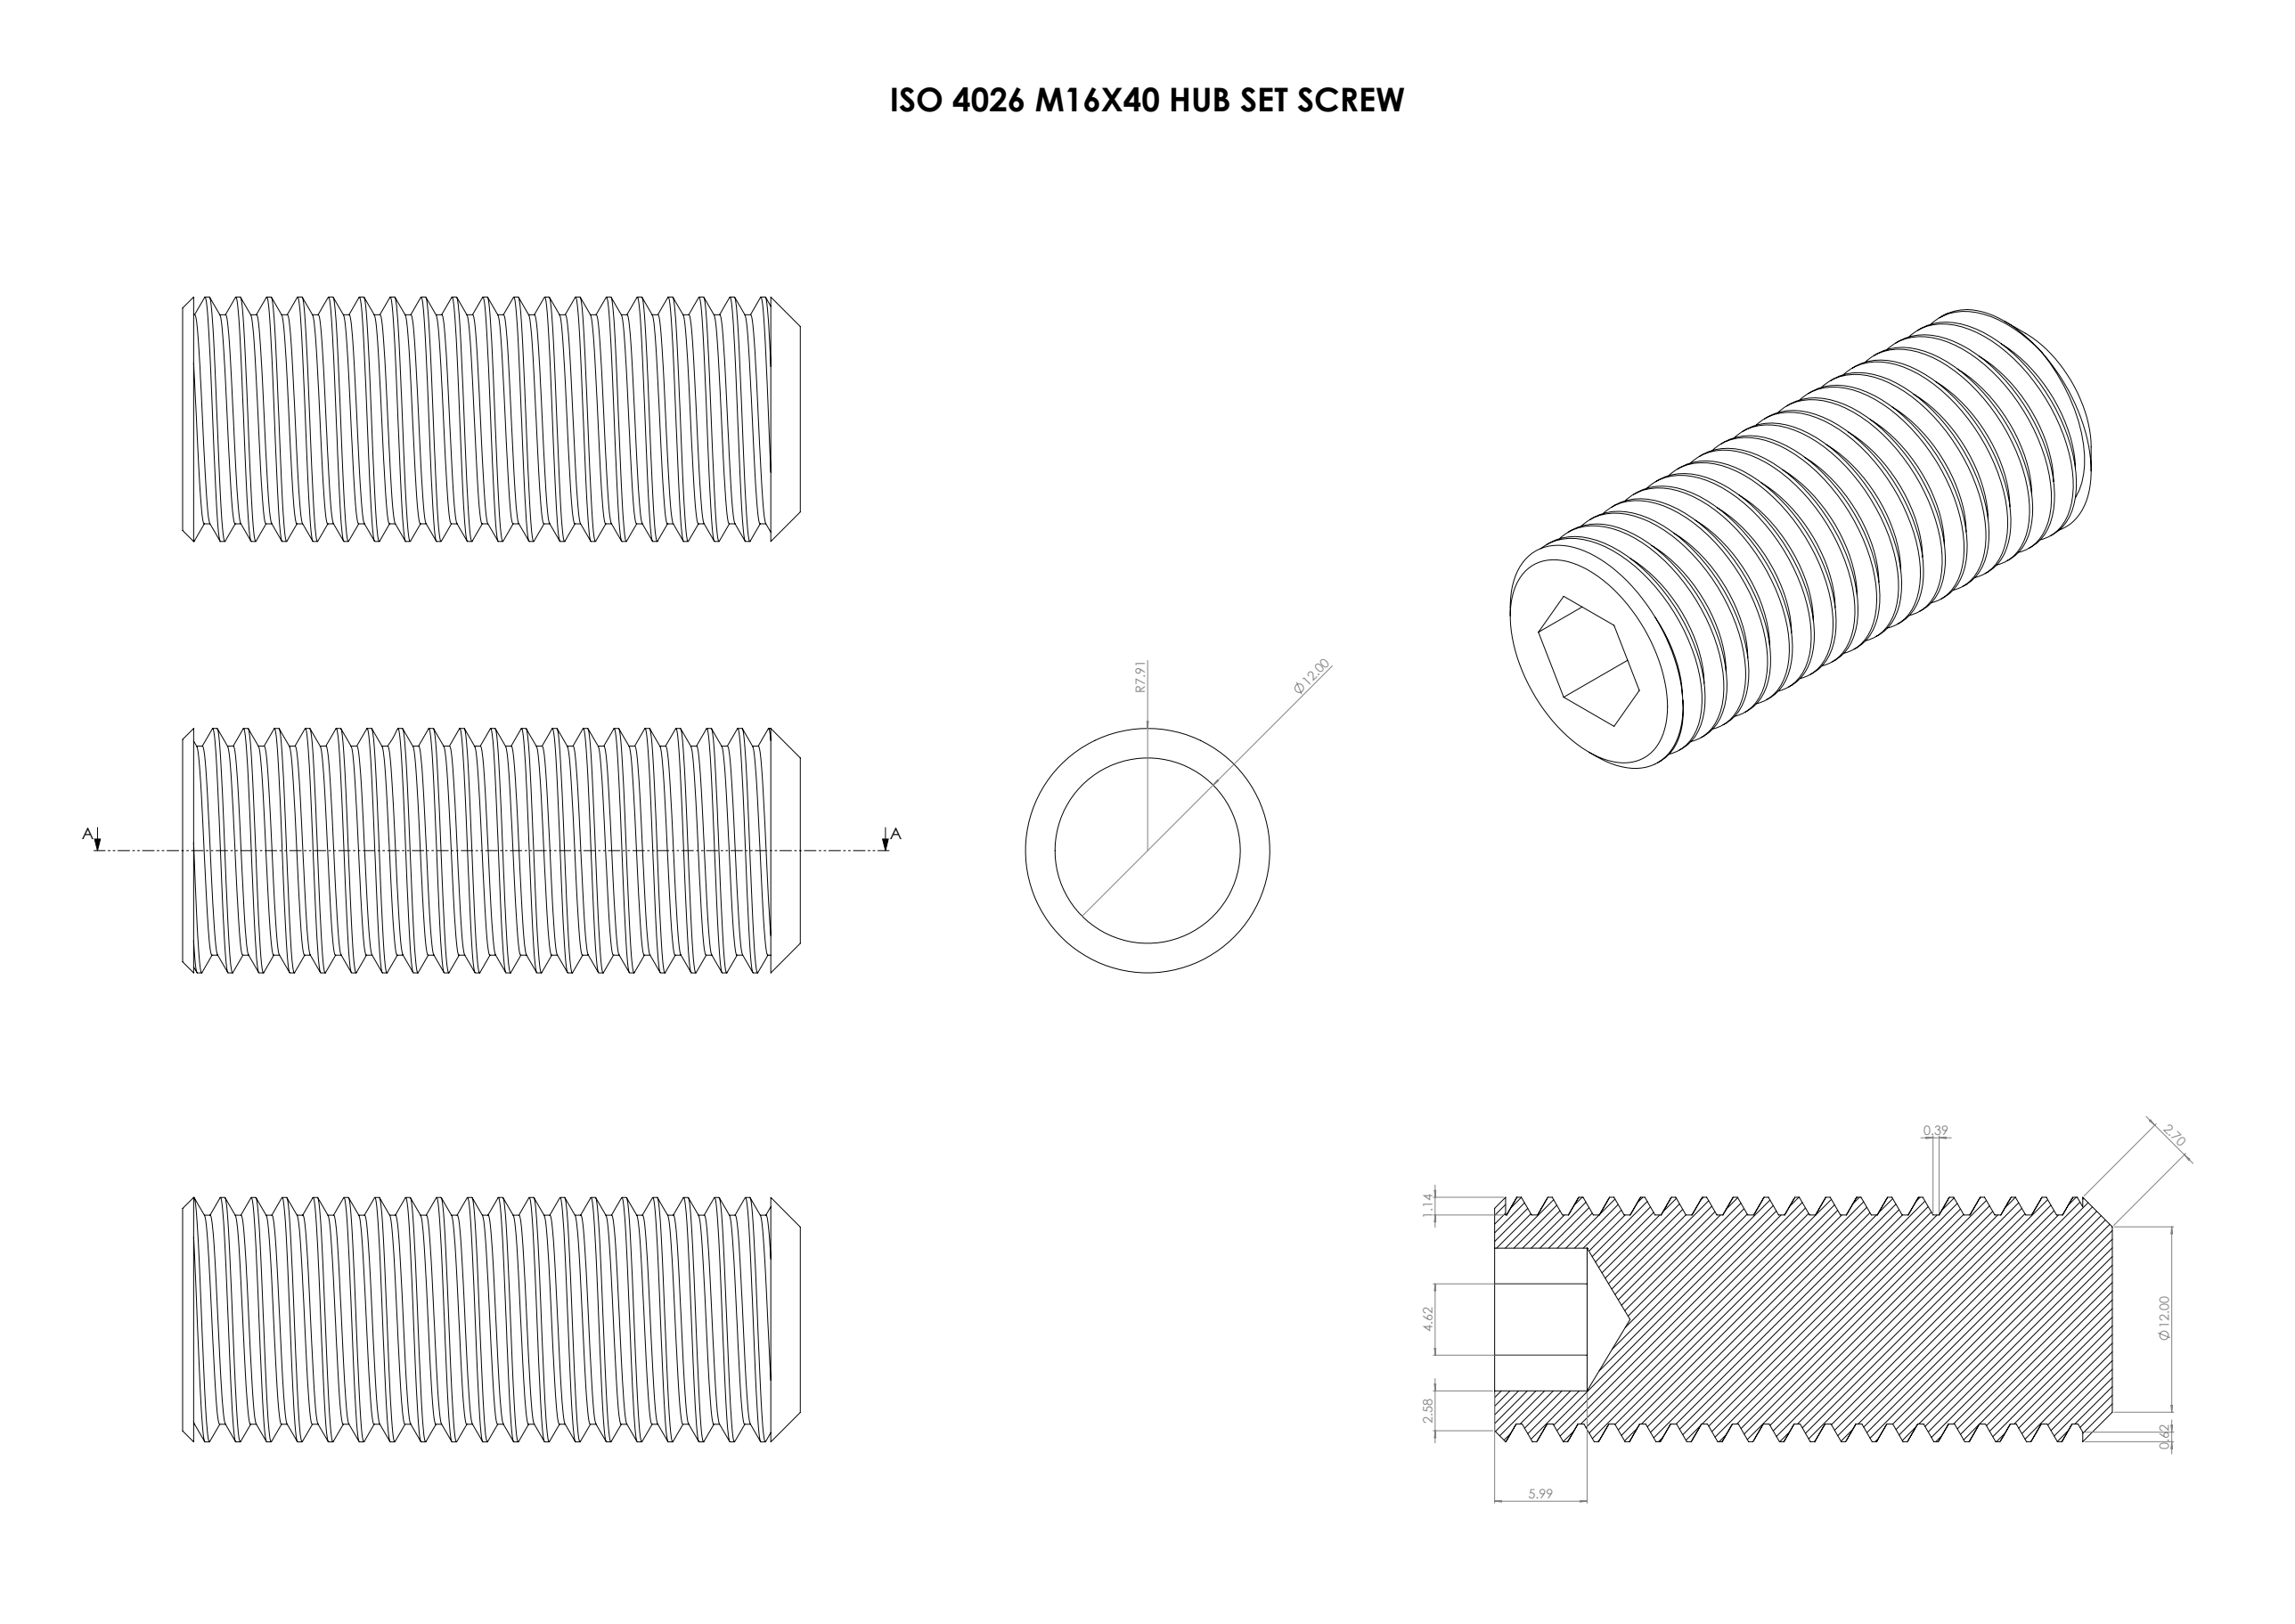
ISO-10303-21;
HEADER;
/* Generated by software containing ST-Developer
 * from STEP Tools, Inc. (www.steptools.com) 
 */

FILE_DESCRIPTION(
/* description */ (''),
/* implementation_level */ '2;1');

FILE_NAME(
/* name */ '14_ISO_4026_M16x40_Hub_Set_Screw.step',
/* time_stamp */ '2026-10-19T23:58:09-07:00',
/* author */ (''),
/* organization */ (''),
/* preprocessor_version */ 'ST-DEVELOPER v20.2',
/* originating_system */ 'Autodesk Translation Framework v15.15.0.0',
/* authorisation */ '');

FILE_SCHEMA (('AP203_CONFIGURATION_CONTROLLED_3D_DESIGN_OF_MECHANICAL_PARTS_AND_ASSEMBLIES_MIM_LF { 1 0 10303 203 3 1 4 }',
'AUTOMOTIVE_DESIGN { 1 0 10303 214 3 1 1 }','INTEGRATED_CNC_SCHEMA','MODEL_BASED_INTEGRATED_MANUFACTURING_SCHEMA',
'PROCESS_PLANNING_SCHEMA','AP242_MANAGED_MODEL_BASED_3D_ENGINEERING_MIM_LF { 1 0 10303 442 3 1 4 }'));
ENDSEC;

DATA;
#10=MECHANICAL_DESIGN_GEOMETRIC_PRESENTATION_REPRESENTATION('',(#416),#70757);
#241=(
BOUNDED_CURVE()
B_SPLINE_CURVE(2,(#59352,#59353,#59354),.UNSPECIFIED.,.F.,.F.)
B_SPLINE_CURVE_WITH_KNOTS((3,3),(0.,0.00348603246849772),.UNSPECIFIED.)
CURVE()
GEOMETRIC_REPRESENTATION_ITEM()
RATIONAL_B_SPLINE_CURVE((1.,1.00000655818292,1.))
REPRESENTATION_ITEM('')
);
#242=(
BOUNDED_CURVE()
B_SPLINE_CURVE(2,(#59356,#59357,#59358),.UNSPECIFIED.,.F.,.F.)
B_SPLINE_CURVE_WITH_KNOTS((3,3),(0.,0.0034860324684977),.UNSPECIFIED.)
CURVE()
GEOMETRIC_REPRESENTATION_ITEM()
RATIONAL_B_SPLINE_CURVE((1.,1.00000655824651,1.))
REPRESENTATION_ITEM('')
);
#243=(
BOUNDED_CURVE()
B_SPLINE_CURVE(2,(#59361,#59362,#59363),.UNSPECIFIED.,.F.,.F.)
B_SPLINE_CURVE_WITH_KNOTS((3,3),(0.,0.00348603246849777),.UNSPECIFIED.)
CURVE()
GEOMETRIC_REPRESENTATION_ITEM()
RATIONAL_B_SPLINE_CURVE((1.,1.00000655828125,1.))
REPRESENTATION_ITEM('')
);
#244=(
BOUNDED_CURVE()
B_SPLINE_CURVE(2,(#59365,#59366,#59367),.UNSPECIFIED.,.F.,.F.)
B_SPLINE_CURVE_WITH_KNOTS((3,3),(0.,0.00348603246849785),.UNSPECIFIED.)
CURVE()
GEOMETRIC_REPRESENTATION_ITEM()
RATIONAL_B_SPLINE_CURVE((1.,1.00000655858972,1.))
REPRESENTATION_ITEM('')
);
#245=(
BOUNDED_CURVE()
B_SPLINE_CURVE(2,(#59370,#59371,#59372),.UNSPECIFIED.,.F.,.F.)
B_SPLINE_CURVE_WITH_KNOTS((3,3),(0.,0.00348603246849743),.UNSPECIFIED.)
CURVE()
GEOMETRIC_REPRESENTATION_ITEM()
RATIONAL_B_SPLINE_CURVE((1.,1.00000655826316,1.))
REPRESENTATION_ITEM('')
);
#246=(
BOUNDED_CURVE()
B_SPLINE_CURVE(2,(#59374,#59375,#59376),.UNSPECIFIED.,.F.,.F.)
B_SPLINE_CURVE_WITH_KNOTS((3,3),(0.,0.00348603246849747),.UNSPECIFIED.)
CURVE()
GEOMETRIC_REPRESENTATION_ITEM()
RATIONAL_B_SPLINE_CURVE((1.,1.00000655837246,1.))
REPRESENTATION_ITEM('')
);
#247=(
BOUNDED_CURVE()
B_SPLINE_CURVE(2,(#59379,#59380,#59381),.UNSPECIFIED.,.F.,.F.)
B_SPLINE_CURVE_WITH_KNOTS((3,3),(0.,0.00348603246849727),.UNSPECIFIED.)
CURVE()
GEOMETRIC_REPRESENTATION_ITEM()
RATIONAL_B_SPLINE_CURVE((1.,1.00000655774933,1.))
REPRESENTATION_ITEM('')
);
#248=(
BOUNDED_CURVE()
B_SPLINE_CURVE(2,(#59383,#59384,#59385),.UNSPECIFIED.,.F.,.F.)
B_SPLINE_CURVE_WITH_KNOTS((3,3),(0.,0.00348603246849747),.UNSPECIFIED.)
CURVE()
GEOMETRIC_REPRESENTATION_ITEM()
RATIONAL_B_SPLINE_CURVE((1.,1.00000655778188,1.))
REPRESENTATION_ITEM('')
);
#249=(
BOUNDED_CURVE()
B_SPLINE_CURVE(2,(#59388,#59389,#59390),.UNSPECIFIED.,.F.,.F.)
B_SPLINE_CURVE_WITH_KNOTS((3,3),(0.,0.00348603246849769),.UNSPECIFIED.)
CURVE()
GEOMETRIC_REPRESENTATION_ITEM()
RATIONAL_B_SPLINE_CURVE((1.,1.00000655825998,1.))
REPRESENTATION_ITEM('')
);
#250=(
BOUNDED_CURVE()
B_SPLINE_CURVE(2,(#59392,#59393,#59394),.UNSPECIFIED.,.F.,.F.)
B_SPLINE_CURVE_WITH_KNOTS((3,3),(0.,0.00348603246849761),.UNSPECIFIED.)
CURVE()
GEOMETRIC_REPRESENTATION_ITEM()
RATIONAL_B_SPLINE_CURVE((1.,1.00000655838487,1.))
REPRESENTATION_ITEM('')
);
#251=(
BOUNDED_CURVE()
B_SPLINE_CURVE(2,(#59397,#59398,#59399),.UNSPECIFIED.,.F.,.F.)
B_SPLINE_CURVE_WITH_KNOTS((3,3),(0.,0.00348603246849764),.UNSPECIFIED.)
CURVE()
GEOMETRIC_REPRESENTATION_ITEM()
RATIONAL_B_SPLINE_CURVE((1.,1.00000655822052,1.))
REPRESENTATION_ITEM('')
);
#252=(
BOUNDED_CURVE()
B_SPLINE_CURVE(2,(#59401,#59402,#59403),.UNSPECIFIED.,.F.,.F.)
B_SPLINE_CURVE_WITH_KNOTS((3,3),(0.,0.00348603246849749),.UNSPECIFIED.)
CURVE()
GEOMETRIC_REPRESENTATION_ITEM()
RATIONAL_B_SPLINE_CURVE((1.,1.00000655832735,1.))
REPRESENTATION_ITEM('')
);
#278=B_SPLINE_SURFACE_WITH_KNOTS('',3,3,((#57157,#57158,#57159,#57160,#57161,
#57162,#57163,#57164,#57165,#57166,#57167,#57168,#57169,#57170,#57171,#57172,
#57173,#57174,#57175,#57176,#57177,#57178,#57179,#57180,#57181,#57182,#57183,
#57184,#57185,#57186,#57187,#57188,#57189,#57190,#57191,#57192,#57193,#57194,
#57195,#57196,#57197,#57198,#57199,#57200,#57201,#57202,#57203,#57204,#57205,
#57206,#57207,#57208,#57209,#57210,#57211,#57212,#57213,#57214,#57215,#57216,
#57217,#57218,#57219,#57220,#57221,#57222,#57223,#57224,#57225,#57226,#57227,
#57228,#57229,#57230,#57231,#57232,#57233,#57234,#57235,#57236,#57237,#57238,
#57239,#57240,#57241,#57242,#57243,#57244,#57245,#57246,#57247,#57248,#57249,
#57250,#57251,#57252,#57253,#57254,#57255,#57256,#57257,#57258,#57259,#57260,
#57261,#57262,#57263,#57264,#57265,#57266,#57267,#57268,#57269,#57270,#57271,
#57272,#57273,#57274,#57275,#57276,#57277,#57278,#57279,#57280,#57281,#57282,
#57283,#57284,#57285,#57286,#57287,#57288,#57289,#57290,#57291,#57292,#57293,
#57294,#57295,#57296,#57297,#57298,#57299,#57300,#57301,#57302,#57303,#57304,
#57305,#57306,#57307,#57308,#57309,#57310,#57311,#57312,#57313,#57314,#57315,
#57316,#57317,#57318,#57319,#57320,#57321,#57322,#57323,#57324,#57325,#57326,
#57327,#57328,#57329,#57330,#57331,#57332,#57333,#57334,#57335,#57336,#57337,
#57338,#57339,#57340,#57341,#57342,#57343,#57344,#57345,#57346,#57347,#57348,
#57349,#57350,#57351,#57352,#57353,#57354,#57355,#57356,#57357,#57358,#57359,
#57360,#57361,#57362,#57363,#57364,#57365,#57366,#57367,#57368,#57369,#57370,
#57371,#57372,#57373,#57374,#57375,#57376,#57377,#57378,#57379,#57380,#57381,
#57382,#57383,#57384,#57385,#57386,#57387,#57388,#57389,#57390,#57391,#57392,
#57393,#57394,#57395,#57396,#57397,#57398,#57399),(#57400,#57401,#57402,
#57403,#57404,#57405,#57406,#57407,#57408,#57409,#57410,#57411,#57412,#57413,
#57414,#57415,#57416,#57417,#57418,#57419,#57420,#57421,#57422,#57423,#57424,
#57425,#57426,#57427,#57428,#57429,#57430,#57431,#57432,#57433,#57434,#57435,
#57436,#57437,#57438,#57439,#57440,#57441,#57442,#57443,#57444,#57445,#57446,
#57447,#57448,#57449,#57450,#57451,#57452,#57453,#57454,#57455,#57456,#57457,
#57458,#57459,#57460,#57461,#57462,#57463,#57464,#57465,#57466,#57467,#57468,
#57469,#57470,#57471,#57472,#57473,#57474,#57475,#57476,#57477,#57478,#57479,
#57480,#57481,#57482,#57483,#57484,#57485,#57486,#57487,#57488,#57489,#57490,
#57491,#57492,#57493,#57494,#57495,#57496,#57497,#57498,#57499,#57500,#57501,
#57502,#57503,#57504,#57505,#57506,#57507,#57508,#57509,#57510,#57511,#57512,
#57513,#57514,#57515,#57516,#57517,#57518,#57519,#57520,#57521,#57522,#57523,
#57524,#57525,#57526,#57527,#57528,#57529,#57530,#57531,#57532,#57533,#57534,
#57535,#57536,#57537,#57538,#57539,#57540,#57541,#57542,#57543,#57544,#57545,
#57546,#57547,#57548,#57549,#57550,#57551,#57552,#57553,#57554,#57555,#57556,
#57557,#57558,#57559,#57560,#57561,#57562,#57563,#57564,#57565,#57566,#57567,
#57568,#57569,#57570,#57571,#57572,#57573,#57574,#57575,#57576,#57577,#57578,
#57579,#57580,#57581,#57582,#57583,#57584,#57585,#57586,#57587,#57588,#57589,
#57590,#57591,#57592,#57593,#57594,#57595,#57596,#57597,#57598,#57599,#57600,
#57601,#57602,#57603,#57604,#57605,#57606,#57607,#57608,#57609,#57610,#57611,
#57612,#57613,#57614,#57615,#57616,#57617,#57618,#57619,#57620,#57621,#57622,
#57623,#57624,#57625,#57626,#57627,#57628,#57629,#57630,#57631,#57632,#57633,
#57634,#57635,#57636,#57637,#57638,#57639,#57640,#57641,#57642),(#57643,
#57644,#57645,#57646,#57647,#57648,#57649,#57650,#57651,#57652,#57653,#57654,
#57655,#57656,#57657,#57658,#57659,#57660,#57661,#57662,#57663,#57664,#57665,
#57666,#57667,#57668,#57669,#57670,#57671,#57672,#57673,#57674,#57675,#57676,
#57677,#57678,#57679,#57680,#57681,#57682,#57683,#57684,#57685,#57686,#57687,
#57688,#57689,#57690,#57691,#57692,#57693,#57694,#57695,#57696,#57697,#57698,
#57699,#57700,#57701,#57702,#57703,#57704,#57705,#57706,#57707,#57708,#57709,
#57710,#57711,#57712,#57713,#57714,#57715,#57716,#57717,#57718,#57719,#57720,
#57721,#57722,#57723,#57724,#57725,#57726,#57727,#57728,#57729,#57730,#57731,
#57732,#57733,#57734,#57735,#57736,#57737,#57738,#57739,#57740,#57741,#57742,
#57743,#57744,#57745,#57746,#57747,#57748,#57749,#57750,#57751,#57752,#57753,
#57754,#57755,#57756,#57757,#57758,#57759,#57760,#57761,#57762,#57763,#57764,
#57765,#57766,#57767,#57768,#57769,#57770,#57771,#57772,#57773,#57774,#57775,
#57776,#57777,#57778,#57779,#57780,#57781,#57782,#57783,#57784,#57785,#57786,
#57787,#57788,#57789,#57790,#57791,#57792,#57793,#57794,#57795,#57796,#57797,
#57798,#57799,#57800,#57801,#57802,#57803,#57804,#57805,#57806,#57807,#57808,
#57809,#57810,#57811,#57812,#57813,#57814,#57815,#57816,#57817,#57818,#57819,
#57820,#57821,#57822,#57823,#57824,#57825,#57826,#57827,#57828,#57829,#57830,
#57831,#57832,#57833,#57834,#57835,#57836,#57837,#57838,#57839,#57840,#57841,
#57842,#57843,#57844,#57845,#57846,#57847,#57848,#57849,#57850,#57851,#57852,
#57853,#57854,#57855,#57856,#57857,#57858,#57859,#57860,#57861,#57862,#57863,
#57864,#57865,#57866,#57867,#57868,#57869,#57870,#57871,#57872,#57873,#57874,
#57875,#57876,#57877,#57878,#57879,#57880,#57881,#57882,#57883,#57884,#57885),
(#57886,#57887,#57888,#57889,#57890,#57891,#57892,#57893,#57894,#57895,
#57896,#57897,#57898,#57899,#57900,#57901,#57902,#57903,#57904,#57905,#57906,
#57907,#57908,#57909,#57910,#57911,#57912,#57913,#57914,#57915,#57916,#57917,
#57918,#57919,#57920,#57921,#57922,#57923,#57924,#57925,#57926,#57927,#57928,
#57929,#57930,#57931,#57932,#57933,#57934,#57935,#57936,#57937,#57938,#57939,
#57940,#57941,#57942,#57943,#57944,#57945,#57946,#57947,#57948,#57949,#57950,
#57951,#57952,#57953,#57954,#57955,#57956,#57957,#57958,#57959,#57960,#57961,
#57962,#57963,#57964,#57965,#57966,#57967,#57968,#57969,#57970,#57971,#57972,
#57973,#57974,#57975,#57976,#57977,#57978,#57979,#57980,#57981,#57982,#57983,
#57984,#57985,#57986,#57987,#57988,#57989,#57990,#57991,#57992,#57993,#57994,
#57995,#57996,#57997,#57998,#57999,#58000,#58001,#58002,#58003,#58004,#58005,
#58006,#58007,#58008,#58009,#58010,#58011,#58012,#58013,#58014,#58015,#58016,
#58017,#58018,#58019,#58020,#58021,#58022,#58023,#58024,#58025,#58026,#58027,
#58028,#58029,#58030,#58031,#58032,#58033,#58034,#58035,#58036,#58037,#58038,
#58039,#58040,#58041,#58042,#58043,#58044,#58045,#58046,#58047,#58048,#58049,
#58050,#58051,#58052,#58053,#58054,#58055,#58056,#58057,#58058,#58059,#58060,
#58061,#58062,#58063,#58064,#58065,#58066,#58067,#58068,#58069,#58070,#58071,
#58072,#58073,#58074,#58075,#58076,#58077,#58078,#58079,#58080,#58081,#58082,
#58083,#58084,#58085,#58086,#58087,#58088,#58089,#58090,#58091,#58092,#58093,
#58094,#58095,#58096,#58097,#58098,#58099,#58100,#58101,#58102,#58103,#58104,
#58105,#58106,#58107,#58108,#58109,#58110,#58111,#58112,#58113,#58114,#58115,
#58116,#58117,#58118,#58119,#58120,#58121,#58122,#58123,#58124,#58125,#58126,
#58127,#58128)),.UNSPECIFIED.,.F.,.F.,.F.,(4,4),(4,1,1,1,1,1,1,1,1,1,1,
1,1,1,1,1,1,1,1,1,1,1,1,1,1,1,1,1,1,1,1,1,1,1,1,1,1,1,1,1,1,1,1,1,1,1,1,
1,1,1,1,1,1,1,1,1,1,1,1,1,1,1,1,1,1,1,1,1,1,1,1,1,1,1,1,1,1,1,1,1,1,1,1,
1,1,1,1,1,1,1,1,1,1,1,1,1,1,1,1,1,1,1,1,1,1,1,1,1,1,1,1,1,1,1,1,1,1,1,1,
1,1,1,1,1,1,1,1,1,1,1,1,1,1,1,1,1,1,1,1,1,1,1,1,1,1,1,1,1,1,1,1,1,1,1,1,
1,1,1,1,1,1,1,1,1,1,1,1,1,1,1,1,1,1,1,1,1,1,1,1,1,1,1,1,1,1,1,1,1,1,1,1,
1,1,1,1,1,1,1,1,1,1,1,1,1,1,1,1,1,1,1,1,1,1,1,1,1,1,1,1,1,1,1,1,1,1,1,1,
1,1,1,1,1,1,1,1,1,1,1,1,1,4),(0.,0.132097741590586),(8.30112925462614,8.79905190745349,
9.29697456028084,9.79489721310818,10.2928198659355,10.7907425187629,11.2886651715902,
11.7865878244176,12.2845104772449,12.7824331300723,13.2803557828996,13.778278435727,
14.2762010885543,14.7741237413817,15.272046394209,15.7699690470363,16.2678916998637,
16.765814352691,17.2637370055184,17.7616596583457,18.2595823111731,18.7575049640004,
19.2554276168278,19.7533502696551,20.2512729224825,20.7491955753098,21.2471182281372,
21.7450408809645,22.2429635337919,22.7408861866192,23.2388088394466,23.7367314922739,
24.2346541451012,24.7325767979286,25.2304994507559,25.7284221035833,26.2263447564106,
26.724267409238,27.2221900620653,27.7201127148927,28.21803536772,28.7159580205474,
29.2138806733747,29.7118033262021,30.2097259790294,30.7076486318568,31.2055712846841,
31.7034939375114,32.2014165903388,32.6993392431661,33.1972618959935,33.6951845488208,
34.1931072016482,34.6910298544755,35.1889525073029,35.6868751601302,36.1847978129576,
36.6827204657849,37.1806431186123,37.6785657714396,38.176488424267,38.6744110770943,
39.1723337299217,39.670256382749,40.1681790355763,40.6661016884037,41.164024341231,
41.6619469940584,42.1598696468857,42.6577922997131,43.1557149525404,43.6536376053678,
44.1515602581951,44.6494829110225,45.1474055638498,45.6453282166772,46.1432508695045,
46.6411735223319,47.1390961751592,47.6370188279866,48.1349414808139,48.6328641336412,
49.1307867864686,49.6287094392959,50.1266320921233,50.6245547449506,51.122477397778,
51.6204000506053,52.1183227034327,52.61624535626,53.1141680090874,53.6120906619147,
54.1100133147421,54.6079359675694,55.1058586203968,55.6037812732241,56.1017039260515,
56.5996265788788,57.0975492317061,57.5954718845335,58.0933945373608,58.5913171901882,
59.0892398430155,59.5871624958429,60.0850851486702,60.5830078014976,61.0809304543249,
61.5788531071523,62.0767757599796,62.574698412807,63.0726210656343,63.5705437184617,
64.068466371289,64.5663890241163,65.0643116769437,65.562234329771,66.0601569825984,
66.5580796354257,67.0560022882531,67.5539249410804,68.0518475939078,68.5497702467351,
69.0476928995625,69.5456155523898,70.0435382052172,70.5414608580445,71.0393835108719,
71.5373061636992,72.0352288165266,72.5331514693539,73.0310741221813,73.5289967750086,
74.0269194278359,74.5248420806633,75.0227647334906,75.520687386318,76.0186100391453,
76.5165326919727,77.0144553448,77.5123779976274,78.0103006504547,78.5082233032821,
79.0061459561094,79.5040686089368,80.0019912617641,80.4999139145914,80.9978365674188,
81.4957592202462,81.9936818730735,82.4916045259008,82.9895271787282,83.4874498315555,
83.9853724843829,84.4832951372102,84.9812177900376,85.4791404428649,85.9770630956923,
86.4749857485196,86.972908401347,87.4708310541743,87.9687537070017,88.466676359829,
88.9645990126564,89.4625216654837,89.960444318311,90.4583669711384,90.9562896239657,
91.4542122767931,91.9521349296204,92.4500575824478,92.9479802352751,93.4459028881025,
93.9438255409298,94.4417481937572,94.9396708465845,95.4375934994119,95.9355161522392,
96.4334388050665,96.9313614578939,97.4292841107213,97.9272067635486,98.4251294163759,
98.9230520692033,99.4209747220306,99.918897374858,100.416820027685,100.914742680513,
101.41266533334,101.910587986167,102.408510638995,102.906433291822,103.404355944649,
103.902278597477,104.400201250304,104.898123903131,105.396046555959,105.893969208786,
106.391891861613,106.889814514441,107.387737167268,107.885659820096,108.383582472923,
108.88150512575,109.379427778578,109.877350431405,110.375273084232,110.87319573706,
111.371118389887,111.869041042714,112.366963695542,112.864886348369,113.362809001196,
113.860731654024,114.358654306851,114.856576959678,115.354499612506,115.852422265333,
116.35034491816,116.848267570988,117.346190223815,117.844112876642,118.34203552947,
118.839958182297,119.337880835125,119.835803487952,120.333726140779,120.831648793607,
121.329571446434,121.827494099261,122.325416752089,122.823339404916,123.321262057743,
123.819184710571,124.317107363398,124.815030016225,125.312952669053,125.81087532188,
126.308797974707,126.806720627535,127.304643280362,127.802565933189),
 .UNSPECIFIED.);
#279=B_SPLINE_SURFACE_WITH_KNOTS('',3,3,((#58334,#58335,#58336,#58337,#58338,
#58339,#58340,#58341,#58342,#58343,#58344,#58345,#58346,#58347,#58348,#58349,
#58350,#58351,#58352,#58353,#58354,#58355,#58356,#58357,#58358,#58359,#58360,
#58361,#58362,#58363,#58364,#58365,#58366,#58367,#58368,#58369,#58370,#58371,
#58372,#58373,#58374,#58375,#58376,#58377,#58378,#58379,#58380,#58381,#58382,
#58383,#58384,#58385,#58386,#58387,#58388,#58389,#58390,#58391,#58392,#58393,
#58394,#58395,#58396,#58397,#58398,#58399,#58400,#58401,#58402,#58403,#58404,
#58405,#58406,#58407,#58408,#58409,#58410,#58411,#58412,#58413,#58414,#58415,
#58416,#58417,#58418,#58419,#58420,#58421,#58422,#58423,#58424,#58425,#58426,
#58427,#58428,#58429,#58430,#58431,#58432,#58433,#58434,#58435,#58436,#58437,
#58438,#58439,#58440,#58441,#58442,#58443,#58444,#58445,#58446,#58447,#58448,
#58449,#58450,#58451,#58452,#58453,#58454,#58455,#58456,#58457,#58458,#58459,
#58460,#58461,#58462,#58463,#58464,#58465,#58466,#58467,#58468,#58469,#58470,
#58471,#58472,#58473,#58474,#58475,#58476,#58477,#58478,#58479,#58480,#58481,
#58482,#58483,#58484,#58485,#58486,#58487,#58488,#58489,#58490,#58491,#58492,
#58493,#58494,#58495,#58496,#58497,#58498,#58499,#58500,#58501,#58502,#58503,
#58504,#58505,#58506,#58507,#58508,#58509,#58510,#58511,#58512,#58513,#58514,
#58515,#58516,#58517,#58518,#58519,#58520,#58521,#58522,#58523,#58524,#58525,
#58526,#58527,#58528,#58529,#58530,#58531,#58532,#58533,#58534,#58535,#58536,
#58537,#58538,#58539,#58540,#58541,#58542,#58543,#58544,#58545,#58546,#58547,
#58548,#58549,#58550,#58551,#58552,#58553,#58554,#58555,#58556,#58557,#58558,
#58559,#58560,#58561,#58562,#58563,#58564,#58565,#58566,#58567,#58568,#58569,
#58570,#58571,#58572,#58573,#58574,#58575,#58576),(#58577,#58578,#58579,
#58580,#58581,#58582,#58583,#58584,#58585,#58586,#58587,#58588,#58589,#58590,
#58591,#58592,#58593,#58594,#58595,#58596,#58597,#58598,#58599,#58600,#58601,
#58602,#58603,#58604,#58605,#58606,#58607,#58608,#58609,#58610,#58611,#58612,
#58613,#58614,#58615,#58616,#58617,#58618,#58619,#58620,#58621,#58622,#58623,
#58624,#58625,#58626,#58627,#58628,#58629,#58630,#58631,#58632,#58633,#58634,
#58635,#58636,#58637,#58638,#58639,#58640,#58641,#58642,#58643,#58644,#58645,
#58646,#58647,#58648,#58649,#58650,#58651,#58652,#58653,#58654,#58655,#58656,
#58657,#58658,#58659,#58660,#58661,#58662,#58663,#58664,#58665,#58666,#58667,
#58668,#58669,#58670,#58671,#58672,#58673,#58674,#58675,#58676,#58677,#58678,
#58679,#58680,#58681,#58682,#58683,#58684,#58685,#58686,#58687,#58688,#58689,
#58690,#58691,#58692,#58693,#58694,#58695,#58696,#58697,#58698,#58699,#58700,
#58701,#58702,#58703,#58704,#58705,#58706,#58707,#58708,#58709,#58710,#58711,
#58712,#58713,#58714,#58715,#58716,#58717,#58718,#58719,#58720,#58721,#58722,
#58723,#58724,#58725,#58726,#58727,#58728,#58729,#58730,#58731,#58732,#58733,
#58734,#58735,#58736,#58737,#58738,#58739,#58740,#58741,#58742,#58743,#58744,
#58745,#58746,#58747,#58748,#58749,#58750,#58751,#58752,#58753,#58754,#58755,
#58756,#58757,#58758,#58759,#58760,#58761,#58762,#58763,#58764,#58765,#58766,
#58767,#58768,#58769,#58770,#58771,#58772,#58773,#58774,#58775,#58776,#58777,
#58778,#58779,#58780,#58781,#58782,#58783,#58784,#58785,#58786,#58787,#58788,
#58789,#58790,#58791,#58792,#58793,#58794,#58795,#58796,#58797,#58798,#58799,
#58800,#58801,#58802,#58803,#58804,#58805,#58806,#58807,#58808,#58809,#58810,
#58811,#58812,#58813,#58814,#58815,#58816,#58817,#58818,#58819),(#58820,
#58821,#58822,#58823,#58824,#58825,#58826,#58827,#58828,#58829,#58830,#58831,
#58832,#58833,#58834,#58835,#58836,#58837,#58838,#58839,#58840,#58841,#58842,
#58843,#58844,#58845,#58846,#58847,#58848,#58849,#58850,#58851,#58852,#58853,
#58854,#58855,#58856,#58857,#58858,#58859,#58860,#58861,#58862,#58863,#58864,
#58865,#58866,#58867,#58868,#58869,#58870,#58871,#58872,#58873,#58874,#58875,
#58876,#58877,#58878,#58879,#58880,#58881,#58882,#58883,#58884,#58885,#58886,
#58887,#58888,#58889,#58890,#58891,#58892,#58893,#58894,#58895,#58896,#58897,
#58898,#58899,#58900,#58901,#58902,#58903,#58904,#58905,#58906,#58907,#58908,
#58909,#58910,#58911,#58912,#58913,#58914,#58915,#58916,#58917,#58918,#58919,
#58920,#58921,#58922,#58923,#58924,#58925,#58926,#58927,#58928,#58929,#58930,
#58931,#58932,#58933,#58934,#58935,#58936,#58937,#58938,#58939,#58940,#58941,
#58942,#58943,#58944,#58945,#58946,#58947,#58948,#58949,#58950,#58951,#58952,
#58953,#58954,#58955,#58956,#58957,#58958,#58959,#58960,#58961,#58962,#58963,
#58964,#58965,#58966,#58967,#58968,#58969,#58970,#58971,#58972,#58973,#58974,
#58975,#58976,#58977,#58978,#58979,#58980,#58981,#58982,#58983,#58984,#58985,
#58986,#58987,#58988,#58989,#58990,#58991,#58992,#58993,#58994,#58995,#58996,
#58997,#58998,#58999,#59000,#59001,#59002,#59003,#59004,#59005,#59006,#59007,
#59008,#59009,#59010,#59011,#59012,#59013,#59014,#59015,#59016,#59017,#59018,
#59019,#59020,#59021,#59022,#59023,#59024,#59025,#59026,#59027,#59028,#59029,
#59030,#59031,#59032,#59033,#59034,#59035,#59036,#59037,#59038,#59039,#59040,
#59041,#59042,#59043,#59044,#59045,#59046,#59047,#59048,#59049,#59050,#59051,
#59052,#59053,#59054,#59055,#59056,#59057,#59058,#59059,#59060,#59061,#59062),
(#59063,#59064,#59065,#59066,#59067,#59068,#59069,#59070,#59071,#59072,
#59073,#59074,#59075,#59076,#59077,#59078,#59079,#59080,#59081,#59082,#59083,
#59084,#59085,#59086,#59087,#59088,#59089,#59090,#59091,#59092,#59093,#59094,
#59095,#59096,#59097,#59098,#59099,#59100,#59101,#59102,#59103,#59104,#59105,
#59106,#59107,#59108,#59109,#59110,#59111,#59112,#59113,#59114,#59115,#59116,
#59117,#59118,#59119,#59120,#59121,#59122,#59123,#59124,#59125,#59126,#59127,
#59128,#59129,#59130,#59131,#59132,#59133,#59134,#59135,#59136,#59137,#59138,
#59139,#59140,#59141,#59142,#59143,#59144,#59145,#59146,#59147,#59148,#59149,
#59150,#59151,#59152,#59153,#59154,#59155,#59156,#59157,#59158,#59159,#59160,
#59161,#59162,#59163,#59164,#59165,#59166,#59167,#59168,#59169,#59170,#59171,
#59172,#59173,#59174,#59175,#59176,#59177,#59178,#59179,#59180,#59181,#59182,
#59183,#59184,#59185,#59186,#59187,#59188,#59189,#59190,#59191,#59192,#59193,
#59194,#59195,#59196,#59197,#59198,#59199,#59200,#59201,#59202,#59203,#59204,
#59205,#59206,#59207,#59208,#59209,#59210,#59211,#59212,#59213,#59214,#59215,
#59216,#59217,#59218,#59219,#59220,#59221,#59222,#59223,#59224,#59225,#59226,
#59227,#59228,#59229,#59230,#59231,#59232,#59233,#59234,#59235,#59236,#59237,
#59238,#59239,#59240,#59241,#59242,#59243,#59244,#59245,#59246,#59247,#59248,
#59249,#59250,#59251,#59252,#59253,#59254,#59255,#59256,#59257,#59258,#59259,
#59260,#59261,#59262,#59263,#59264,#59265,#59266,#59267,#59268,#59269,#59270,
#59271,#59272,#59273,#59274,#59275,#59276,#59277,#59278,#59279,#59280,#59281,
#59282,#59283,#59284,#59285,#59286,#59287,#59288,#59289,#59290,#59291,#59292,
#59293,#59294,#59295,#59296,#59297,#59298,#59299,#59300,#59301,#59302,#59303,
#59304,#59305)),.UNSPECIFIED.,.F.,.F.,.F.,(4,4),(4,1,1,1,1,1,1,1,1,1,1,
1,1,1,1,1,1,1,1,1,1,1,1,1,1,1,1,1,1,1,1,1,1,1,1,1,1,1,1,1,1,1,1,1,1,1,1,
1,1,1,1,1,1,1,1,1,1,1,1,1,1,1,1,1,1,1,1,1,1,1,1,1,1,1,1,1,1,1,1,1,1,1,1,
1,1,1,1,1,1,1,1,1,1,1,1,1,1,1,1,1,1,1,1,1,1,1,1,1,1,1,1,1,1,1,1,1,1,1,1,
1,1,1,1,1,1,1,1,1,1,1,1,1,1,1,1,1,1,1,1,1,1,1,1,1,1,1,1,1,1,1,1,1,1,1,1,
1,1,1,1,1,1,1,1,1,1,1,1,1,1,1,1,1,1,1,1,1,1,1,1,1,1,1,1,1,1,1,1,1,1,1,1,
1,1,1,1,1,1,1,1,1,1,1,1,1,1,1,1,1,1,1,1,1,1,1,1,1,1,1,1,1,1,1,1,1,1,1,1,
1,1,1,1,1,1,1,1,1,1,1,1,1,4),(0.,0.132097741590586),(11.6150328478182,12.1129555006455,
12.6108781534729,13.1088008063002,13.6067234591276,14.1046461119549,14.6025687647823,
15.1004914176096,15.5984140704369,16.0963367232643,16.5942593760916,17.092182028919,
17.5901046817463,18.0880273345737,18.585949987401,19.0838726402284,19.5817952930557,
20.0797179458831,20.5776405987104,21.0755632515378,21.5734859043651,22.0714085571925,
22.5693312100198,23.0672538628472,23.5651765156745,24.0630991685018,24.5610218213292,
25.0589444741565,25.5568671269839,26.0547897798112,26.5527124326386,27.0506350854659,
27.5485577382933,28.0464803911206,28.544403043948,29.0423256967753,29.5402483496027,
30.03817100243,30.5360936552574,31.0340163080847,31.5319389609121,32.0298616137394,
32.5277842665667,33.0257069193941,33.5236295722214,34.0215522250488,34.5194748778761,
35.0173975307035,35.5153201835308,36.0132428363582,36.5111654891855,37.0090881420129,
37.5070107948402,38.0049334476676,38.5028561004949,39.0007787533223,39.4987014061496,
39.9966240589769,40.4945467118043,40.9924693646316,41.490392017459,41.9883146702863,
42.4862373231137,42.984159975941,43.4820826287684,43.9800052815957,44.4779279344231,
44.9758505872504,45.4737732400778,45.9716958929051,46.4696185457325,46.9675411985598,
47.4654638513871,47.9633865042145,48.4613091570418,48.9592318098692,49.4571544626965,
49.9550771155239,50.4529997683512,50.9509224211786,51.4488450740059,51.9467677268333,
52.4446903796606,52.942613032488,53.4405356853153,53.9384583381427,54.43638099097,
54.9343036437973,55.4322262966247,55.930148949452,56.4280716022794,56.9259942551067,
57.4239169079341,57.9218395607614,58.4197622135888,58.9176848664161,59.4156075192435,
59.9135301720708,60.4114528248982,60.9093754777255,61.4072981305529,61.9052207833802,
62.4031434362076,62.9010660890349,63.3989887418622,63.8969113946896,64.3948340475169,
64.8927567003443,65.3906793531716,65.888602005999,66.3865246588263,66.8844473116537,
67.382369964481,67.8802926173084,68.3782152701357,68.8761379229631,69.3740605757904,
69.8719832286178,70.3699058814451,70.8678285342725,71.3657511870998,71.8636738399271,
72.3615964927545,72.8595191455818,73.3574417984092,73.8553644512365,74.3532871040639,
74.8512097568912,75.3491324097186,75.8470550625459,76.3449777153733,76.8429003682006,
77.340823021028,77.8387456738553,78.3366683266827,78.83459097951,79.3325136323374,
79.8304362851647,80.328358937992,80.8262815908194,81.3242042436467,81.8221268964741,
82.3200495493014,82.8179722021288,83.3158948549561,83.8138175077835,84.3117401606108,
84.8096628134382,85.3075854662655,85.8055081190928,86.3034307719202,86.8013534247476,
87.2992760775749,87.7971987304022,88.2951213832296,88.7930440360569,89.2909666888843,
89.7888893417116,90.286811994539,90.7847346473663,91.2826573001937,91.780579953021,
92.2785026058484,92.7764252586757,93.2743479115031,93.7722705643304,94.2701932171578,
94.7681158699851,95.2660385228125,95.7639611756398,96.2618838284671,96.7598064812945,
97.2577291341218,97.7556517869492,98.2535744397765,98.7514970926039,99.2494197454312,
99.7473423982586,100.245265051086,100.743187703913,101.241110356741,101.739033009568,
102.236955662395,102.734878315223,103.23280096805,103.730723620877,104.228646273705,
104.726568926532,105.224491579359,105.722414232187,106.220336885014,106.718259537841,
107.216182190669,107.714104843496,108.212027496323,108.709950149151,109.207872801978,
109.705795454805,110.203718107633,110.70164076046,111.199563413288,111.697486066115,
112.195408718942,112.69333137177,113.191254024597,113.689176677424,114.187099330252,
114.685021983079,115.182944635906,115.680867288734,116.178789941561,116.676712594388,
117.174635247216,117.672557900043,118.17048055287,118.668403205698,119.166325858525,
119.664248511352,120.16217116418,120.660093817007,121.158016469834,121.655939122662,
122.153861775489,122.651784428317,123.149707081144,123.647629733971,124.145552386799,
124.643475039626,125.141397692453,125.639320345281,126.137242998108,126.635165650935,
127.133088303763,127.63101095659,128.128933609417,128.626856262245,129.124778915072,
129.622701567899,130.120624220727,130.618546873554,131.116469526381),
 .UNSPECIFIED.);
#386=SHAPE_REPRESENTATION_RELATIONSHIP('SRR','None',#70827,#401);
#401=ADVANCED_BREP_SHAPE_REPRESENTATION('',(#476),#70751);
#416=STYLED_ITEM('',(#71054),#476);
#476=MANIFOLD_SOLID_BREP('Set screw',#26881);
#683=CYLINDRICAL_SURFACE('',#27690,0.7911);
#684=CYLINDRICAL_SURFACE('',#27692,0.7911);
#685=CYLINDRICAL_SURFACE('',#27693,0.7911);
#686=CYLINDRICAL_SURFACE('',#27694,0.7911);
#687=CYLINDRICAL_SURFACE('',#27695,0.7911);
#688=CYLINDRICAL_SURFACE('',#27696,0.7911);
#689=CYLINDRICAL_SURFACE('',#27697,0.7911);
#690=CYLINDRICAL_SURFACE('',#27698,0.7911);
#691=CYLINDRICAL_SURFACE('',#27699,0.7911);
#692=CYLINDRICAL_SURFACE('',#27700,0.7911);
#693=CYLINDRICAL_SURFACE('',#27701,0.7911);
#694=CYLINDRICAL_SURFACE('',#27702,0.7911);
#695=CYLINDRICAL_SURFACE('',#27703,0.7911);
#696=CYLINDRICAL_SURFACE('',#27704,0.7911);
#697=CYLINDRICAL_SURFACE('',#27705,0.7911);
#698=CYLINDRICAL_SURFACE('',#27706,0.7911);
#699=CYLINDRICAL_SURFACE('',#27707,0.7911);
#700=CYLINDRICAL_SURFACE('',#27708,0.7911);
#701=CYLINDRICAL_SURFACE('',#27709,0.7911);
#702=CYLINDRICAL_SURFACE('',#27710,0.6767);
#703=CYLINDRICAL_SURFACE('',#27712,0.6767);
#704=CYLINDRICAL_SURFACE('',#27714,0.6767);
#705=CYLINDRICAL_SURFACE('',#27715,0.6767);
#706=CYLINDRICAL_SURFACE('',#27716,0.6767);
#707=CYLINDRICAL_SURFACE('',#27717,0.6767);
#708=CYLINDRICAL_SURFACE('',#27718,0.6767);
#709=CYLINDRICAL_SURFACE('',#27719,0.6767);
#710=CYLINDRICAL_SURFACE('',#27720,0.6767);
#711=CYLINDRICAL_SURFACE('',#27721,0.6767);
#712=CYLINDRICAL_SURFACE('',#27722,0.6767);
#713=CYLINDRICAL_SURFACE('',#27723,0.6767);
#714=CYLINDRICAL_SURFACE('',#27724,0.6767);
#715=CYLINDRICAL_SURFACE('',#27725,0.6767);
#716=CYLINDRICAL_SURFACE('',#27726,0.6767);
#717=CYLINDRICAL_SURFACE('',#27727,0.6767);
#718=CYLINDRICAL_SURFACE('',#27728,0.6767);
#719=CYLINDRICAL_SURFACE('',#27729,0.6767);
#720=CYLINDRICAL_SURFACE('',#27730,0.6767);
#721=CYLINDRICAL_SURFACE('',#27738,0.6767);
#722=CYLINDRICAL_SURFACE('',#27786,0.7911);
#867=FACE_BOUND('',#4614,.T.);
#1293=B_SPLINE_CURVE_WITH_KNOTS('',3,(#54716,#54717,#54718,#54719,#54720,
#54721,#54722,#54723,#54724,#54725,#54726,#54727,#54728,#54729,#54730,#54731),
 .UNSPECIFIED.,.F.,.F.,(4,3,3,3,3,4),(-4.09293042013069,-3.98338122261878,
-3.48545856979143,-2.98753591696408,-2.48961326413674,-2.07498647268396),
 .UNSPECIFIED.);
#1294=B_SPLINE_CURVE_WITH_KNOTS('',3,(#54734,#54735,#54736,#54737,#54738,
#54739,#54740,#54741,#54742,#54743),.UNSPECIFIED.,.F.,.F.,(4,3,3,4),(0.,
0.497922652827334,0.99584530565469,1.12364870614302),.UNSPECIFIED.);
#1295=B_SPLINE_CURVE_WITH_KNOTS('',3,(#54748,#54749,#54750,#54751,#54752,
#54753,#54754,#54755,#54756,#54757,#54758,#54759,#54760,#54761,#54762,#54763,
#54764,#54765,#54766,#54767,#54768,#54769,#54770,#54771,#54772,#54773,#54774,
#54775,#54776,#54777,#54778,#54779,#54780,#54781,#54782,#54783,#54784,#54785,
#54786,#54787),.UNSPECIFIED.,.F.,.F.,(4,3,3,3,3,3,3,3,3,3,3,3,3,4),(-10.3761157273103,
-9.95845305654694,-9.46053040371959,-8.96260775089224,-8.4646850980649,
-7.96676244523755,-7.46883979241021,-6.97091713958286,-6.47299448675551,
-5.97507183392816,-5.47714918110082,-4.97922652827347,-4.48130387544612,
-4.09293042013069),.UNSPECIFIED.);
#1296=B_SPLINE_CURVE_WITH_KNOTS('',3,(#54788,#54789,#54790,#54791,#54792,
#54793,#54794,#54795,#54796,#54797,#54798,#54799,#54800,#54801,#54802,#54803,
#54804,#54805,#54806,#54807,#54808,#54809,#54810,#54811,#54812,#54813,#54814,
#54815,#54816,#54817,#54818,#54819,#54820,#54821,#54822,#54823,#54824,#54825,
#54826,#54827),.UNSPECIFIED.,.F.,.F.,(4,3,3,3,3,3,3,3,3,3,3,3,3,4),(1.12364870614302,
1.49376795848204,1.99169061130939,2.48961326413673,2.98753591696408,3.48545856979143,
3.98338122261877,4.48130387544612,4.97922652827347,5.47714918110082,5.97507183392816,
6.47299448675551,6.97091713958286,7.40683401332261),.UNSPECIFIED.);
#1297=B_SPLINE_CURVE_WITH_KNOTS('',3,(#54832,#54833,#54834,#54835,#54836,
#54837,#54838,#54839,#54840,#54841,#54842,#54843,#54844,#54845,#54846,#54847,
#54848,#54849,#54850,#54851,#54852,#54853,#54854,#54855,#54856,#54857,#54858,
#54859,#54860,#54861,#54862,#54863,#54864,#54865,#54866,#54867,#54868,#54869,
#54870,#54871,#54872,#54873,#54874),.UNSPECIFIED.,.F.,.F.,(4,3,3,3,3,3,
3,3,3,3,3,3,3,3,4),(-16.6593010344899,-16.4314475433024,-15.9335248904751,
-15.4356022376478,-14.9376795848204,-14.4397569319931,-13.9418342791657,
-13.4439116263384,-12.945988973511,-12.4480663206837,-11.9501436678563,
-11.452221015029,-10.9542983622016,-10.4563757093743,-10.3761157273103),
 .UNSPECIFIED.);
#1298=B_SPLINE_CURVE_WITH_KNOTS('',3,(#54875,#54876,#54877,#54878,#54879,
#54880,#54881,#54882,#54883,#54884,#54885,#54886,#54887,#54888,#54889,#54890,
#54891,#54892,#54893,#54894,#54895,#54896,#54897,#54898,#54899,#54900,#54901,
#54902,#54903,#54904,#54905,#54906,#54907,#54908,#54909,#54910,#54911,#54912,
#54913,#54914,#54915,#54916,#54917),.UNSPECIFIED.,.F.,.F.,(4,3,3,3,3,3,
3,3,3,3,3,3,3,3,4),(7.40683401332261,7.4688397924102,7.96676244523755,8.4646850980649,
8.96260775089224,9.46053040371959,9.95845305654694,10.4563757093743,10.9542983622016,
11.452221015029,11.9501436678563,12.4480663206837,12.945988973511,13.4439116263384,
13.6900193205022),.UNSPECIFIED.);
#1299=B_SPLINE_CURVE_WITH_KNOTS('',3,(#54922,#54923,#54924,#54925,#54926,
#54927,#54928,#54929,#54930,#54931,#54932,#54933,#54934,#54935,#54936,#54937,
#54938,#54939,#54940,#54941,#54942,#54943,#54944,#54945,#54946,#54947,#54948,
#54949,#54950,#54951,#54952,#54953,#54954,#54955,#54956,#54957,#54958,#54959,
#54960,#54961,#54962,#54963,#54964),.UNSPECIFIED.,.F.,.F.,(4,3,3,3,3,3,
3,3,3,3,3,3,3,3,4),(-22.9424863416694,-22.904442030058,-22.4065193772306,
-21.9085967244033,-21.4106740715759,-20.9127514187486,-20.4148287659212,
-19.9169061130939,-19.4189834602665,-18.9210608074392,-18.4231381546118,
-17.9252155017845,-17.4272928489571,-16.9293701961298,-16.6593010344899),
 .UNSPECIFIED.);
#1300=B_SPLINE_CURVE_WITH_KNOTS('',3,(#54965,#54966,#54967,#54968,#54969,
#54970,#54971,#54972,#54973,#54974,#54975,#54976,#54977,#54978,#54979,#54980,
#54981,#54982,#54983,#54984,#54985,#54986,#54987,#54988,#54989,#54990,#54991,
#54992,#54993,#54994,#54995,#54996,#54997,#54998,#54999,#55000,#55001,#55002,
#55003,#55004,#55005,#55006,#55007),.UNSPECIFIED.,.F.,.F.,(4,3,3,3,3,3,
3,3,3,3,3,3,3,3,4),(13.6900193205022,13.9418342791657,14.4397569319931,
14.9376795848204,15.4356022376478,15.9335248904751,16.4314475433025,16.9293701961298,
17.4272928489571,17.9252155017845,18.4231381546118,18.9210608074392,19.4189834602665,
19.9169061130939,19.9732046276818),.UNSPECIFIED.);
#1301=B_SPLINE_CURVE_WITH_KNOTS('',3,(#55012,#55013,#55014,#55015,#55016,
#55017,#55018,#55019,#55020,#55021,#55022,#55023,#55024,#55025,#55026,#55027,
#55028,#55029,#55030,#55031,#55032,#55033,#55034,#55035,#55036,#55037,#55038,
#55039,#55040,#55041,#55042,#55043,#55044,#55045,#55046,#55047,#55048,#55049,
#55050,#55051),.UNSPECIFIED.,.F.,.F.,(4,3,3,3,3,3,3,3,3,3,3,3,3,4),(-29.225671648849,
-28.8795138639861,-28.3815912111588,-27.8836685583314,-27.3857459055041,
-26.8878232526767,-26.3899005998494,-25.891977947022,-25.3940552941947,
-24.8961326413673,-24.39820998854,-23.9002873357127,-23.4023646828853,-22.9424863416694),
 .UNSPECIFIED.);
#1302=B_SPLINE_CURVE_WITH_KNOTS('',3,(#55052,#55053,#55054,#55055,#55056,
#55057,#55058,#55059,#55060,#55061,#55062,#55063,#55064,#55065,#55066,#55067,
#55068,#55069,#55070,#55071,#55072,#55073,#55074,#55075,#55076,#55077,#55078,
#55079,#55080,#55081,#55082,#55083,#55084,#55085,#55086,#55087,#55088,#55089,
#55090,#55091),.UNSPECIFIED.,.F.,.F.,(4,3,3,3,3,3,3,3,3,3,3,3,3,4),(19.9732046276818,
20.4148287659212,20.9127514187486,21.4106740715759,21.9085967244033,22.4065193772306,
22.904442030058,23.4023646828853,23.9002873357127,24.39820998854,24.8961326413673,
25.3940552941947,25.891977947022,26.2563899348614),.UNSPECIFIED.);
#1303=B_SPLINE_CURVE_WITH_KNOTS('',3,(#55096,#55097,#55098,#55099,#55100,
#55101,#55102,#55103,#55104,#55105,#55106,#55107,#55108,#55109,#55110,#55111,
#55112,#55113,#55114,#55115,#55116,#55117,#55118,#55119,#55120,#55121,#55122,
#55123,#55124,#55125,#55126,#55127,#55128,#55129,#55130,#55131,#55132,#55133,
#55134,#55135,#55136,#55137,#55138),.UNSPECIFIED.,.F.,.F.,(4,3,3,3,3,3,
3,3,3,3,3,3,3,3,4),(-35.5088569560286,-35.3525083507416,-34.8545856979143,
-34.3566630450869,-33.8587403922596,-33.3608177394322,-32.8628950866049,
-32.3649724337776,-31.8670497809502,-31.3691271281229,-30.8712044752955,
-30.3732818224682,-29.8753591696408,-29.3774365168135,-29.225671648849),
 .UNSPECIFIED.);
#1304=B_SPLINE_CURVE_WITH_KNOTS('',3,(#55139,#55140,#55141,#55142,#55143,
#55144,#55145,#55146,#55147,#55148,#55149,#55150,#55151,#55152,#55153,#55154,
#55155,#55156,#55157,#55158,#55159,#55160,#55161,#55162,#55163,#55164,#55165,
#55166,#55167,#55168,#55169,#55170,#55171,#55172,#55173,#55174,#55175,#55176,
#55177,#55178,#55179,#55180,#55181),.UNSPECIFIED.,.F.,.F.,(4,3,3,3,3,3,
3,3,3,3,3,3,3,3,4),(26.2563899348614,26.3899005998494,26.8878232526767,
27.3857459055041,27.8836685583314,28.3815912111588,28.8795138639861,29.3774365168135,
29.8753591696408,30.3732818224682,30.8712044752955,31.3691271281229,31.8670497809502,
32.3649724337775,32.5395752420409),.UNSPECIFIED.);
#1305=B_SPLINE_CURVE_WITH_KNOTS('',3,(#55186,#55187,#55188,#55189,#55190,
#55191,#55192,#55193,#55194,#55195,#55196,#55197,#55198,#55199,#55200,#55201,
#55202,#55203,#55204,#55205,#55206,#55207,#55208,#55209,#55210,#55211,#55212,
#55213,#55214,#55215,#55216,#55217,#55218,#55219,#55220,#55221,#55222,#55223,
#55224,#55225),.UNSPECIFIED.,.F.,.F.,(4,3,3,3,3,3,3,3,3,3,3,3,3,4),(-41.7920422632082,
-41.3275801846698,-40.8296575318424,-40.3317348790151,-39.8338122261878,
-39.3358895733604,-38.8379669205331,-38.3400442677057,-37.8421216148784,
-37.344198962051,-36.8462763092237,-36.3483536563963,-35.850431003569,-35.5088569560286),
 .UNSPECIFIED.);
#1306=B_SPLINE_CURVE_WITH_KNOTS('',3,(#55226,#55227,#55228,#55229,#55230,
#55231,#55232,#55233,#55234,#55235,#55236,#55237,#55238,#55239,#55240,#55241,
#55242,#55243,#55244,#55245,#55246,#55247,#55248,#55249,#55250,#55251,#55252,
#55253,#55254,#55255,#55256,#55257,#55258,#55259,#55260,#55261,#55262,#55263,
#55264,#55265),.UNSPECIFIED.,.F.,.F.,(4,3,3,3,3,3,3,3,3,3,3,3,3,4),(32.5395752420409,
32.8628950866049,33.3608177394322,33.8587403922596,34.3566630450869,34.8545856979143,
35.3525083507416,35.850431003569,36.3483536563963,36.8462763092237,37.344198962051,
37.8421216148784,38.3400442677057,38.8227605492205),.UNSPECIFIED.);
#1307=B_SPLINE_CURVE_WITH_KNOTS('',3,(#55270,#55271,#55272,#55273,#55274,
#55275,#55276,#55277,#55278,#55279,#55280,#55281,#55282,#55283,#55284,#55285,
#55286,#55287,#55288,#55289,#55290,#55291,#55292,#55293,#55294,#55295,#55296,
#55297,#55298,#55299,#55300,#55301,#55302,#55303,#55304,#55305,#55306,#55307,
#55308,#55309,#55310,#55311,#55312),.UNSPECIFIED.,.F.,.F.,(4,3,3,3,3,3,
3,3,3,3,3,3,3,3,4),(-48.0752275703878,-47.8005746714253,-47.302652018598,
-46.8047293657706,-46.3068067129433,-45.8088840601159,-45.3109614072886,
-44.8130387544612,-44.3151161016339,-43.8171934488065,-43.3192707959792,
-42.8213481431518,-42.3234254903245,-41.8255028374971,-41.7920422632082),
 .UNSPECIFIED.);
#1308=B_SPLINE_CURVE_WITH_KNOTS('',3,(#55313,#55314,#55315,#55316,#55317,
#55318,#55319,#55320,#55321,#55322,#55323,#55324,#55325,#55326,#55327,#55328,
#55329,#55330,#55331,#55332,#55333,#55334,#55335,#55336,#55337,#55338,#55339,
#55340,#55341,#55342,#55343,#55344,#55345,#55346,#55347,#55348,#55349,#55350,
#55351,#55352,#55353,#55354,#55355),.UNSPECIFIED.,.F.,.F.,(4,3,3,3,3,3,
3,3,3,3,3,3,3,3,4),(38.8227605492205,38.8379669205331,39.3358895733604,
39.8338122261878,40.3317348790151,40.8296575318425,41.3275801846698,41.8255028374971,
42.3234254903245,42.8213481431518,43.3192707959792,43.8171934488065,44.3151161016339,
44.8130387544612,45.1059458564001),.UNSPECIFIED.);
#1309=B_SPLINE_CURVE_WITH_KNOTS('',3,(#55360,#55361,#55362,#55363,#55364,
#55365,#55366,#55367,#55368,#55369,#55370,#55371,#55372,#55373,#55374,#55375,
#55376,#55377,#55378,#55379,#55380,#55381,#55382,#55383,#55384,#55385,#55386,
#55387,#55388,#55389,#55390,#55391,#55392,#55393,#55394,#55395,#55396,#55397,
#55398,#55399,#55400,#55401,#55402),.UNSPECIFIED.,.F.,.F.,(4,3,3,3,3,3,
3,3,3,3,3,3,3,3,4),(-54.3584128775674,-54.2735691581808,-53.7756465053535,
-53.2777238525261,-52.7798011996988,-52.2818785468714,-51.7839558940441,
-51.2860332412167,-50.7881105883894,-50.290187935562,-49.7922652827347,
-49.2943426299073,-48.79641997708,-48.2984973242527,-48.0752275703878),
 .UNSPECIFIED.);
#1310=B_SPLINE_CURVE_WITH_KNOTS('',3,(#55403,#55404,#55405,#55406,#55407,
#55408,#55409,#55410,#55411,#55412,#55413,#55414,#55415,#55416,#55417,#55418,
#55419,#55420,#55421,#55422,#55423,#55424,#55425,#55426,#55427,#55428,#55429,
#55430,#55431,#55432,#55433,#55434,#55435,#55436,#55437,#55438,#55439,#55440,
#55441,#55442,#55443,#55444,#55445),.UNSPECIFIED.,.F.,.F.,(4,3,3,3,3,3,
3,3,3,3,3,3,3,3,4),(45.1059458564001,45.3109614072886,45.8088840601159,
46.3068067129433,46.8047293657706,47.302652018598,47.8005746714253,48.2984973242527,
48.79641997708,49.2943426299074,49.7922652827347,50.2901879355621,50.7881105883894,
51.2860332412167,51.3891311635797),.UNSPECIFIED.);
#1311=B_SPLINE_CURVE_WITH_KNOTS('',3,(#55450,#55451,#55452,#55453,#55454,
#55455,#55456,#55457,#55458,#55459,#55460,#55461,#55462,#55463,#55464,#55465,
#55466,#55467,#55468,#55469,#55470,#55471,#55472,#55473,#55474,#55475,#55476,
#55477,#55478,#55479,#55480,#55481,#55482,#55483,#55484,#55485,#55486,#55487,
#55488,#55489),.UNSPECIFIED.,.F.,.F.,(4,3,3,3,3,3,3,3,3,3,3,3,3,4),(-60.641598184747,
-60.248640992109,-59.7507183392816,-59.2527956864543,-58.754873033627,-58.2569503807996,
-57.7590277279723,-57.2611050751449,-56.7631824223175,-56.2652597694902,
-55.7673371166629,-55.2694144638355,-54.7714918110082,-54.3584128775674),
 .UNSPECIFIED.);
#1312=B_SPLINE_CURVE_WITH_KNOTS('',3,(#55490,#55491,#55492,#55493,#55494,
#55495,#55496,#55497,#55498,#55499,#55500,#55501,#55502,#55503,#55504,#55505,
#55506,#55507,#55508,#55509,#55510,#55511,#55512,#55513,#55514,#55515,#55516,
#55517,#55518,#55519,#55520,#55521,#55522,#55523,#55524,#55525,#55526,#55527,
#55528,#55529),.UNSPECIFIED.,.F.,.F.,(4,3,3,3,3,3,3,3,3,3,3,3,3,4),(51.3891311635797,
51.7839558940441,52.2818785468714,52.7798011996988,53.2777238525261,53.7756465053535,
54.2735691581808,54.7714918110082,55.2694144638355,55.7673371166629,56.2652597694902,
56.7631824223176,57.2611050751449,57.6723164707593),.UNSPECIFIED.);
#1313=B_SPLINE_CURVE_WITH_KNOTS('',3,(#55534,#55535,#55536,#55537,#55538,
#55539,#55540,#55541,#55542,#55543,#55544,#55545,#55546,#55547,#55548,#55549,
#55550,#55551,#55552,#55553,#55554,#55555,#55556,#55557,#55558,#55559,#55560,
#55561,#55562,#55563,#55564,#55565,#55566,#55567,#55568,#55569,#55570,#55571,
#55572,#55573,#55574,#55575,#55576),.UNSPECIFIED.,.F.,.F.,(4,3,3,3,3,3,
3,3,3,3,3,3,3,3,4),(-66.9247834919266,-66.7216354788645,-66.2237128260371,
-65.7257901732098,-65.2278675203824,-64.7299448675551,-64.2320222147278,
-63.7340995619004,-63.2361769090731,-62.7382542562457,-62.2403316034184,
-61.742408950591,-61.2444862977637,-60.7465636449363,-60.641598184747),
 .UNSPECIFIED.);
#1314=B_SPLINE_CURVE_WITH_KNOTS('',3,(#55577,#55578,#55579,#55580,#55581,
#55582,#55583,#55584,#55585,#55586,#55587,#55588,#55589,#55590,#55591,#55592,
#55593,#55594,#55595,#55596,#55597,#55598,#55599,#55600,#55601,#55602,#55603,
#55604,#55605,#55606,#55607,#55608,#55609,#55610,#55611,#55612,#55613,#55614,
#55615,#55616,#55617,#55618,#55619),.UNSPECIFIED.,.F.,.F.,(4,3,3,3,3,3,
3,3,3,3,3,3,3,3,4),(57.6723164707593,57.7590277279723,58.2569503807996,
58.754873033627,59.2527956864543,59.7507183392817,60.248640992109,60.7465636449363,
61.2444862977637,61.742408950591,62.2403316034184,62.7382542562457,63.2361769090731,
63.7340995619004,63.9555017779389),.UNSPECIFIED.);
#1315=B_SPLINE_CURVE_WITH_KNOTS('',3,(#55624,#55625,#55626,#55627,#55628,
#55629,#55630,#55631,#55632,#55633,#55634,#55635,#55636,#55637,#55638,#55639,
#55640,#55641,#55642,#55643,#55644,#55645,#55646,#55647,#55648,#55649,#55650,
#55651,#55652,#55653,#55654,#55655,#55656,#55657,#55658,#55659,#55660,#55661,
#55662,#55663,#55664,#55665,#55666),.UNSPECIFIED.,.F.,.F.,(4,3,3,3,3,3,
3,3,3,3,3,3,3,3,4),(-73.2079687991062,-73.19462996562,-72.6967073127926,
-72.1987846599653,-71.700862007138,-71.2029393543106,-70.7050167014833,
-70.2070940486559,-69.7091713958286,-69.2112487430012,-68.7133260901739,
-68.2154034373465,-67.7174807845192,-67.2195581316918,-66.9247834919266),
 .UNSPECIFIED.);
#1316=B_SPLINE_CURVE_WITH_KNOTS('',3,(#55667,#55668,#55669,#55670,#55671,
#55672,#55673,#55674,#55675,#55676,#55677,#55678,#55679,#55680,#55681,#55682,
#55683,#55684,#55685,#55686,#55687,#55688,#55689,#55690,#55691,#55692,#55693,
#55694,#55695,#55696,#55697,#55698,#55699,#55700,#55701,#55702,#55703,#55704,
#55705,#55706,#55707,#55708,#55709),.UNSPECIFIED.,.F.,.F.,(4,3,3,3,3,3,
3,3,3,3,3,3,3,3,4),(63.9555017779389,64.2320222147278,64.7299448675551,
65.2278675203825,65.7257901732098,66.2237128260372,66.7216354788645,67.2195581316918,
67.7174807845192,68.2154034373465,68.7133260901739,69.2112487430012,69.7091713958286,
70.2070940486559,70.2386870851185),.UNSPECIFIED.);
#1317=B_SPLINE_CURVE_WITH_KNOTS('',3,(#55714,#55715,#55716,#55717,#55718,
#55719,#55720,#55721,#55722,#55723,#55724,#55725,#55726,#55727,#55728,#55729,
#55730,#55731,#55732,#55733,#55734,#55735,#55736,#55737,#55738,#55739,#55740,
#55741,#55742,#55743,#55744,#55745,#55746,#55747,#55748,#55749,#55750,#55751,
#55752,#55753),.UNSPECIFIED.,.F.,.F.,(4,3,3,3,3,3,3,3,3,3,3,3,3,4),(-79.4911541062858,
-79.1697017995482,-78.6717791467208,-78.1738564938935,-77.6759338410661,
-77.1780111882388,-76.6800885354114,-76.1821658825841,-75.6842432297567,
-75.1863205769294,-74.688397924102,-74.1904752712747,-73.6925526184473,
-73.2079687991062),.UNSPECIFIED.);
#1318=B_SPLINE_CURVE_WITH_KNOTS('',3,(#55754,#55755,#55756,#55757,#55758,
#55759,#55760,#55761,#55762,#55763,#55764,#55765,#55766,#55767,#55768,#55769,
#55770,#55771,#55772,#55773,#55774,#55775,#55776,#55777,#55778,#55779,#55780,
#55781,#55782,#55783,#55784,#55785,#55786,#55787,#55788,#55789,#55790,#55791,
#55792,#55793),.UNSPECIFIED.,.F.,.F.,(4,3,3,3,3,3,3,3,3,3,3,3,3,4),(70.2386870851185,
70.7050167014833,71.2029393543106,71.700862007138,72.1987846599653,72.6967073127927,
73.19462996562,73.6925526184474,74.1904752712747,74.688397924102,75.1863205769294,
75.6842432297567,76.1821658825841,76.5218723922981),.UNSPECIFIED.);
#1319=B_SPLINE_CURVE_WITH_KNOTS('',3,(#55798,#55799,#55800,#55801,#55802,
#55803,#55804,#55805,#55806,#55807,#55808,#55809,#55810,#55811,#55812,#55813,
#55814,#55815,#55816,#55817,#55818,#55819,#55820,#55821,#55822,#55823,#55824,
#55825,#55826,#55827,#55828,#55829,#55830,#55831,#55832,#55833,#55834,#55835,
#55836,#55837,#55838,#55839,#55840),.UNSPECIFIED.,.F.,.F.,(4,3,3,3,3,3,
3,3,3,3,3,3,3,3,4),(-85.7743394134654,-85.6426962863037,-85.1447736334763,
-84.646850980649,-84.1489283278216,-83.6510056749943,-83.153083022167,-82.6551603693396,
-82.1572377165122,-81.6593150636849,-81.1613924108575,-80.6634697580302,
-80.1655471052028,-79.6676244523755,-79.4911541062858),.UNSPECIFIED.);
#1320=B_SPLINE_CURVE_WITH_KNOTS('',3,(#55841,#55842,#55843,#55844,#55845,
#55846,#55847,#55848,#55849,#55850,#55851,#55852,#55853,#55854,#55855,#55856,
#55857,#55858,#55859,#55860,#55861,#55862,#55863,#55864,#55865,#55866,#55867,
#55868,#55869,#55870,#55871,#55872,#55873,#55874,#55875,#55876,#55877,#55878,
#55879,#55880,#55881,#55882,#55883),.UNSPECIFIED.,.F.,.F.,(4,3,3,3,3,3,
3,3,3,3,3,3,3,3,4),(76.5218723922981,76.6800885354114,77.1780111882388,
77.6759338410661,78.1738564938935,78.6717791467208,79.1697017995482,79.6676244523755,
80.1655471052028,80.6634697580302,81.1613924108576,81.6593150636849,82.1572377165122,
82.6551603693396,82.8050576994777),.UNSPECIFIED.);
#1321=B_SPLINE_CURVE_WITH_KNOTS('',3,(#55888,#55889,#55890,#55891,#55892,
#55893,#55894,#55895,#55896,#55897,#55898,#55899,#55900,#55901,#55902,#55903,
#55904,#55905,#55906,#55907,#55908,#55909,#55910,#55911,#55912,#55913,#55914,
#55915,#55916,#55917,#55918,#55919,#55920,#55921,#55922,#55923,#55924,#55925,
#55926,#55927),.UNSPECIFIED.,.F.,.F.,(4,3,3,3,3,3,3,3,3,3,3,3,3,4),(-92.057524720645,
-91.6177681202318,-91.1198454674045,-90.6219228145771,-90.1240001617498,
-89.6260775089224,-89.1281548560951,-88.6302322032678,-88.1323095504404,
-87.6343868976131,-87.1364642447857,-86.6385415919584,-86.140618939131,
-85.7743394134654),.UNSPECIFIED.);
#1322=B_SPLINE_CURVE_WITH_KNOTS('',3,(#55928,#55929,#55930,#55931,#55932,
#55933,#55934,#55935,#55936,#55937,#55938,#55939,#55940,#55941,#55942,#55943,
#55944,#55945,#55946,#55947,#55948,#55949,#55950,#55951,#55952,#55953,#55954,
#55955,#55956,#55957,#55958,#55959,#55960,#55961,#55962,#55963,#55964,#55965,
#55966,#55967),.UNSPECIFIED.,.F.,.F.,(4,3,3,3,3,3,3,3,3,3,3,3,3,4),(82.8050576994777,
83.1530830221669,83.6510056749943,84.1489283278216,84.646850980649,85.1447736334763,
85.6426962863037,86.140618939131,86.6385415919584,87.1364642447857,87.6343868976131,
88.1323095504404,88.6302322032678,89.0882430066573),.UNSPECIFIED.);
#1323=B_SPLINE_CURVE_WITH_KNOTS('',3,(#55972,#55973,#55974,#55975,#55976,
#55977,#55978,#55979,#55980,#55981,#55982,#55983,#55984,#55985,#55986,#55987,
#55988,#55989,#55990,#55991,#55992,#55993,#55994,#55995,#55996,#55997,#55998,
#55999,#56000,#56001,#56002,#56003,#56004,#56005,#56006,#56007,#56008,#56009,
#56010,#56011,#56012,#56013,#56014),.UNSPECIFIED.,.F.,.F.,(4,3,3,3,3,3,
3,3,3,3,3,3,3,3,4),(-98.3407100278245,-98.0907626069873,-97.59283995416,
-97.0949173013326,-96.5969946485053,-96.099071995678,-95.6011493428506,
-95.1032266900232,-94.6053040371959,-94.1073813843686,-93.6094587315412,
-93.1115360787139,-92.6136134258865,-92.1156907730592,-92.057524720645),
 .UNSPECIFIED.);
#1324=B_SPLINE_CURVE_WITH_KNOTS('',3,(#56015,#56016,#56017,#56018,#56019,
#56020,#56021,#56022,#56023,#56024,#56025,#56026,#56027,#56028,#56029,#56030,
#56031,#56032,#56033,#56034,#56035,#56036,#56037,#56038,#56039,#56040,#56041,
#56042,#56043,#56044,#56045,#56046,#56047,#56048,#56049,#56050,#56051,#56052,
#56053,#56054,#56055,#56056,#56057),.UNSPECIFIED.,.F.,.F.,(4,3,3,3,3,3,
3,3,3,3,3,3,3,3,4),(89.0882430066573,89.1281548560951,89.6260775089225,
90.1240001617498,90.6219228145772,91.1198454674045,91.6177681202318,92.1156907730592,
92.6136134258865,93.1115360787139,93.6094587315412,94.1073813843686,94.6053040371959,
95.1032266900233,95.3714283138369),.UNSPECIFIED.);
#1325=B_SPLINE_CURVE_WITH_KNOTS('',3,(#56062,#56063,#56064,#56065,#56066,
#56067,#56068,#56069,#56070,#56071,#56072,#56073,#56074,#56075,#56076,#56077,
#56078,#56079,#56080,#56081,#56082,#56083,#56084,#56085,#56086,#56087,#56088,
#56089,#56090,#56091,#56092,#56093,#56094,#56095,#56096,#56097,#56098,#56099,
#56100,#56101,#56102,#56103,#56104),.UNSPECIFIED.,.F.,.F.,(4,3,3,3,3,3,
3,3,3,3,3,3,3,3,4),(-104.623895335004,-104.563757093743,-104.065834440916,
-103.567911788088,-103.069989135261,-102.572066482433,-102.074143829606,
-101.576221176779,-101.078298523951,-100.580375871124,-100.082453218297,
-99.5845305654694,-99.086607912642,-98.5886852598147,-98.3407100278245),
 .UNSPECIFIED.);
#1326=B_SPLINE_CURVE_WITH_KNOTS('',3,(#56105,#56106,#56107,#56108,#56109,
#56110,#56111,#56112,#56113,#56114,#56115,#56116,#56117,#56118,#56119,#56120,
#56121,#56122,#56123,#56124,#56125,#56126,#56127,#56128,#56129,#56130,#56131,
#56132,#56133,#56134,#56135,#56136,#56137,#56138,#56139,#56140,#56141,#56142,
#56143,#56144,#56145,#56146,#56147),.UNSPECIFIED.,.F.,.F.,(4,3,3,3,3,3,
3,3,3,3,3,3,3,3,4),(95.3714283138369,95.6011493428506,96.099071995678,96.5969946485053,
97.0949173013327,97.59283995416,98.0907626069874,98.5886852598147,99.0866079126421,
99.5845305654694,100.082453218297,100.580375871124,101.078298523951,101.576221176779,
101.654613621016),.UNSPECIFIED.);
#1327=B_SPLINE_CURVE_WITH_KNOTS('',3,(#56152,#56153,#56154,#56155,#56156,
#56157,#56158,#56159,#56160,#56161,#56162,#56163,#56164,#56165,#56166,#56167,
#56168,#56169,#56170,#56171,#56172,#56173,#56174,#56175,#56176,#56177,#56178,
#56179,#56180,#56181,#56182,#56183,#56184,#56185,#56186,#56187,#56188,#56189,
#56190,#56191),.UNSPECIFIED.,.F.,.F.,(4,3,3,3,3,3,3,3,3,3,3,3,3,4),(-110.907080642184,
-110.538828927671,-110.040906274844,-109.542983622016,-109.045060969189,
-108.547138316362,-108.049215663534,-107.551293010707,-107.05337035788,
-106.555447705052,-106.057525052225,-105.559602399398,-105.06167974657,
-104.623895335004),.UNSPECIFIED.);
#1328=B_SPLINE_CURVE_WITH_KNOTS('',3,(#56192,#56193,#56194,#56195,#56196,
#56197,#56198,#56199,#56200,#56201,#56202,#56203,#56204,#56205,#56206,#56207,
#56208,#56209,#56210,#56211,#56212,#56213,#56214,#56215,#56216,#56217,#56218,
#56219,#56220,#56221,#56222,#56223,#56224,#56225,#56226,#56227,#56228,#56229,
#56230,#56231),.UNSPECIFIED.,.F.,.F.,(4,3,3,3,3,3,3,3,3,3,3,3,3,4),(101.654613621016,
102.074143829606,102.572066482433,103.069989135261,103.567911788088,104.065834440916,
104.563757093743,105.06167974657,105.559602399398,106.057525052225,106.555447705052,
107.05337035788,107.551293010707,107.937798928196),.UNSPECIFIED.);
#1329=B_SPLINE_CURVE_WITH_KNOTS('',3,(#56236,#56237,#56238,#56239,#56240,
#56241,#56242,#56243,#56244,#56245,#56246,#56247,#56248,#56249,#56250,#56251,
#56252,#56253,#56254,#56255,#56256,#56257,#56258,#56259,#56260,#56261,#56262,
#56263,#56264,#56265,#56266,#56267,#56268,#56269,#56270,#56271,#56272,#56273,
#56274,#56275,#56276,#56277,#56278),.UNSPECIFIED.,.F.,.F.,(4,3,3,3,3,3,
3,3,3,3,3,3,3,3,4),(-117.190265949363,-117.011823414427,-116.513900761599,
-116.015978108772,-115.518055455944,-115.020132803117,-114.52221015029,
-114.024287497462,-113.526364844635,-113.028442191808,-112.53051953898,
-112.032596886153,-111.534674233326,-111.036751580498,-110.907080642184),
 .UNSPECIFIED.);
#1330=B_SPLINE_CURVE_WITH_KNOTS('',3,(#56279,#56280,#56281,#56282,#56283,
#56284,#56285,#56286,#56287,#56288,#56289,#56290,#56291,#56292,#56293,#56294,
#56295,#56296,#56297,#56298,#56299,#56300,#56301,#56302,#56303,#56304,#56305,
#56306,#56307,#56308,#56309,#56310,#56311,#56312,#56313,#56314,#56315,#56316,
#56317,#56318,#56319,#56320,#56321),.UNSPECIFIED.,.F.,.F.,(4,3,3,3,3,3,
3,3,3,3,3,3,3,3,4),(107.937798928196,108.049215663534,108.547138316362,
109.045060969189,109.542983622016,110.040906274844,110.538828927671,111.036751580498,
111.534674233326,112.032596886153,112.53051953898,113.028442191808,113.526364844635,
114.024287497462,114.220984235376),.UNSPECIFIED.);
#1331=B_SPLINE_CURVE_WITH_KNOTS('',3,(#56327,#56328,#56329,#56330),
 .UNSPECIFIED.,.F.,.F.,(4,4),(128.805298797182,129.041483053697),
 .UNSPECIFIED.);
#1332=B_SPLINE_CURVE_WITH_KNOTS('',3,(#56336,#56337,#56338,#56339,#56340,
#56341,#56342,#56343,#56344,#56345,#56346,#56347,#56348,#56349,#56350,#56351,
#56352),.UNSPECIFIED.,.F.,.F.,(4,1,1,1,1,1,1,1,1,1,1,1,1,1,4),(122.522113490002,
122.651784428317,123.149707081144,123.647629733971,124.145552386799,124.643475039626,
125.141397692453,125.639320345281,126.137242998108,126.635165650935,127.133088303763,
127.63101095659,128.128933609417,128.626856262245,128.805298797182),
 .UNSPECIFIED.);
#1333=B_SPLINE_CURVE_WITH_KNOTS('',3,(#56355,#56356,#56357,#56358,#56359,
#56360,#56361,#56362,#56363,#56364,#56365,#56366,#56367,#56368),
 .UNSPECIFIED.,.F.,.F.,(4,1,1,1,1,1,1,1,1,1,1,4),(122.522113490002,122.823339404916,
123.321262057743,123.819184710571,124.317107363398,124.815030016225,125.312952669053,
125.81087532188,126.308797974707,126.806720627535,127.304643280362,127.802565933189),
 .UNSPECIFIED.);
#1334=B_SPLINE_CURVE_WITH_KNOTS('',3,(#56373,#56374,#56375,#56376,#56377,
#56378,#56379,#56380,#56381,#56382,#56383,#56384,#56385,#56386,#56387,#56388),
 .UNSPECIFIED.,.F.,.F.,(4,1,1,1,1,1,1,1,1,1,1,1,1,4),(116.238928182822,
116.676712594388,117.174635247216,117.672557900043,118.17048055287,118.668403205698,
119.166325858525,119.664248511352,120.16217116418,120.660093817007,121.158016469834,
121.655939122662,122.153861775489,122.522113490002),.UNSPECIFIED.);
#1335=B_SPLINE_CURVE_WITH_KNOTS('',3,(#56389,#56390,#56391,#56392,#56393,
#56394,#56395,#56396,#56397,#56398,#56399,#56400,#56401,#56402,#56403,#56404,
#56405),.UNSPECIFIED.,.F.,.F.,(4,1,1,1,1,1,1,1,1,1,1,1,1,1,4),(116.238928182822,
116.35034491816,116.848267570988,117.346190223815,117.844112876642,118.34203552947,
118.839958182297,119.337880835125,119.835803487952,120.333726140779,120.831648793607,
121.329571446434,121.827494099261,122.325416752089,122.522113490002),
 .UNSPECIFIED.);
#1336=B_SPLINE_CURVE_WITH_KNOTS('',3,(#56410,#56411,#56412,#56413,#56414,
#56415,#56416,#56417,#56418,#56419,#56420,#56421,#56422,#56423,#56424,#56425,
#56426),.UNSPECIFIED.,.F.,.F.,(4,1,1,1,1,1,1,1,1,1,1,1,1,1,4),(109.955742875643,
110.203718107633,110.70164076046,111.199563413288,111.697486066115,112.195408718942,
112.69333137177,113.191254024597,113.689176677424,114.187099330252,114.685021983079,
115.182944635906,115.680867288734,116.178789941561,116.238928182822),
 .UNSPECIFIED.);
#1337=B_SPLINE_CURVE_WITH_KNOTS('',3,(#56427,#56428,#56429,#56430,#56431,
#56432,#56433,#56434,#56435,#56436,#56437,#56438,#56439,#56440,#56441,#56442),
 .UNSPECIFIED.,.F.,.F.,(4,1,1,1,1,1,1,1,1,1,1,1,1,4),(109.955742875643,
110.375273084232,110.87319573706,111.371118389887,111.869041042714,112.366963695542,
112.864886348369,113.362809001196,113.860731654024,114.358654306851,114.856576959678,
115.354499612506,115.852422265333,116.238928182822),.UNSPECIFIED.);
#1338=B_SPLINE_CURVE_WITH_KNOTS('',3,(#56447,#56448,#56449,#56450,#56451,
#56452,#56453,#56454,#56455,#56456,#56457,#56458,#56459,#56460,#56461,#56462,
#56463),.UNSPECIFIED.,.F.,.F.,(4,1,1,1,1,1,1,1,1,1,1,1,1,1,4),(103.672557568463,
103.730723620877,104.228646273705,104.726568926532,105.224491579359,105.722414232187,
106.220336885014,106.718259537841,107.216182190669,107.714104843496,108.212027496323,
108.709950149151,109.207872801978,109.705795454805,109.955742875643),
 .UNSPECIFIED.);
#1339=B_SPLINE_CURVE_WITH_KNOTS('',3,(#56464,#56465,#56466,#56467,#56468,
#56469,#56470,#56471,#56472,#56473,#56474,#56475,#56476,#56477,#56478,#56479,
#56480),.UNSPECIFIED.,.F.,.F.,(4,1,1,1,1,1,1,1,1,1,1,1,1,1,4),(103.672557568463,
103.902278597477,104.400201250304,104.898123903131,105.396046555959,105.893969208786,
106.391891861613,106.889814514441,107.387737167268,107.885659820096,108.383582472923,
108.88150512575,109.379427778578,109.877350431405,109.955742875643),
 .UNSPECIFIED.);
#1340=B_SPLINE_CURVE_WITH_KNOTS('',3,(#56485,#56486,#56487,#56488,#56489,
#56490,#56491,#56492,#56493,#56494,#56495,#56496,#56497,#56498,#56499,#56500),
 .UNSPECIFIED.,.F.,.F.,(4,1,1,1,1,1,1,1,1,1,1,1,1,4),(97.3893722612835,
97.7556517869492,98.2535744397765,98.7514970926039,99.2494197454312,99.7473423982586,
100.245265051086,100.743187703913,101.241110356741,101.739033009568,102.236955662395,
102.734878315223,103.23280096805,103.672557568463),.UNSPECIFIED.);
#1341=B_SPLINE_CURVE_WITH_KNOTS('',3,(#56501,#56502,#56503,#56504,#56505,
#56506,#56507,#56508,#56509,#56510,#56511,#56512,#56513,#56514,#56515,#56516,
#56517),.UNSPECIFIED.,.F.,.F.,(4,1,1,1,1,1,1,1,1,1,1,1,1,1,4),(97.3893722612835,
97.4292841107213,97.9272067635486,98.4251294163759,98.9230520692033,99.4209747220306,
99.918897374858,100.416820027685,100.914742680513,101.41266533334,101.910587986167,
102.408510638995,102.906433291822,103.404355944649,103.672557568463),
 .UNSPECIFIED.);
#1342=B_SPLINE_CURVE_WITH_KNOTS('',3,(#56522,#56523,#56524,#56525,#56526,
#56527,#56528,#56529,#56530,#56531,#56532,#56533,#56534,#56535,#56536,#56537,
#56538),.UNSPECIFIED.,.F.,.F.,(4,1,1,1,1,1,1,1,1,1,1,1,1,1,4),(91.106186954104,
91.2826573001937,91.780579953021,92.2785026058484,92.7764252586757,93.2743479115031,
93.7722705643304,94.2701932171578,94.7681158699851,95.2660385228125,95.7639611756398,
96.2618838284671,96.7598064812945,97.2577291341218,97.3893722612835),
 .UNSPECIFIED.);
#1343=B_SPLINE_CURVE_WITH_KNOTS('',3,(#56539,#56540,#56541,#56542,#56543,
#56544,#56545,#56546,#56547,#56548,#56549,#56550,#56551,#56552,#56553,#56554),
 .UNSPECIFIED.,.F.,.F.,(4,1,1,1,1,1,1,1,1,1,1,1,1,4),(91.106186954104,91.4542122767931,
91.9521349296204,92.4500575824478,92.9479802352751,93.4459028881025,93.9438255409298,
94.4417481937572,94.9396708465845,95.4375934994119,95.9355161522392,96.4334388050665,
96.9313614578939,97.3893722612835),.UNSPECIFIED.);
#1344=B_SPLINE_CURVE_WITH_KNOTS('',3,(#56559,#56560,#56561,#56562,#56563,
#56564,#56565,#56566,#56567,#56568,#56569,#56570,#56571,#56572,#56573,#56574),
 .UNSPECIFIED.,.F.,.F.,(4,1,1,1,1,1,1,1,1,1,1,1,1,4),(84.8230016469244,
85.3075854662655,85.8055081190928,86.3034307719202,86.8013534247476,87.2992760775749,
87.7971987304022,88.2951213832296,88.7930440360569,89.2909666888843,89.7888893417116,
90.286811994539,90.7847346473663,91.106186954104),.UNSPECIFIED.);
#1345=B_SPLINE_CURVE_WITH_KNOTS('',3,(#56575,#56576,#56577,#56578,#56579,
#56580,#56581,#56582,#56583,#56584,#56585,#56586,#56587,#56588,#56589,#56590,
#56591),.UNSPECIFIED.,.F.,.F.,(4,1,1,1,1,1,1,1,1,1,1,1,1,1,4),(84.8230016469244,
84.9812177900376,85.4791404428649,85.9770630956923,86.4749857485196,86.972908401347,
87.4708310541743,87.9687537070017,88.466676359829,88.9645990126564,89.4625216654837,
89.960444318311,90.4583669711384,90.9562896239657,91.106186954104),
 .UNSPECIFIED.);
#1346=B_SPLINE_CURVE_WITH_KNOTS('',3,(#56596,#56597,#56598,#56599,#56600,
#56601,#56602,#56603,#56604,#56605,#56606,#56607,#56608,#56609,#56610,#56611,
#56612),.UNSPECIFIED.,.F.,.F.,(4,1,1,1,1,1,1,1,1,1,1,1,1,1,4),(78.5398163397448,
78.83459097951,79.3325136323374,79.8304362851647,80.328358937992,80.8262815908194,
81.3242042436467,81.8221268964741,82.3200495493014,82.8179722021288,83.3158948549561,
83.8138175077835,84.3117401606108,84.8096628134382,84.8230016469244),
 .UNSPECIFIED.);
#1347=B_SPLINE_CURVE_WITH_KNOTS('',3,(#56613,#56614,#56615,#56616,#56617,
#56618,#56619,#56620,#56621,#56622,#56623,#56624,#56625,#56626,#56627,#56628),
 .UNSPECIFIED.,.F.,.F.,(4,1,1,1,1,1,1,1,1,1,1,1,1,4),(78.5398163397448,
79.0061459561094,79.5040686089368,80.0019912617641,80.4999139145914,80.9978365674188,
81.4957592202462,81.9936818730735,82.4916045259008,82.9895271787282,83.4874498315555,
83.9853724843829,84.4832951372102,84.8230016469244),.UNSPECIFIED.);
#1348=B_SPLINE_CURVE_WITH_KNOTS('',3,(#56633,#56634,#56635,#56636,#56637,
#56638,#56639,#56640,#56641,#56642,#56643,#56644,#56645,#56646,#56647,#56648,
#56649),.UNSPECIFIED.,.F.,.F.,(4,1,1,1,1,1,1,1,1,1,1,1,1,1,4),(72.2566310325652,
72.3615964927545,72.8595191455818,73.3574417984092,73.8553644512365,74.3532871040639,
74.8512097568912,75.3491324097186,75.8470550625459,76.3449777153733,76.8429003682006,
77.340823021028,77.8387456738553,78.3366683266827,78.5398163397448),
 .UNSPECIFIED.);
#1349=B_SPLINE_CURVE_WITH_KNOTS('',3,(#56650,#56651,#56652,#56653,#56654,
#56655,#56656,#56657,#56658,#56659,#56660,#56661,#56662,#56663,#56664,#56665,
#56666),.UNSPECIFIED.,.F.,.F.,(4,1,1,1,1,1,1,1,1,1,1,1,1,1,4),(72.2566310325652,
72.5331514693539,73.0310741221813,73.5289967750086,74.0269194278359,74.5248420806633,
75.0227647334906,75.520687386318,76.0186100391453,76.5165326919727,77.0144553448,
77.5123779976274,78.0103006504547,78.5082233032821,78.5398163397448),
 .UNSPECIFIED.);
#1350=B_SPLINE_CURVE_WITH_KNOTS('',3,(#56671,#56672,#56673,#56674,#56675,
#56676,#56677,#56678,#56679,#56680,#56681,#56682,#56683,#56684,#56685,#56686),
 .UNSPECIFIED.,.F.,.F.,(4,1,1,1,1,1,1,1,1,1,1,1,1,4),(65.9734457253856,
66.3865246588263,66.8844473116537,67.382369964481,67.8802926173084,68.3782152701357,
68.8761379229631,69.3740605757904,69.8719832286178,70.3699058814451,70.8678285342725,
71.3657511870998,71.8636738399271,72.2566310325652),.UNSPECIFIED.);
#1351=B_SPLINE_CURVE_WITH_KNOTS('',3,(#56687,#56688,#56689,#56690,#56691,
#56692,#56693,#56694,#56695,#56696,#56697,#56698,#56699,#56700,#56701,#56702,
#56703),.UNSPECIFIED.,.F.,.F.,(4,1,1,1,1,1,1,1,1,1,1,1,1,1,4),(65.9734457253856,
66.0601569825984,66.5580796354257,67.0560022882531,67.5539249410804,68.0518475939078,
68.5497702467351,69.0476928995625,69.5456155523898,70.0435382052172,70.5414608580445,
71.0393835108719,71.5373061636992,72.0352288165266,72.2566310325652),
 .UNSPECIFIED.);
#1352=B_SPLINE_CURVE_WITH_KNOTS('',3,(#56708,#56709,#56710,#56711,#56712,
#56713,#56714,#56715,#56716,#56717,#56718,#56719,#56720,#56721,#56722,#56723,
#56724),.UNSPECIFIED.,.F.,.F.,(4,1,1,1,1,1,1,1,1,1,1,1,1,1,4),(59.690260418206,
59.9135301720708,60.4114528248982,60.9093754777255,61.4072981305529,61.9052207833802,
62.4031434362076,62.9010660890349,63.3989887418622,63.8969113946896,64.3948340475169,
64.8927567003443,65.3906793531716,65.888602005999,65.9734457253856),
 .UNSPECIFIED.);
#1353=B_SPLINE_CURVE_WITH_KNOTS('',3,(#56725,#56726,#56727,#56728,#56729,
#56730,#56731,#56732,#56733,#56734,#56735,#56736,#56737,#56738,#56739,#56740),
 .UNSPECIFIED.,.F.,.F.,(4,1,1,1,1,1,1,1,1,1,1,1,1,4),(59.690260418206,60.0850851486702,
60.5830078014976,61.0809304543249,61.5788531071523,62.0767757599796,62.574698412807,
63.0726210656343,63.5705437184617,64.068466371289,64.5663890241163,65.0643116769437,
65.562234329771,65.9734457253856),.UNSPECIFIED.);
#1354=B_SPLINE_CURVE_WITH_KNOTS('',3,(#56745,#56746,#56747,#56748,#56749,
#56750,#56751,#56752,#56753,#56754,#56755,#56756,#56757,#56758,#56759,#56760,
#56761),.UNSPECIFIED.,.F.,.F.,(4,1,1,1,1,1,1,1,1,1,1,1,1,1,4),(53.4070751110264,
53.4405356853153,53.9384583381427,54.43638099097,54.9343036437973,55.4322262966247,
55.930148949452,56.4280716022794,56.9259942551067,57.4239169079341,57.9218395607614,
58.4197622135888,58.9176848664161,59.4156075192435,59.690260418206),
 .UNSPECIFIED.);
#1355=B_SPLINE_CURVE_WITH_KNOTS('',3,(#56762,#56763,#56764,#56765,#56766,
#56767,#56768,#56769,#56770,#56771,#56772,#56773,#56774,#56775,#56776,#56777,
#56778),.UNSPECIFIED.,.F.,.F.,(4,1,1,1,1,1,1,1,1,1,1,1,1,1,4),(53.4070751110264,
53.6120906619147,54.1100133147421,54.6079359675694,55.1058586203968,55.6037812732241,
56.1017039260515,56.5996265788788,57.0975492317061,57.5954718845335,58.0933945373608,
58.5913171901882,59.0892398430155,59.5871624958429,59.690260418206),
 .UNSPECIFIED.);
#1356=B_SPLINE_CURVE_WITH_KNOTS('',3,(#56783,#56784,#56785,#56786,#56787,
#56788,#56789,#56790,#56791,#56792,#56793,#56794,#56795,#56796,#56797,#56798),
 .UNSPECIFIED.,.F.,.F.,(4,1,1,1,1,1,1,1,1,1,1,1,1,4),(47.1238898038468,
47.4654638513871,47.9633865042145,48.4613091570418,48.9592318098692,49.4571544626965,
49.9550771155239,50.4529997683512,50.9509224211786,51.4488450740059,51.9467677268333,
52.4446903796606,52.942613032488,53.4070751110264),.UNSPECIFIED.);
#1357=B_SPLINE_CURVE_WITH_KNOTS('',3,(#56799,#56800,#56801,#56802,#56803,
#56804,#56805,#56806,#56807,#56808,#56809,#56810,#56811,#56812,#56813,#56814,
#56815),.UNSPECIFIED.,.F.,.F.,(4,1,1,1,1,1,1,1,1,1,1,1,1,1,4),(47.1238898038468,
47.1390961751592,47.6370188279866,48.1349414808139,48.6328641336412,49.1307867864686,
49.6287094392959,50.1266320921233,50.6245547449506,51.122477397778,51.6204000506053,
52.1183227034327,52.61624535626,53.1141680090874,53.4070751110264),
 .UNSPECIFIED.);
#1358=B_SPLINE_CURVE_WITH_KNOTS('',3,(#56820,#56821,#56822,#56823,#56824,
#56825,#56826,#56827,#56828,#56829,#56830,#56831,#56832,#56833,#56834,#56835,
#56836),.UNSPECIFIED.,.F.,.F.,(4,1,1,1,1,1,1,1,1,1,1,1,1,1,4),(40.8407044966672,
40.9924693646316,41.490392017459,41.9883146702863,42.4862373231137,42.984159975941,
43.4820826287684,43.9800052815957,44.4779279344231,44.9758505872504,45.4737732400778,
45.9716958929051,46.4696185457325,46.9675411985598,47.1238898038468),
 .UNSPECIFIED.);
#1359=B_SPLINE_CURVE_WITH_KNOTS('',3,(#56837,#56838,#56839,#56840,#56841,
#56842,#56843,#56844,#56845,#56846,#56847,#56848,#56849,#56850,#56851,#56852),
 .UNSPECIFIED.,.F.,.F.,(4,1,1,1,1,1,1,1,1,1,1,1,1,4),(40.8407044966672,
41.164024341231,41.6619469940584,42.1598696468857,42.6577922997131,43.1557149525404,
43.6536376053678,44.1515602581951,44.6494829110225,45.1474055638498,45.6453282166772,
46.1432508695045,46.6411735223319,47.1238898038468),.UNSPECIFIED.);
#1360=B_SPLINE_CURVE_WITH_KNOTS('',3,(#56857,#56858,#56859,#56860,#56861,
#56862,#56863,#56864,#56865,#56866,#56867,#56868,#56869,#56870,#56871,#56872),
 .UNSPECIFIED.,.F.,.F.,(4,1,1,1,1,1,1,1,1,1,1,1,1,4),(34.5575191894876,
35.0173975307035,35.5153201835308,36.0132428363582,36.5111654891855,37.0090881420129,
37.5070107948402,38.0049334476676,38.5028561004949,39.0007787533223,39.4987014061496,
39.9966240589769,40.4945467118043,40.8407044966672),.UNSPECIFIED.);
#1361=B_SPLINE_CURVE_WITH_KNOTS('',3,(#56873,#56874,#56875,#56876,#56877,
#56878,#56879,#56880,#56881,#56882,#56883,#56884,#56885,#56886,#56887,#56888,
#56889),.UNSPECIFIED.,.F.,.F.,(4,1,1,1,1,1,1,1,1,1,1,1,1,1,4),(34.5575191894876,
34.6910298544755,35.1889525073029,35.6868751601302,36.1847978129576,36.6827204657849,
37.1806431186123,37.6785657714396,38.176488424267,38.6744110770943,39.1723337299217,
39.670256382749,40.1681790355763,40.6661016884037,40.8407044966672),
 .UNSPECIFIED.);
#1362=B_SPLINE_CURVE_WITH_KNOTS('',3,(#56894,#56895,#56896,#56897,#56898,
#56899,#56900,#56901,#56902,#56903,#56904,#56905,#56906,#56907,#56908,#56909,
#56910),.UNSPECIFIED.,.F.,.F.,(4,1,1,1,1,1,1,1,1,1,1,1,1,1,4),(28.274333882308,
28.544403043948,29.0423256967753,29.5402483496027,30.03817100243,30.5360936552574,
31.0340163080847,31.5319389609121,32.0298616137394,32.5277842665667,33.0257069193941,
33.5236295722214,34.0215522250488,34.5194748778761,34.5575191894876),
 .UNSPECIFIED.);
#1363=B_SPLINE_CURVE_WITH_KNOTS('',3,(#56911,#56912,#56913,#56914,#56915,
#56916,#56917,#56918,#56919,#56920,#56921,#56922,#56923,#56924,#56925,#56926),
 .UNSPECIFIED.,.F.,.F.,(4,1,1,1,1,1,1,1,1,1,1,1,1,4),(28.274333882308,28.7159580205474,
29.2138806733747,29.7118033262021,30.2097259790294,30.7076486318568,31.2055712846841,
31.7034939375114,32.2014165903388,32.6993392431661,33.1972618959935,33.6951845488208,
34.1931072016482,34.5575191894876),.UNSPECIFIED.);
#1364=B_SPLINE_CURVE_WITH_KNOTS('',3,(#56931,#56932,#56933,#56934,#56935,
#56936,#56937,#56938,#56939,#56940,#56941,#56942,#56943,#56944,#56945,#56946,
#56947),.UNSPECIFIED.,.F.,.F.,(4,1,1,1,1,1,1,1,1,1,1,1,1,1,4),(21.9911485751285,
22.0714085571925,22.5693312100198,23.0672538628472,23.5651765156745,24.0630991685018,
24.5610218213292,25.0589444741565,25.5568671269839,26.0547897798112,26.5527124326386,
27.0506350854659,27.5485577382933,28.0464803911206,28.274333882308),
 .UNSPECIFIED.);
#1365=B_SPLINE_CURVE_WITH_KNOTS('',3,(#56948,#56949,#56950,#56951,#56952,
#56953,#56954,#56955,#56956,#56957,#56958,#56959,#56960,#56961,#56962,#56963,
#56964),.UNSPECIFIED.,.F.,.F.,(4,1,1,1,1,1,1,1,1,1,1,1,1,1,4),(21.9911485751284,
22.2429635337919,22.7408861866192,23.2388088394466,23.7367314922739,24.2346541451012,
24.7325767979286,25.2304994507559,25.7284221035833,26.2263447564106,26.724267409238,
27.2221900620653,27.7201127148927,28.21803536772,28.274333882308),
 .UNSPECIFIED.);
#1366=B_SPLINE_CURVE_WITH_KNOTS('',3,(#56969,#56970,#56971,#56972,#56973,
#56974,#56975,#56976,#56977,#56978,#56979,#56980,#56981,#56982,#56983,#56984),
 .UNSPECIFIED.,.F.,.F.,(4,1,1,1,1,1,1,1,1,1,1,1,1,4),(15.7079632679489,
16.0963367232643,16.5942593760916,17.092182028919,17.5901046817463,18.0880273345737,
18.585949987401,19.0838726402284,19.5817952930557,20.0797179458831,20.5776405987104,
21.0755632515378,21.5734859043651,21.9911485751285),.UNSPECIFIED.);
#1367=B_SPLINE_CURVE_WITH_KNOTS('',3,(#56985,#56986,#56987,#56988,#56989,
#56990,#56991,#56992,#56993,#56994,#56995,#56996,#56997,#56998,#56999,#57000,
#57001),.UNSPECIFIED.,.F.,.F.,(4,1,1,1,1,1,1,1,1,1,1,1,1,1,4),(15.7079632679489,
15.7699690470363,16.2678916998637,16.765814352691,17.2637370055184,17.7616596583457,
18.2595823111731,18.7575049640004,19.2554276168278,19.7533502696551,20.2512729224825,
20.7491955753098,21.2471182281372,21.7450408809645,21.9911485751284),
 .UNSPECIFIED.);
#1368=B_SPLINE_CURVE_WITH_KNOTS('',3,(#57004,#57005,#57006,#57007,#57008,
#57009,#57010,#57011,#57012,#57013,#57014,#57015,#57016,#57017,#57018,#57019,
#57020,#57021,#57022,#57023,#57024,#57025,#57026,#57027,#57028,#57029,#57030,
#57031,#57032,#57033,#57034,#57035,#57036,#57037,#57038,#57039,#57040,#57041,
#57042,#57043,#57044,#57045,#57046,#57047,#57048,#57049,#57050,#57051,#57052,
#57053,#57054,#57055,#57056,#57057,#57058,#57059,#57060,#57061,#57062,#57063,
#57064,#57065,#57066,#57067,#57068,#57069,#57070,#57071,#57072,#57073,#57074,
#57075,#57076),.UNSPECIFIED.,.F.,.F.,(4,3,3,3,3,3,3,3,3,3,3,3,3,3,3,3,3,
3,3,3,3,3,3,3,4),(-1.5337369924875,-1.47677061263148,-1.38962639938855,
-1.35507536526616,-1.32724414064724,-1.22771895015351,-1.18711717053979,
-1.15068880045998,-1.12819375965977,-1.025630033795,-0.956371897287304,
-0.903212019653327,-0.873016070576496,-0.765510661060737,-0.671471231953964,
-0.617073852749348,-0.584769201911625,-0.476808850183147,-0.389352944633647,
-0.338455007564916,-0.310839780970012,-0.288641127038734,-0.179465062927756,
-0.0693975027893272,0.),.UNSPECIFIED.);
#1369=B_SPLINE_CURVE_WITH_KNOTS('',3,(#57081,#57082,#57083,#57084,#57085,
#57086,#57087,#57088,#57089,#57090,#57091,#57092,#57093,#57094,#57095,#57096,
#57097,#57098,#57099,#57100,#57101,#57102,#57103,#57104,#57105,#57106,#57107,
#57108,#57109,#57110,#57111,#57112,#57113,#57114,#57115,#57116,#57117,#57118,
#57119,#57120,#57121,#57122,#57123,#57124,#57125,#57126,#57127,#57128,#57129,
#57130,#57131,#57132,#57133,#57134,#57135,#57136,#57137,#57138,#57139,#57140,
#57141,#57142,#57143,#57144,#57145,#57146,#57147,#57148,#57149,#57150,#57151,
#57152,#57153,#57154,#57155,#57156),.UNSPECIFIED.,.F.,.F.,(4,3,3,3,3,3,
3,3,3,3,3,3,3,3,3,3,3,3,3,3,3,3,3,3,3,4),(-1.52870610664523,-1.46295898258929,
-1.36663193757431,-1.32703526012654,-1.2997044260243,-1.18867761427683,
-1.11943990274735,-1.09574005239823,-1.07765080252936,-0.970731016244023,
-0.864758172879583,-0.827864567613179,-0.806080610019377,-0.705048430139015,
-0.615223349572955,-0.566959037307119,-0.545377495328381,-0.521920092205195,
-0.420087461813239,-0.345748107874776,-0.297592979860876,-0.272101849578479,
-0.253166135873108,-0.153094666311387,-0.0548803280409424,0.),
 .UNSPECIFIED.);
#1370=B_SPLINE_CURVE_WITH_KNOTS('',3,(#58129,#58130,#58131,#58132,#58133,
#58134,#58135,#58136,#58137,#58138,#58139,#58140,#58141,#58142,#58143,#58144,
#58145,#58146,#58147,#58148,#58149,#58150),.UNSPECIFIED.,.F.,.F.,(4,3,3,
3,3,3,3,4),(114.220984235376,114.52221015029,115.020132803117,115.518055455945,
116.015978108772,116.513900761599,117.011823414427,117.426450205879),
 .UNSPECIFIED.);
#1371=B_SPLINE_CURVE_WITH_KNOTS('',3,(#58152,#58153,#58154,#58155,#58156,
#58157,#58158,#58159,#58160,#58161,#58162,#58163,#58164,#58165,#58166,#58167,
#58168,#58169,#58170,#58171,#58172,#58173,#58174,#58175,#58176,#58177,#58178,
#58179,#58180,#58181,#58182,#58183,#58184,#58185,#58186,#58187,#58188,#58189,
#58190,#58191,#58192,#58193,#58194,#58195,#58196,#58197,#58198,#58199,#58200,
#58201,#58202,#58203,#58204,#58205,#58206,#58207,#58208,#58209,#58210,#58211,
#58212,#58213,#58214,#58215,#58216,#58217,#58218,#58219,#58220,#58221,#58222,
#58223,#58224),.UNSPECIFIED.,.F.,.F.,(4,3,3,3,3,3,3,3,3,3,3,3,3,3,3,3,3,
3,3,3,3,3,3,3,4),(-1.53373699248749,-1.47677061263144,-1.38962639938852,
-1.35507537101752,-1.32724414240614,-1.22771895103294,-1.18711716909541,
-1.15068880119813,-1.12819375965975,-1.02563002916522,-0.95637190842141,
-0.903212033779905,-0.873016068995821,-0.765510661060749,-0.671471231953977,
-0.617073858764053,-0.584769201584582,-0.476808845396831,-0.389352944633662,
-0.338455004320312,-0.310839774199194,-0.288641121416588,-0.179465094293374,
-0.0693975125282933,0.),.UNSPECIFIED.);
#1372=B_SPLINE_CURVE_WITH_KNOTS('',3,(#58225,#58226,#58227,#58228,#58229,
#58230,#58231,#58232,#58233,#58234,#58235,#58236,#58237,#58238),
 .UNSPECIFIED.,.F.,.F.,(4,1,1,1,1,1,1,1,1,1,1,4),(10.3761157273101,10.7907425187629,
11.2886651715902,11.7865878244176,12.2845104772449,12.7824331300723,13.2803557828996,
13.778278435727,14.2762010885543,14.7741237413817,15.272046394209,15.7079632679489),
 .UNSPECIFIED.);
#1373=B_SPLINE_CURVE_WITH_KNOTS('',3,(#58244,#58245,#58246,#58247,#58248,
#58249,#58250,#58251,#58252,#58253,#58254,#58255,#58256,#58257,#58258,#58259,
#58260,#58261,#58262,#58263,#58264,#58265,#58266,#58267,#58268,#58269,#58270,
#58271,#58272,#58273,#58274,#58275,#58276,#58277,#58278,#58279,#58280,#58281,
#58282,#58283,#58284,#58285,#58286,#58287,#58288,#58289,#58290,#58291,#58292,
#58293,#58294,#58295,#58296,#58297,#58298,#58299,#58300,#58301,#58302,#58303,
#58304,#58305,#58306,#58307,#58308,#58309,#58310,#58311,#58312,#58313,#58314,
#58315,#58316,#58317,#58318,#58319),.UNSPECIFIED.,.F.,.F.,(4,3,3,3,3,3,
3,3,3,3,3,3,3,3,3,3,3,3,3,3,3,3,3,3,3,4),(-1.52870610664511,-1.46295898258918,
-1.36663193757421,-1.32703525676065,-1.29970441890487,-1.18867761071707,
-1.11943990050039,-1.09574005213221,-1.07765080252928,-0.970731019336594,
-0.864758197089689,-0.827864489400151,-0.806080595680503,-0.705048430138953,
-0.615223349572903,-0.566959036424461,-0.545377489997276,-0.521920089539238,
-0.420087427185088,-0.345748107874755,-0.297592967728844,-0.272101809436843,
-0.253166083083881,-0.153094612893034,-0.0548803342925537,0.),
 .UNSPECIFIED.);
#1374=B_SPLINE_CURVE_WITH_KNOTS('',3,(#58322,#58323,#58324,#58325,#58326,
#58327,#58328,#58329,#58330,#58331,#58332,#58333),.UNSPECIFIED.,.F.,.F.,
(4,1,1,1,1,1,1,1,1,4),(11.6150328478182,12.1129555006455,12.6108781534729,
13.1088008063002,13.6067234591276,14.1046461119549,14.6025687647823,15.1004914176096,
15.5984140704369,15.7079632679489),.UNSPECIFIED.);
#1375=B_SPLINE_CURVE_WITH_KNOTS('',3,(#59306,#59307,#59308,#59309,#59310,
#59311,#59312,#59313,#59314,#59315,#59316,#59317,#59318,#59319,#59320,#59321),
 .UNSPECIFIED.,.F.,.F.,(4,3,3,3,3,4),(-119.501436678563,-119.003514025736,
-118.505591372909,-118.007668720081,-117.509746067254,-117.190265949363),
 .UNSPECIFIED.);
#1877=PLANE('',#27731);
#1878=PLANE('',#27734);
#1879=PLANE('',#27739);
#1880=PLANE('',#27741);
#1881=PLANE('',#27743);
#1882=PLANE('',#27745);
#1883=PLANE('',#27747);
#1884=PLANE('',#27749);
#1885=PLANE('',#27759);
#1886=PLANE('',#27760);
#1887=PLANE('',#27761);
#1888=PLANE('',#27762);
#1889=PLANE('',#27763);
#1890=PLANE('',#27764);
#1891=PLANE('',#27765);
#1892=PLANE('',#27766);
#1893=PLANE('',#27767);
#1894=PLANE('',#27768);
#1895=PLANE('',#27769);
#1896=PLANE('',#27770);
#1897=PLANE('',#27771);
#1898=PLANE('',#27772);
#1899=PLANE('',#27773);
#1900=PLANE('',#27774);
#1901=PLANE('',#27775);
#1902=PLANE('',#27776);
#1903=PLANE('',#27777);
#1904=PLANE('',#27778);
#1905=PLANE('',#27779);
#1906=PLANE('',#27780);
#1907=PLANE('',#27781);
#1908=PLANE('',#27782);
#1909=PLANE('',#27783);
#1910=PLANE('',#27790);
#3024=FACE_OUTER_BOUND('',#4535,.T.);
#3025=FACE_OUTER_BOUND('',#4536,.T.);
#3026=FACE_OUTER_BOUND('',#4537,.T.);
#3027=FACE_OUTER_BOUND('',#4538,.T.);
#3028=FACE_OUTER_BOUND('',#4539,.T.);
#3029=FACE_OUTER_BOUND('',#4540,.T.);
#3030=FACE_OUTER_BOUND('',#4541,.T.);
#3031=FACE_OUTER_BOUND('',#4542,.T.);
#3032=FACE_OUTER_BOUND('',#4543,.T.);
#3033=FACE_OUTER_BOUND('',#4544,.T.);
#3034=FACE_OUTER_BOUND('',#4545,.T.);
#3035=FACE_OUTER_BOUND('',#4546,.T.);
#3036=FACE_OUTER_BOUND('',#4547,.T.);
#3037=FACE_OUTER_BOUND('',#4548,.T.);
#3038=FACE_OUTER_BOUND('',#4549,.T.);
#3039=FACE_OUTER_BOUND('',#4550,.T.);
#3040=FACE_OUTER_BOUND('',#4551,.T.);
#3041=FACE_OUTER_BOUND('',#4552,.T.);
#3042=FACE_OUTER_BOUND('',#4553,.T.);
#3043=FACE_OUTER_BOUND('',#4554,.T.);
#3044=FACE_OUTER_BOUND('',#4555,.T.);
#3045=FACE_OUTER_BOUND('',#4556,.T.);
#3046=FACE_OUTER_BOUND('',#4557,.T.);
#3047=FACE_OUTER_BOUND('',#4558,.T.);
#3048=FACE_OUTER_BOUND('',#4559,.T.);
#3049=FACE_OUTER_BOUND('',#4560,.T.);
#3050=FACE_OUTER_BOUND('',#4561,.T.);
#3051=FACE_OUTER_BOUND('',#4562,.T.);
#3052=FACE_OUTER_BOUND('',#4563,.T.);
#3053=FACE_OUTER_BOUND('',#4564,.T.);
#3054=FACE_OUTER_BOUND('',#4565,.T.);
#3055=FACE_OUTER_BOUND('',#4566,.T.);
#3056=FACE_OUTER_BOUND('',#4567,.T.);
#3057=FACE_OUTER_BOUND('',#4568,.T.);
#3058=FACE_OUTER_BOUND('',#4569,.T.);
#3059=FACE_OUTER_BOUND('',#4570,.T.);
#3060=FACE_OUTER_BOUND('',#4571,.T.);
#3061=FACE_OUTER_BOUND('',#4572,.T.);
#3062=FACE_OUTER_BOUND('',#4573,.T.);
#3063=FACE_OUTER_BOUND('',#4574,.T.);
#3064=FACE_OUTER_BOUND('',#4575,.T.);
#3065=FACE_OUTER_BOUND('',#4576,.T.);
#3066=FACE_OUTER_BOUND('',#4577,.T.);
#3067=FACE_OUTER_BOUND('',#4578,.T.);
#3068=FACE_OUTER_BOUND('',#4579,.T.);
#3069=FACE_OUTER_BOUND('',#4580,.T.);
#3070=FACE_OUTER_BOUND('',#4581,.T.);
#3071=FACE_OUTER_BOUND('',#4582,.T.);
#3072=FACE_OUTER_BOUND('',#4583,.T.);
#3073=FACE_OUTER_BOUND('',#4584,.T.);
#3074=FACE_OUTER_BOUND('',#4585,.T.);
#3075=FACE_OUTER_BOUND('',#4586,.T.);
#3076=FACE_OUTER_BOUND('',#4587,.T.);
#3077=FACE_OUTER_BOUND('',#4588,.T.);
#3078=FACE_OUTER_BOUND('',#4589,.T.);
#3079=FACE_OUTER_BOUND('',#4590,.T.);
#3080=FACE_OUTER_BOUND('',#4591,.T.);
#3081=FACE_OUTER_BOUND('',#4592,.T.);
#3082=FACE_OUTER_BOUND('',#4593,.T.);
#3083=FACE_OUTER_BOUND('',#4594,.T.);
#3084=FACE_OUTER_BOUND('',#4595,.T.);
#3085=FACE_OUTER_BOUND('',#4596,.T.);
#3086=FACE_OUTER_BOUND('',#4597,.T.);
#3087=FACE_OUTER_BOUND('',#4598,.T.);
#3088=FACE_OUTER_BOUND('',#4599,.T.);
#3089=FACE_OUTER_BOUND('',#4600,.T.);
#3090=FACE_OUTER_BOUND('',#4601,.T.);
#3091=FACE_OUTER_BOUND('',#4602,.T.);
#3092=FACE_OUTER_BOUND('',#4603,.T.);
#3093=FACE_OUTER_BOUND('',#4604,.T.);
#3094=FACE_OUTER_BOUND('',#4605,.T.);
#3095=FACE_OUTER_BOUND('',#4606,.T.);
#3096=FACE_OUTER_BOUND('',#4607,.T.);
#3097=FACE_OUTER_BOUND('',#4608,.T.);
#3098=FACE_OUTER_BOUND('',#4609,.T.);
#3099=FACE_OUTER_BOUND('',#4610,.T.);
#3100=FACE_OUTER_BOUND('',#4611,.T.);
#3101=FACE_OUTER_BOUND('',#4612,.T.);
#3102=FACE_OUTER_BOUND('',#4613,.T.);
#4535=EDGE_LOOP('',(#19856,#19857,#19858,#19859));
#4536=EDGE_LOOP('',(#19860,#19861,#19862,#19863));
#4537=EDGE_LOOP('',(#19864,#19865,#19866,#19867));
#4538=EDGE_LOOP('',(#19868,#19869,#19870,#19871));
#4539=EDGE_LOOP('',(#19872,#19873,#19874,#19875));
#4540=EDGE_LOOP('',(#19876,#19877,#19878,#19879));
#4541=EDGE_LOOP('',(#19880,#19881,#19882,#19883));
#4542=EDGE_LOOP('',(#19884,#19885,#19886,#19887));
#4543=EDGE_LOOP('',(#19888,#19889,#19890,#19891));
#4544=EDGE_LOOP('',(#19892,#19893,#19894,#19895));
#4545=EDGE_LOOP('',(#19896,#19897,#19898,#19899));
#4546=EDGE_LOOP('',(#19900,#19901,#19902,#19903));
#4547=EDGE_LOOP('',(#19904,#19905,#19906,#19907));
#4548=EDGE_LOOP('',(#19908,#19909,#19910,#19911));
#4549=EDGE_LOOP('',(#19912,#19913,#19914,#19915));
#4550=EDGE_LOOP('',(#19916,#19917,#19918,#19919));
#4551=EDGE_LOOP('',(#19920,#19921,#19922,#19923));
#4552=EDGE_LOOP('',(#19924,#19925,#19926,#19927));
#4553=EDGE_LOOP('',(#19928,#19929,#19930,#19931));
#4554=EDGE_LOOP('',(#19932,#19933,#19934));
#4555=EDGE_LOOP('',(#19935,#19936,#19937,#19938,#19939));
#4556=EDGE_LOOP('',(#19940,#19941,#19942,#19943));
#4557=EDGE_LOOP('',(#19944,#19945,#19946,#19947));
#4558=EDGE_LOOP('',(#19948,#19949,#19950,#19951));
#4559=EDGE_LOOP('',(#19952,#19953,#19954,#19955));
#4560=EDGE_LOOP('',(#19956,#19957,#19958,#19959));
#4561=EDGE_LOOP('',(#19960,#19961,#19962,#19963));
#4562=EDGE_LOOP('',(#19964,#19965,#19966,#19967));
#4563=EDGE_LOOP('',(#19968,#19969,#19970,#19971));
#4564=EDGE_LOOP('',(#19972,#19973,#19974,#19975));
#4565=EDGE_LOOP('',(#19976,#19977,#19978,#19979));
#4566=EDGE_LOOP('',(#19980,#19981,#19982,#19983));
#4567=EDGE_LOOP('',(#19984,#19985,#19986,#19987));
#4568=EDGE_LOOP('',(#19988,#19989,#19990,#19991));
#4569=EDGE_LOOP('',(#19992,#19993,#19994,#19995));
#4570=EDGE_LOOP('',(#19996,#19997,#19998,#19999));
#4571=EDGE_LOOP('',(#20000,#20001,#20002,#20003));
#4572=EDGE_LOOP('',(#20004,#20005,#20006,#20007));
#4573=EDGE_LOOP('',(#20008,#20009,#20010,#20011,#20012,#20013));
#4574=EDGE_LOOP('',(#20014,#20015,#20016,#20017,#20018,#20019,#20020,#20021,
#20022,#20023,#20024,#20025,#20026,#20027,#20028,#20029,#20030,#20031,#20032,
#20033,#20034,#20035,#20036,#20037,#20038,#20039,#20040,#20041,#20042,#20043,
#20044,#20045,#20046,#20047,#20048,#20049,#20050,#20051,#20052,#20053,#20054));
#4575=EDGE_LOOP('',(#20055,#20056,#20057,#20058,#20059));
#4576=EDGE_LOOP('',(#20060,#20061,#20062,#20063));
#4577=EDGE_LOOP('',(#20064,#20065,#20066,#20067,#20068,#20069,#20070,#20071,
#20072,#20073,#20074,#20075,#20076,#20077,#20078,#20079,#20080,#20081,#20082,
#20083,#20084,#20085,#20086,#20087,#20088,#20089,#20090,#20091,#20092,#20093,
#20094,#20095,#20096,#20097,#20098,#20099,#20100,#20101,#20102,#20103,#20104,
#20105));
#4578=EDGE_LOOP('',(#20106,#20107));
#4579=EDGE_LOOP('',(#20108,#20109));
#4580=EDGE_LOOP('',(#20110,#20111));
#4581=EDGE_LOOP('',(#20112,#20113));
#4582=EDGE_LOOP('',(#20114,#20115));
#4583=EDGE_LOOP('',(#20116,#20117));
#4584=EDGE_LOOP('',(#20118,#20119,#20120,#20121,#20122,#20123,#20124,#20125,
#20126,#20127,#20128,#20129,#20130,#20131,#20132,#20133,#20134,#20135,#20136,
#20137,#20138,#20139,#20140,#20141,#20142,#20143,#20144));
#4585=EDGE_LOOP('',(#20145,#20146,#20147,#20148));
#4586=EDGE_LOOP('',(#20149,#20150,#20151));
#4587=EDGE_LOOP('',(#20152,#20153,#20154,#20155));
#4588=EDGE_LOOP('',(#20156,#20157,#20158));
#4589=EDGE_LOOP('',(#20159,#20160,#20161));
#4590=EDGE_LOOP('',(#20162,#20163,#20164,#20165));
#4591=EDGE_LOOP('',(#20166,#20167,#20168));
#4592=EDGE_LOOP('',(#20169,#20170,#20171,#20172));
#4593=EDGE_LOOP('',(#20173,#20174,#20175));
#4594=EDGE_LOOP('',(#20176,#20177,#20178));
#4595=EDGE_LOOP('',(#20179,#20180,#20181));
#4596=EDGE_LOOP('',(#20182,#20183,#20184));
#4597=EDGE_LOOP('',(#20185,#20186,#20187));
#4598=EDGE_LOOP('',(#20188,#20189,#20190));
#4599=EDGE_LOOP('',(#20191,#20192,#20193));
#4600=EDGE_LOOP('',(#20194,#20195,#20196,#20197));
#4601=EDGE_LOOP('',(#20198,#20199,#20200,#20201));
#4602=EDGE_LOOP('',(#20202,#20203,#20204));
#4603=EDGE_LOOP('',(#20205,#20206,#20207));
#4604=EDGE_LOOP('',(#20208,#20209,#20210));
#4605=EDGE_LOOP('',(#20211,#20212,#20213,#20214));
#4606=EDGE_LOOP('',(#20215,#20216,#20217));
#4607=EDGE_LOOP('',(#20218,#20219,#20220));
#4608=EDGE_LOOP('',(#20221,#20222,#20223));
#4609=EDGE_LOOP('',(#20224));
#4610=EDGE_LOOP('',(#20225,#20226,#20227,#20228,#20229,#20230));
#4611=EDGE_LOOP('',(#20231,#20232,#20233,#20234));
#4612=EDGE_LOOP('',(#20235,#20236,#20237,#20238,#20239,#20240));
#4613=EDGE_LOOP('',(#20241));
#4614=EDGE_LOOP('',(#20242,#20243,#20244,#20245,#20246,#20247));
#6157=LINE('',#54714,#8654);
#6158=LINE('',#54747,#8655);
#6159=LINE('',#54831,#8656);
#6160=LINE('',#54921,#8657);
#6161=LINE('',#55011,#8658);
#6162=LINE('',#55095,#8659);
#6163=LINE('',#55185,#8660);
#6164=LINE('',#55269,#8661);
#6165=LINE('',#55359,#8662);
#6166=LINE('',#55449,#8663);
#6167=LINE('',#55533,#8664);
#6168=LINE('',#55623,#8665);
#6169=LINE('',#55713,#8666);
#6170=LINE('',#55797,#8667);
#6171=LINE('',#55887,#8668);
#6172=LINE('',#55971,#8669);
#6173=LINE('',#56061,#8670);
#6174=LINE('',#56151,#8671);
#6175=LINE('',#56235,#8672);
#6176=LINE('',#56325,#8673);
#6177=LINE('',#56335,#8674);
#6178=LINE('',#56372,#8675);
#6179=LINE('',#56409,#8676);
#6180=LINE('',#56446,#8677);
#6181=LINE('',#56484,#8678);
#6182=LINE('',#56521,#8679);
#6183=LINE('',#56558,#8680);
#6184=LINE('',#56595,#8681);
#6185=LINE('',#56632,#8682);
#6186=LINE('',#56670,#8683);
#6187=LINE('',#56707,#8684);
#6188=LINE('',#56744,#8685);
#6189=LINE('',#56782,#8686);
#6190=LINE('',#56819,#8687);
#6191=LINE('',#56856,#8688);
#6192=LINE('',#56893,#8689);
#6193=LINE('',#56930,#8690);
#6194=LINE('',#56968,#8691);
#6195=LINE('',#59325,#8692);
#6196=LINE('',#59329,#8693);
#6197=LINE('',#59333,#8694);
#6198=LINE('',#59337,#8695);
#6199=LINE('',#59341,#8696);
#6200=LINE('',#59344,#8697);
#6201=LINE('',#59349,#8698);
#6202=LINE('',#59407,#8699);
#6203=LINE('',#59409,#8700);
#6204=LINE('',#59410,#8701);
#6205=LINE('',#59413,#8702);
#6206=LINE('',#59414,#8703);
#6207=LINE('',#59417,#8704);
#6208=LINE('',#59418,#8705);
#6209=LINE('',#59421,#8706);
#6210=LINE('',#59422,#8707);
#6211=LINE('',#59425,#8708);
#6212=LINE('',#59426,#8709);
#6213=LINE('',#59429,#8710);
#6214=LINE('',#59430,#8711);
#6215=LINE('',#59433,#8712);
#6216=LINE('',#59434,#8713);
#6217=LINE('',#59437,#8714);
#6218=LINE('',#59438,#8715);
#6219=LINE('',#59441,#8716);
#6220=LINE('',#59442,#8717);
#6221=LINE('',#59444,#8718);
#6222=LINE('',#59446,#8719);
#6223=LINE('',#59449,#8720);
#6224=LINE('',#59452,#8721);
#6225=LINE('',#59453,#8722);
#6226=LINE('',#59455,#8723);
#6227=LINE('',#59457,#8724);
#6228=LINE('',#59460,#8725);
#6229=LINE('',#59461,#8726);
#6230=LINE('',#59463,#8727);
#6231=LINE('',#59467,#8728);
#6232=LINE('',#59475,#8729);
#6233=LINE('',#59481,#8730);
#8654=VECTOR('',#30788,0.8);
#8655=VECTOR('',#30793,0.8);
#8656=VECTOR('',#30796,0.8);
#8657=VECTOR('',#30799,0.8);
#8658=VECTOR('',#30802,0.8);
#8659=VECTOR('',#30805,0.8);
#8660=VECTOR('',#30808,0.8);
#8661=VECTOR('',#30811,0.8);
#8662=VECTOR('',#30814,0.8);
#8663=VECTOR('',#30817,0.8);
#8664=VECTOR('',#30820,0.8);
#8665=VECTOR('',#30823,0.8);
#8666=VECTOR('',#30826,0.8);
#8667=VECTOR('',#30829,0.8);
#8668=VECTOR('',#30832,0.8);
#8669=VECTOR('',#30835,0.8);
#8670=VECTOR('',#30838,0.8);
#8671=VECTOR('',#30841,0.8);
#8672=VECTOR('',#30844,0.8);
#8673=VECTOR('',#30847,0.6767);
#8674=VECTOR('',#30852,0.6767);
#8675=VECTOR('',#30857,0.6767);
#8676=VECTOR('',#30860,0.6767);
#8677=VECTOR('',#30863,0.6767);
#8678=VECTOR('',#30866,0.6767);
#8679=VECTOR('',#30869,0.6767);
#8680=VECTOR('',#30872,0.6767);
#8681=VECTOR('',#30875,0.6767);
#8682=VECTOR('',#30878,0.6767);
#8683=VECTOR('',#30881,0.6767);
#8684=VECTOR('',#30884,0.6767);
#8685=VECTOR('',#30887,0.6767);
#8686=VECTOR('',#30890,0.6767);
#8687=VECTOR('',#30893,0.6767);
#8688=VECTOR('',#30896,0.6767);
#8689=VECTOR('',#30899,0.6767);
#8690=VECTOR('',#30902,0.6767);
#8691=VECTOR('',#30905,0.6767);
#8692=VECTOR('',#30924,1.);
#8693=VECTOR('',#30929,1.);
#8694=VECTOR('',#30934,1.);
#8695=VECTOR('',#30939,1.);
#8696=VECTOR('',#30944,1.);
#8697=VECTOR('',#30949,1.);
#8698=VECTOR('',#30954,0.23094010767585);
#8699=VECTOR('',#30971,1.);
#8700=VECTOR('',#30972,1.);
#8701=VECTOR('',#30973,1.);
#8702=VECTOR('',#30976,1.);
#8703=VECTOR('',#30977,1.);
#8704=VECTOR('',#30980,1.);
#8705=VECTOR('',#30981,1.);
#8706=VECTOR('',#30984,1.);
#8707=VECTOR('',#30985,1.);
#8708=VECTOR('',#30988,1.);
#8709=VECTOR('',#30989,1.);
#8710=VECTOR('',#30992,1.);
#8711=VECTOR('',#30993,1.);
#8712=VECTOR('',#30996,1.);
#8713=VECTOR('',#30997,1.);
#8714=VECTOR('',#31000,1.);
#8715=VECTOR('',#31001,1.);
#8716=VECTOR('',#31004,1.);
#8717=VECTOR('',#31005,1.);
#8718=VECTOR('',#31008,1.);
#8719=VECTOR('',#31011,1.);
#8720=VECTOR('',#31016,1.);
#8721=VECTOR('',#31019,1.);
#8722=VECTOR('',#31020,1.);
#8723=VECTOR('',#31023,1.);
#8724=VECTOR('',#31026,1.);
#8725=VECTOR('',#31029,1.);
#8726=VECTOR('',#31030,1.);
#8727=VECTOR('',#31033,1.);
#8728=VECTOR('',#31040,1.);
#8729=VECTOR('',#31053,0.7);
#8730=VECTOR('',#31062,0.76);
#10840=CIRCLE('',#27691,0.7911);
#10841=CIRCLE('',#27711,0.6767);
#10842=CIRCLE('',#27713,0.6767);
#10843=CIRCLE('',#27732,0.7911);
#10844=CIRCLE('',#27733,0.7911);
#10845=CIRCLE('',#27735,0.7911);
#10846=CIRCLE('',#27736,0.7911);
#10847=CIRCLE('',#27737,0.6767);
#10848=CIRCLE('',#27740,0.461880215351701);
#10849=CIRCLE('',#27742,0.461880215351701);
#10850=CIRCLE('',#27744,0.461880215351701);
#10851=CIRCLE('',#27746,0.461880215351701);
#10852=CIRCLE('',#27748,0.461880215351701);
#10853=CIRCLE('',#27750,0.461880215351701);
#10854=CIRCLE('',#27752,0.460219541126976);
#10855=CIRCLE('',#27753,0.460219541126976);
#10856=CIRCLE('',#27754,0.460219541126976);
#10857=CIRCLE('',#27755,0.460219541126976);
#10858=CIRCLE('',#27756,0.460219541126976);
#10859=CIRCLE('',#27757,0.460219541126976);
#10860=CIRCLE('',#27758,0.460219541126976);
#10861=CIRCLE('',#27784,0.6);
#10862=CIRCLE('',#27787,0.7911);
#10863=CIRCLE('',#27789,0.72);
#11884=VERTEX_POINT('',#54712);
#11885=VERTEX_POINT('',#54713);
#11886=VERTEX_POINT('',#54715);
#11887=VERTEX_POINT('',#54732);
#11888=VERTEX_POINT('',#54745);
#11889=VERTEX_POINT('',#54746);
#11890=VERTEX_POINT('',#54829);
#11891=VERTEX_POINT('',#54830);
#11892=VERTEX_POINT('',#54919);
#11893=VERTEX_POINT('',#54920);
#11894=VERTEX_POINT('',#55009);
#11895=VERTEX_POINT('',#55010);
#11896=VERTEX_POINT('',#55093);
#11897=VERTEX_POINT('',#55094);
#11898=VERTEX_POINT('',#55183);
#11899=VERTEX_POINT('',#55184);
#11900=VERTEX_POINT('',#55267);
#11901=VERTEX_POINT('',#55268);
#11902=VERTEX_POINT('',#55357);
#11903=VERTEX_POINT('',#55358);
#11904=VERTEX_POINT('',#55447);
#11905=VERTEX_POINT('',#55448);
#11906=VERTEX_POINT('',#55531);
#11907=VERTEX_POINT('',#55532);
#11908=VERTEX_POINT('',#55621);
#11909=VERTEX_POINT('',#55622);
#11910=VERTEX_POINT('',#55711);
#11911=VERTEX_POINT('',#55712);
#11912=VERTEX_POINT('',#55795);
#11913=VERTEX_POINT('',#55796);
#11914=VERTEX_POINT('',#55885);
#11915=VERTEX_POINT('',#55886);
#11916=VERTEX_POINT('',#55969);
#11917=VERTEX_POINT('',#55970);
#11918=VERTEX_POINT('',#56059);
#11919=VERTEX_POINT('',#56060);
#11920=VERTEX_POINT('',#56149);
#11921=VERTEX_POINT('',#56150);
#11922=VERTEX_POINT('',#56233);
#11923=VERTEX_POINT('',#56234);
#11924=VERTEX_POINT('',#56323);
#11925=VERTEX_POINT('',#56324);
#11926=VERTEX_POINT('',#56326);
#11927=VERTEX_POINT('',#56333);
#11928=VERTEX_POINT('',#56334);
#11929=VERTEX_POINT('',#56353);
#11930=VERTEX_POINT('',#56370);
#11931=VERTEX_POINT('',#56371);
#11932=VERTEX_POINT('',#56407);
#11933=VERTEX_POINT('',#56408);
#11934=VERTEX_POINT('',#56444);
#11935=VERTEX_POINT('',#56445);
#11936=VERTEX_POINT('',#56482);
#11937=VERTEX_POINT('',#56483);
#11938=VERTEX_POINT('',#56519);
#11939=VERTEX_POINT('',#56520);
#11940=VERTEX_POINT('',#56556);
#11941=VERTEX_POINT('',#56557);
#11942=VERTEX_POINT('',#56593);
#11943=VERTEX_POINT('',#56594);
#11944=VERTEX_POINT('',#56630);
#11945=VERTEX_POINT('',#56631);
#11946=VERTEX_POINT('',#56668);
#11947=VERTEX_POINT('',#56669);
#11948=VERTEX_POINT('',#56705);
#11949=VERTEX_POINT('',#56706);
#11950=VERTEX_POINT('',#56742);
#11951=VERTEX_POINT('',#56743);
#11952=VERTEX_POINT('',#56780);
#11953=VERTEX_POINT('',#56781);
#11954=VERTEX_POINT('',#56817);
#11955=VERTEX_POINT('',#56818);
#11956=VERTEX_POINT('',#56854);
#11957=VERTEX_POINT('',#56855);
#11958=VERTEX_POINT('',#56891);
#11959=VERTEX_POINT('',#56892);
#11960=VERTEX_POINT('',#56928);
#11961=VERTEX_POINT('',#56929);
#11962=VERTEX_POINT('',#56966);
#11963=VERTEX_POINT('',#56967);
#11964=VERTEX_POINT('',#57003);
#11965=VERTEX_POINT('',#57077);
#11966=VERTEX_POINT('',#57079);
#11967=VERTEX_POINT('',#58151);
#11968=VERTEX_POINT('',#58240);
#11969=VERTEX_POINT('',#58243);
#11970=VERTEX_POINT('',#59323);
#11971=VERTEX_POINT('',#59324);
#11972=VERTEX_POINT('',#59328);
#11973=VERTEX_POINT('',#59332);
#11974=VERTEX_POINT('',#59336);
#11975=VERTEX_POINT('',#59340);
#11976=VERTEX_POINT('',#59347);
#11977=VERTEX_POINT('',#59348);
#11978=VERTEX_POINT('',#59350);
#11979=VERTEX_POINT('',#59355);
#11980=VERTEX_POINT('',#59359);
#11981=VERTEX_POINT('',#59364);
#11982=VERTEX_POINT('',#59368);
#11983=VERTEX_POINT('',#59373);
#11984=VERTEX_POINT('',#59377);
#11985=VERTEX_POINT('',#59382);
#11986=VERTEX_POINT('',#59386);
#11987=VERTEX_POINT('',#59391);
#11988=VERTEX_POINT('',#59395);
#11989=VERTEX_POINT('',#59400);
#11990=VERTEX_POINT('',#59406);
#11991=VERTEX_POINT('',#59408);
#11992=VERTEX_POINT('',#59412);
#11993=VERTEX_POINT('',#59416);
#11994=VERTEX_POINT('',#59420);
#11995=VERTEX_POINT('',#59424);
#11996=VERTEX_POINT('',#59428);
#11997=VERTEX_POINT('',#59432);
#11998=VERTEX_POINT('',#59436);
#11999=VERTEX_POINT('',#59440);
#12000=VERTEX_POINT('',#59451);
#12001=VERTEX_POINT('',#59459);
#12002=VERTEX_POINT('',#59472);
#12003=VERTEX_POINT('',#59479);
#14781=EDGE_CURVE('',#11884,#11885,#6157,.T.);
#14782=EDGE_CURVE('',#11884,#11886,#1293,.T.);
#14783=EDGE_CURVE('',#11886,#11887,#10840,.T.);
#14784=EDGE_CURVE('',#11887,#11885,#1294,.T.);
#14785=EDGE_CURVE('',#11888,#11889,#6158,.T.);
#14786=EDGE_CURVE('',#11888,#11884,#1295,.T.);
#14787=EDGE_CURVE('',#11885,#11889,#1296,.T.);
#14788=EDGE_CURVE('',#11890,#11891,#6159,.T.);
#14789=EDGE_CURVE('',#11890,#11888,#1297,.T.);
#14790=EDGE_CURVE('',#11889,#11891,#1298,.T.);
#14791=EDGE_CURVE('',#11892,#11893,#6160,.T.);
#14792=EDGE_CURVE('',#11892,#11890,#1299,.T.);
#14793=EDGE_CURVE('',#11891,#11893,#1300,.T.);
#14794=EDGE_CURVE('',#11894,#11895,#6161,.T.);
#14795=EDGE_CURVE('',#11894,#11892,#1301,.T.);
#14796=EDGE_CURVE('',#11893,#11895,#1302,.T.);
#14797=EDGE_CURVE('',#11896,#11897,#6162,.T.);
#14798=EDGE_CURVE('',#11896,#11894,#1303,.T.);
#14799=EDGE_CURVE('',#11895,#11897,#1304,.T.);
#14800=EDGE_CURVE('',#11898,#11899,#6163,.T.);
#14801=EDGE_CURVE('',#11898,#11896,#1305,.T.);
#14802=EDGE_CURVE('',#11897,#11899,#1306,.T.);
#14803=EDGE_CURVE('',#11900,#11901,#6164,.T.);
#14804=EDGE_CURVE('',#11900,#11898,#1307,.T.);
#14805=EDGE_CURVE('',#11899,#11901,#1308,.T.);
#14806=EDGE_CURVE('',#11902,#11903,#6165,.T.);
#14807=EDGE_CURVE('',#11902,#11900,#1309,.T.);
#14808=EDGE_CURVE('',#11901,#11903,#1310,.T.);
#14809=EDGE_CURVE('',#11904,#11905,#6166,.T.);
#14810=EDGE_CURVE('',#11904,#11902,#1311,.T.);
#14811=EDGE_CURVE('',#11903,#11905,#1312,.T.);
#14812=EDGE_CURVE('',#11906,#11907,#6167,.T.);
#14813=EDGE_CURVE('',#11906,#11904,#1313,.T.);
#14814=EDGE_CURVE('',#11905,#11907,#1314,.T.);
#14815=EDGE_CURVE('',#11908,#11909,#6168,.T.);
#14816=EDGE_CURVE('',#11908,#11906,#1315,.T.);
#14817=EDGE_CURVE('',#11907,#11909,#1316,.T.);
#14818=EDGE_CURVE('',#11910,#11911,#6169,.T.);
#14819=EDGE_CURVE('',#11910,#11908,#1317,.T.);
#14820=EDGE_CURVE('',#11909,#11911,#1318,.T.);
#14821=EDGE_CURVE('',#11912,#11913,#6170,.T.);
#14822=EDGE_CURVE('',#11912,#11910,#1319,.T.);
#14823=EDGE_CURVE('',#11911,#11913,#1320,.T.);
#14824=EDGE_CURVE('',#11914,#11915,#6171,.T.);
#14825=EDGE_CURVE('',#11914,#11912,#1321,.T.);
#14826=EDGE_CURVE('',#11913,#11915,#1322,.T.);
#14827=EDGE_CURVE('',#11916,#11917,#6172,.T.);
#14828=EDGE_CURVE('',#11916,#11914,#1323,.T.);
#14829=EDGE_CURVE('',#11915,#11917,#1324,.T.);
#14830=EDGE_CURVE('',#11918,#11919,#6173,.T.);
#14831=EDGE_CURVE('',#11918,#11916,#1325,.T.);
#14832=EDGE_CURVE('',#11917,#11919,#1326,.T.);
#14833=EDGE_CURVE('',#11920,#11921,#6174,.T.);
#14834=EDGE_CURVE('',#11920,#11918,#1327,.T.);
#14835=EDGE_CURVE('',#11919,#11921,#1328,.T.);
#14836=EDGE_CURVE('',#11922,#11923,#6175,.T.);
#14837=EDGE_CURVE('',#11922,#11920,#1329,.T.);
#14838=EDGE_CURVE('',#11921,#11923,#1330,.T.);
#14839=EDGE_CURVE('',#11924,#11925,#6176,.T.);
#14840=EDGE_CURVE('',#11924,#11926,#1331,.T.);
#14841=EDGE_CURVE('',#11925,#11926,#10841,.T.);
#14842=EDGE_CURVE('',#11927,#11928,#6177,.T.);
#14843=EDGE_CURVE('',#11927,#11924,#1332,.T.);
#14844=EDGE_CURVE('',#11929,#11925,#10842,.T.);
#14845=EDGE_CURVE('',#11928,#11929,#1333,.T.);
#14846=EDGE_CURVE('',#11930,#11931,#6178,.T.);
#14847=EDGE_CURVE('',#11930,#11927,#1334,.T.);
#14848=EDGE_CURVE('',#11931,#11928,#1335,.T.);
#14849=EDGE_CURVE('',#11932,#11933,#6179,.T.);
#14850=EDGE_CURVE('',#11932,#11930,#1336,.T.);
#14851=EDGE_CURVE('',#11933,#11931,#1337,.T.);
#14852=EDGE_CURVE('',#11934,#11935,#6180,.T.);
#14853=EDGE_CURVE('',#11934,#11932,#1338,.T.);
#14854=EDGE_CURVE('',#11935,#11933,#1339,.T.);
#14855=EDGE_CURVE('',#11936,#11937,#6181,.T.);
#14856=EDGE_CURVE('',#11936,#11934,#1340,.T.);
#14857=EDGE_CURVE('',#11937,#11935,#1341,.T.);
#14858=EDGE_CURVE('',#11938,#11939,#6182,.T.);
#14859=EDGE_CURVE('',#11938,#11936,#1342,.T.);
#14860=EDGE_CURVE('',#11939,#11937,#1343,.T.);
#14861=EDGE_CURVE('',#11940,#11941,#6183,.T.);
#14862=EDGE_CURVE('',#11940,#11938,#1344,.T.);
#14863=EDGE_CURVE('',#11941,#11939,#1345,.T.);
#14864=EDGE_CURVE('',#11942,#11943,#6184,.T.);
#14865=EDGE_CURVE('',#11942,#11940,#1346,.T.);
#14866=EDGE_CURVE('',#11943,#11941,#1347,.T.);
#14867=EDGE_CURVE('',#11944,#11945,#6185,.T.);
#14868=EDGE_CURVE('',#11944,#11942,#1348,.T.);
#14869=EDGE_CURVE('',#11945,#11943,#1349,.T.);
#14870=EDGE_CURVE('',#11946,#11947,#6186,.T.);
#14871=EDGE_CURVE('',#11946,#11944,#1350,.T.);
#14872=EDGE_CURVE('',#11947,#11945,#1351,.T.);
#14873=EDGE_CURVE('',#11948,#11949,#6187,.T.);
#14874=EDGE_CURVE('',#11948,#11946,#1352,.T.);
#14875=EDGE_CURVE('',#11949,#11947,#1353,.T.);
#14876=EDGE_CURVE('',#11950,#11951,#6188,.T.);
#14877=EDGE_CURVE('',#11950,#11948,#1354,.T.);
#14878=EDGE_CURVE('',#11951,#11949,#1355,.T.);
#14879=EDGE_CURVE('',#11952,#11953,#6189,.T.);
#14880=EDGE_CURVE('',#11952,#11950,#1356,.T.);
#14881=EDGE_CURVE('',#11953,#11951,#1357,.T.);
#14882=EDGE_CURVE('',#11954,#11955,#6190,.T.);
#14883=EDGE_CURVE('',#11954,#11952,#1358,.T.);
#14884=EDGE_CURVE('',#11955,#11953,#1359,.T.);
#14885=EDGE_CURVE('',#11956,#11957,#6191,.T.);
#14886=EDGE_CURVE('',#11956,#11954,#1360,.T.);
#14887=EDGE_CURVE('',#11957,#11955,#1361,.T.);
#14888=EDGE_CURVE('',#11958,#11959,#6192,.T.);
#14889=EDGE_CURVE('',#11958,#11956,#1362,.T.);
#14890=EDGE_CURVE('',#11959,#11957,#1363,.T.);
#14891=EDGE_CURVE('',#11960,#11961,#6193,.T.);
#14892=EDGE_CURVE('',#11960,#11958,#1364,.T.);
#14893=EDGE_CURVE('',#11961,#11959,#1365,.T.);
#14894=EDGE_CURVE('',#11962,#11963,#6194,.T.);
#14895=EDGE_CURVE('',#11962,#11960,#1366,.T.);
#14896=EDGE_CURVE('',#11963,#11961,#1367,.T.);
#14897=EDGE_CURVE('',#11926,#11964,#1368,.T.);
#14898=EDGE_CURVE('',#11965,#11964,#10843,.F.);
#14899=EDGE_CURVE('',#11966,#11965,#10844,.F.);
#14900=EDGE_CURVE('',#11966,#11929,#1369,.T.);
#14901=EDGE_CURVE('',#11923,#11966,#1370,.T.);
#14902=EDGE_CURVE('',#11967,#11887,#1371,.T.);
#14903=EDGE_CURVE('',#11967,#11963,#1372,.T.);
#14904=EDGE_CURVE('',#11887,#11968,#10845,.T.);
#14905=EDGE_CURVE('',#11968,#11886,#10846,.T.);
#14906=EDGE_CURVE('',#11886,#11969,#1373,.T.);
#14907=EDGE_CURVE('',#11969,#11967,#10847,.T.);
#14908=EDGE_CURVE('',#11969,#11962,#1374,.T.);
#14909=EDGE_CURVE('',#11964,#11922,#1375,.T.);
#14910=EDGE_CURVE('',#11970,#11971,#6195,.T.);
#14911=EDGE_CURVE('',#11971,#11970,#10848,.T.);
#14912=EDGE_CURVE('',#11971,#11972,#6196,.T.);
#14913=EDGE_CURVE('',#11972,#11971,#10849,.T.);
#14914=EDGE_CURVE('',#11972,#11973,#6197,.T.);
#14915=EDGE_CURVE('',#11973,#11972,#10850,.T.);
#14916=EDGE_CURVE('',#11973,#11974,#6198,.T.);
#14917=EDGE_CURVE('',#11974,#11973,#10851,.T.);
#14918=EDGE_CURVE('',#11974,#11975,#6199,.T.);
#14919=EDGE_CURVE('',#11975,#11974,#10852,.T.);
#14920=EDGE_CURVE('',#11975,#11970,#6200,.T.);
#14921=EDGE_CURVE('',#11970,#11975,#10853,.T.);
#14922=EDGE_CURVE('',#11976,#11977,#6201,.T.);
#14923=EDGE_CURVE('',#11978,#11977,#10854,.T.);
#14924=EDGE_CURVE('',#11972,#11978,#241,.T.);
#14925=EDGE_CURVE('',#11979,#11971,#242,.T.);
#14926=EDGE_CURVE('',#11980,#11979,#10855,.T.);
#14927=EDGE_CURVE('',#11971,#11980,#243,.T.);
#14928=EDGE_CURVE('',#11981,#11970,#244,.T.);
#14929=EDGE_CURVE('',#11982,#11981,#10856,.T.);
#14930=EDGE_CURVE('',#11970,#11982,#245,.T.);
#14931=EDGE_CURVE('',#11983,#11975,#246,.T.);
#14932=EDGE_CURVE('',#11984,#11983,#10857,.T.);
#14933=EDGE_CURVE('',#11975,#11984,#247,.T.);
#14934=EDGE_CURVE('',#11985,#11974,#248,.T.);
#14935=EDGE_CURVE('',#11986,#11985,#10858,.T.);
#14936=EDGE_CURVE('',#11974,#11986,#249,.T.);
#14937=EDGE_CURVE('',#11987,#11973,#250,.T.);
#14938=EDGE_CURVE('',#11988,#11987,#10859,.T.);
#14939=EDGE_CURVE('',#11973,#11988,#251,.T.);
#14940=EDGE_CURVE('',#11989,#11972,#252,.T.);
#14941=EDGE_CURVE('',#11977,#11989,#10860,.T.);
#14942=EDGE_CURVE('',#11990,#11973,#6202,.T.);
#14943=EDGE_CURVE('',#11991,#11990,#6203,.T.);
#14944=EDGE_CURVE('',#11991,#11972,#6204,.T.);
#14945=EDGE_CURVE('',#11972,#11992,#6205,.T.);
#14946=EDGE_CURVE('',#11992,#11989,#6206,.T.);
#14947=EDGE_CURVE('',#11993,#11974,#6207,.T.);
#14948=EDGE_CURVE('',#11990,#11993,#6208,.T.);
#14949=EDGE_CURVE('',#11986,#11994,#6209,.T.);
#14950=EDGE_CURVE('',#11974,#11994,#6210,.T.);
#14951=EDGE_CURVE('',#11973,#11995,#6211,.T.);
#14952=EDGE_CURVE('',#11995,#11987,#6212,.T.);
#14953=EDGE_CURVE('',#11996,#11991,#6213,.T.);
#14954=EDGE_CURVE('',#11996,#11971,#6214,.T.);
#14955=EDGE_CURVE('',#11971,#11997,#6215,.T.);
#14956=EDGE_CURVE('',#11997,#11979,#6216,.T.);
#14957=EDGE_CURVE('',#11998,#11975,#6217,.T.);
#14958=EDGE_CURVE('',#11993,#11998,#6218,.T.);
#14959=EDGE_CURVE('',#11984,#11999,#6219,.T.);
#14960=EDGE_CURVE('',#11975,#11999,#6220,.T.);
#14961=EDGE_CURVE('',#11994,#11985,#6221,.T.);
#14962=EDGE_CURVE('',#11988,#11995,#6222,.T.);
#14963=EDGE_CURVE('',#11999,#11983,#6223,.T.);
#14964=EDGE_CURVE('',#12000,#11981,#6224,.T.);
#14965=EDGE_CURVE('',#11982,#12000,#6225,.T.);
#14966=EDGE_CURVE('',#11980,#11997,#6226,.T.);
#14967=EDGE_CURVE('',#11978,#11992,#6227,.T.);
#14968=EDGE_CURVE('',#12001,#11970,#6228,.T.);
#14969=EDGE_CURVE('',#11998,#12001,#6229,.T.);
#14970=EDGE_CURVE('',#11970,#12000,#6230,.T.);
#14971=EDGE_CURVE('',#12001,#11996,#6231,.T.);
#14972=EDGE_CURVE('',#12002,#12002,#10861,.T.);
#14973=EDGE_CURVE('',#11968,#12002,#6232,.T.);
#14974=EDGE_CURVE('',#11964,#11966,#10862,.F.);
#14975=EDGE_CURVE('',#12003,#12003,#10863,.T.);
#14976=EDGE_CURVE('',#12003,#11965,#6233,.T.);
#19856=ORIENTED_EDGE('',*,*,#14781,.F.);
#19857=ORIENTED_EDGE('',*,*,#14782,.T.);
#19858=ORIENTED_EDGE('',*,*,#14783,.T.);
#19859=ORIENTED_EDGE('',*,*,#14784,.T.);
#19860=ORIENTED_EDGE('',*,*,#14785,.F.);
#19861=ORIENTED_EDGE('',*,*,#14786,.T.);
#19862=ORIENTED_EDGE('',*,*,#14781,.T.);
#19863=ORIENTED_EDGE('',*,*,#14787,.T.);
#19864=ORIENTED_EDGE('',*,*,#14788,.F.);
#19865=ORIENTED_EDGE('',*,*,#14789,.T.);
#19866=ORIENTED_EDGE('',*,*,#14785,.T.);
#19867=ORIENTED_EDGE('',*,*,#14790,.T.);
#19868=ORIENTED_EDGE('',*,*,#14791,.F.);
#19869=ORIENTED_EDGE('',*,*,#14792,.T.);
#19870=ORIENTED_EDGE('',*,*,#14788,.T.);
#19871=ORIENTED_EDGE('',*,*,#14793,.T.);
#19872=ORIENTED_EDGE('',*,*,#14794,.F.);
#19873=ORIENTED_EDGE('',*,*,#14795,.T.);
#19874=ORIENTED_EDGE('',*,*,#14791,.T.);
#19875=ORIENTED_EDGE('',*,*,#14796,.T.);
#19876=ORIENTED_EDGE('',*,*,#14797,.F.);
#19877=ORIENTED_EDGE('',*,*,#14798,.T.);
#19878=ORIENTED_EDGE('',*,*,#14794,.T.);
#19879=ORIENTED_EDGE('',*,*,#14799,.T.);
#19880=ORIENTED_EDGE('',*,*,#14800,.F.);
#19881=ORIENTED_EDGE('',*,*,#14801,.T.);
#19882=ORIENTED_EDGE('',*,*,#14797,.T.);
#19883=ORIENTED_EDGE('',*,*,#14802,.T.);
#19884=ORIENTED_EDGE('',*,*,#14803,.F.);
#19885=ORIENTED_EDGE('',*,*,#14804,.T.);
#19886=ORIENTED_EDGE('',*,*,#14800,.T.);
#19887=ORIENTED_EDGE('',*,*,#14805,.T.);
#19888=ORIENTED_EDGE('',*,*,#14806,.F.);
#19889=ORIENTED_EDGE('',*,*,#14807,.T.);
#19890=ORIENTED_EDGE('',*,*,#14803,.T.);
#19891=ORIENTED_EDGE('',*,*,#14808,.T.);
#19892=ORIENTED_EDGE('',*,*,#14809,.F.);
#19893=ORIENTED_EDGE('',*,*,#14810,.T.);
#19894=ORIENTED_EDGE('',*,*,#14806,.T.);
#19895=ORIENTED_EDGE('',*,*,#14811,.T.);
#19896=ORIENTED_EDGE('',*,*,#14812,.F.);
#19897=ORIENTED_EDGE('',*,*,#14813,.T.);
#19898=ORIENTED_EDGE('',*,*,#14809,.T.);
#19899=ORIENTED_EDGE('',*,*,#14814,.T.);
#19900=ORIENTED_EDGE('',*,*,#14815,.F.);
#19901=ORIENTED_EDGE('',*,*,#14816,.T.);
#19902=ORIENTED_EDGE('',*,*,#14812,.T.);
#19903=ORIENTED_EDGE('',*,*,#14817,.T.);
#19904=ORIENTED_EDGE('',*,*,#14818,.F.);
#19905=ORIENTED_EDGE('',*,*,#14819,.T.);
#19906=ORIENTED_EDGE('',*,*,#14815,.T.);
#19907=ORIENTED_EDGE('',*,*,#14820,.T.);
#19908=ORIENTED_EDGE('',*,*,#14821,.F.);
#19909=ORIENTED_EDGE('',*,*,#14822,.T.);
#19910=ORIENTED_EDGE('',*,*,#14818,.T.);
#19911=ORIENTED_EDGE('',*,*,#14823,.T.);
#19912=ORIENTED_EDGE('',*,*,#14824,.F.);
#19913=ORIENTED_EDGE('',*,*,#14825,.T.);
#19914=ORIENTED_EDGE('',*,*,#14821,.T.);
#19915=ORIENTED_EDGE('',*,*,#14826,.T.);
#19916=ORIENTED_EDGE('',*,*,#14827,.F.);
#19917=ORIENTED_EDGE('',*,*,#14828,.T.);
#19918=ORIENTED_EDGE('',*,*,#14824,.T.);
#19919=ORIENTED_EDGE('',*,*,#14829,.T.);
#19920=ORIENTED_EDGE('',*,*,#14830,.F.);
#19921=ORIENTED_EDGE('',*,*,#14831,.T.);
#19922=ORIENTED_EDGE('',*,*,#14827,.T.);
#19923=ORIENTED_EDGE('',*,*,#14832,.T.);
#19924=ORIENTED_EDGE('',*,*,#14833,.F.);
#19925=ORIENTED_EDGE('',*,*,#14834,.T.);
#19926=ORIENTED_EDGE('',*,*,#14830,.T.);
#19927=ORIENTED_EDGE('',*,*,#14835,.T.);
#19928=ORIENTED_EDGE('',*,*,#14836,.F.);
#19929=ORIENTED_EDGE('',*,*,#14837,.T.);
#19930=ORIENTED_EDGE('',*,*,#14833,.T.);
#19931=ORIENTED_EDGE('',*,*,#14838,.T.);
#19932=ORIENTED_EDGE('',*,*,#14839,.F.);
#19933=ORIENTED_EDGE('',*,*,#14840,.T.);
#19934=ORIENTED_EDGE('',*,*,#14841,.F.);
#19935=ORIENTED_EDGE('',*,*,#14842,.F.);
#19936=ORIENTED_EDGE('',*,*,#14843,.T.);
#19937=ORIENTED_EDGE('',*,*,#14839,.T.);
#19938=ORIENTED_EDGE('',*,*,#14844,.F.);
#19939=ORIENTED_EDGE('',*,*,#14845,.F.);
#19940=ORIENTED_EDGE('',*,*,#14846,.F.);
#19941=ORIENTED_EDGE('',*,*,#14847,.T.);
#19942=ORIENTED_EDGE('',*,*,#14842,.T.);
#19943=ORIENTED_EDGE('',*,*,#14848,.F.);
#19944=ORIENTED_EDGE('',*,*,#14849,.F.);
#19945=ORIENTED_EDGE('',*,*,#14850,.T.);
#19946=ORIENTED_EDGE('',*,*,#14846,.T.);
#19947=ORIENTED_EDGE('',*,*,#14851,.F.);
#19948=ORIENTED_EDGE('',*,*,#14852,.F.);
#19949=ORIENTED_EDGE('',*,*,#14853,.T.);
#19950=ORIENTED_EDGE('',*,*,#14849,.T.);
#19951=ORIENTED_EDGE('',*,*,#14854,.F.);
#19952=ORIENTED_EDGE('',*,*,#14855,.F.);
#19953=ORIENTED_EDGE('',*,*,#14856,.T.);
#19954=ORIENTED_EDGE('',*,*,#14852,.T.);
#19955=ORIENTED_EDGE('',*,*,#14857,.F.);
#19956=ORIENTED_EDGE('',*,*,#14858,.F.);
#19957=ORIENTED_EDGE('',*,*,#14859,.T.);
#19958=ORIENTED_EDGE('',*,*,#14855,.T.);
#19959=ORIENTED_EDGE('',*,*,#14860,.F.);
#19960=ORIENTED_EDGE('',*,*,#14861,.F.);
#19961=ORIENTED_EDGE('',*,*,#14862,.T.);
#19962=ORIENTED_EDGE('',*,*,#14858,.T.);
#19963=ORIENTED_EDGE('',*,*,#14863,.F.);
#19964=ORIENTED_EDGE('',*,*,#14864,.F.);
#19965=ORIENTED_EDGE('',*,*,#14865,.T.);
#19966=ORIENTED_EDGE('',*,*,#14861,.T.);
#19967=ORIENTED_EDGE('',*,*,#14866,.F.);
#19968=ORIENTED_EDGE('',*,*,#14867,.F.);
#19969=ORIENTED_EDGE('',*,*,#14868,.T.);
#19970=ORIENTED_EDGE('',*,*,#14864,.T.);
#19971=ORIENTED_EDGE('',*,*,#14869,.F.);
#19972=ORIENTED_EDGE('',*,*,#14870,.F.);
#19973=ORIENTED_EDGE('',*,*,#14871,.T.);
#19974=ORIENTED_EDGE('',*,*,#14867,.T.);
#19975=ORIENTED_EDGE('',*,*,#14872,.F.);
#19976=ORIENTED_EDGE('',*,*,#14873,.F.);
#19977=ORIENTED_EDGE('',*,*,#14874,.T.);
#19978=ORIENTED_EDGE('',*,*,#14870,.T.);
#19979=ORIENTED_EDGE('',*,*,#14875,.F.);
#19980=ORIENTED_EDGE('',*,*,#14876,.F.);
#19981=ORIENTED_EDGE('',*,*,#14877,.T.);
#19982=ORIENTED_EDGE('',*,*,#14873,.T.);
#19983=ORIENTED_EDGE('',*,*,#14878,.F.);
#19984=ORIENTED_EDGE('',*,*,#14879,.F.);
#19985=ORIENTED_EDGE('',*,*,#14880,.T.);
#19986=ORIENTED_EDGE('',*,*,#14876,.T.);
#19987=ORIENTED_EDGE('',*,*,#14881,.F.);
#19988=ORIENTED_EDGE('',*,*,#14882,.F.);
#19989=ORIENTED_EDGE('',*,*,#14883,.T.);
#19990=ORIENTED_EDGE('',*,*,#14879,.T.);
#19991=ORIENTED_EDGE('',*,*,#14884,.F.);
#19992=ORIENTED_EDGE('',*,*,#14885,.F.);
#19993=ORIENTED_EDGE('',*,*,#14886,.T.);
#19994=ORIENTED_EDGE('',*,*,#14882,.T.);
#19995=ORIENTED_EDGE('',*,*,#14887,.F.);
#19996=ORIENTED_EDGE('',*,*,#14888,.F.);
#19997=ORIENTED_EDGE('',*,*,#14889,.T.);
#19998=ORIENTED_EDGE('',*,*,#14885,.T.);
#19999=ORIENTED_EDGE('',*,*,#14890,.F.);
#20000=ORIENTED_EDGE('',*,*,#14891,.F.);
#20001=ORIENTED_EDGE('',*,*,#14892,.T.);
#20002=ORIENTED_EDGE('',*,*,#14888,.T.);
#20003=ORIENTED_EDGE('',*,*,#14893,.F.);
#20004=ORIENTED_EDGE('',*,*,#14894,.F.);
#20005=ORIENTED_EDGE('',*,*,#14895,.T.);
#20006=ORIENTED_EDGE('',*,*,#14891,.T.);
#20007=ORIENTED_EDGE('',*,*,#14896,.F.);
#20008=ORIENTED_EDGE('',*,*,#14844,.T.);
#20009=ORIENTED_EDGE('',*,*,#14841,.T.);
#20010=ORIENTED_EDGE('',*,*,#14897,.T.);
#20011=ORIENTED_EDGE('',*,*,#14898,.F.);
#20012=ORIENTED_EDGE('',*,*,#14899,.F.);
#20013=ORIENTED_EDGE('',*,*,#14900,.T.);
#20014=ORIENTED_EDGE('',*,*,#14900,.F.);
#20015=ORIENTED_EDGE('',*,*,#14901,.F.);
#20016=ORIENTED_EDGE('',*,*,#14838,.F.);
#20017=ORIENTED_EDGE('',*,*,#14835,.F.);
#20018=ORIENTED_EDGE('',*,*,#14832,.F.);
#20019=ORIENTED_EDGE('',*,*,#14829,.F.);
#20020=ORIENTED_EDGE('',*,*,#14826,.F.);
#20021=ORIENTED_EDGE('',*,*,#14823,.F.);
#20022=ORIENTED_EDGE('',*,*,#14820,.F.);
#20023=ORIENTED_EDGE('',*,*,#14817,.F.);
#20024=ORIENTED_EDGE('',*,*,#14814,.F.);
#20025=ORIENTED_EDGE('',*,*,#14811,.F.);
#20026=ORIENTED_EDGE('',*,*,#14808,.F.);
#20027=ORIENTED_EDGE('',*,*,#14805,.F.);
#20028=ORIENTED_EDGE('',*,*,#14802,.F.);
#20029=ORIENTED_EDGE('',*,*,#14799,.F.);
#20030=ORIENTED_EDGE('',*,*,#14796,.F.);
#20031=ORIENTED_EDGE('',*,*,#14793,.F.);
#20032=ORIENTED_EDGE('',*,*,#14790,.F.);
#20033=ORIENTED_EDGE('',*,*,#14787,.F.);
#20034=ORIENTED_EDGE('',*,*,#14784,.F.);
#20035=ORIENTED_EDGE('',*,*,#14902,.F.);
#20036=ORIENTED_EDGE('',*,*,#14903,.T.);
#20037=ORIENTED_EDGE('',*,*,#14896,.T.);
#20038=ORIENTED_EDGE('',*,*,#14893,.T.);
#20039=ORIENTED_EDGE('',*,*,#14890,.T.);
#20040=ORIENTED_EDGE('',*,*,#14887,.T.);
#20041=ORIENTED_EDGE('',*,*,#14884,.T.);
#20042=ORIENTED_EDGE('',*,*,#14881,.T.);
#20043=ORIENTED_EDGE('',*,*,#14878,.T.);
#20044=ORIENTED_EDGE('',*,*,#14875,.T.);
#20045=ORIENTED_EDGE('',*,*,#14872,.T.);
#20046=ORIENTED_EDGE('',*,*,#14869,.T.);
#20047=ORIENTED_EDGE('',*,*,#14866,.T.);
#20048=ORIENTED_EDGE('',*,*,#14863,.T.);
#20049=ORIENTED_EDGE('',*,*,#14860,.T.);
#20050=ORIENTED_EDGE('',*,*,#14857,.T.);
#20051=ORIENTED_EDGE('',*,*,#14854,.T.);
#20052=ORIENTED_EDGE('',*,*,#14851,.T.);
#20053=ORIENTED_EDGE('',*,*,#14848,.T.);
#20054=ORIENTED_EDGE('',*,*,#14845,.T.);
#20055=ORIENTED_EDGE('',*,*,#14904,.T.);
#20056=ORIENTED_EDGE('',*,*,#14905,.T.);
#20057=ORIENTED_EDGE('',*,*,#14906,.T.);
#20058=ORIENTED_EDGE('',*,*,#14907,.T.);
#20059=ORIENTED_EDGE('',*,*,#14902,.T.);
#20060=ORIENTED_EDGE('',*,*,#14894,.T.);
#20061=ORIENTED_EDGE('',*,*,#14903,.F.);
#20062=ORIENTED_EDGE('',*,*,#14907,.F.);
#20063=ORIENTED_EDGE('',*,*,#14908,.T.);
#20064=ORIENTED_EDGE('',*,*,#14897,.F.);
#20065=ORIENTED_EDGE('',*,*,#14840,.F.);
#20066=ORIENTED_EDGE('',*,*,#14843,.F.);
#20067=ORIENTED_EDGE('',*,*,#14847,.F.);
#20068=ORIENTED_EDGE('',*,*,#14850,.F.);
#20069=ORIENTED_EDGE('',*,*,#14853,.F.);
#20070=ORIENTED_EDGE('',*,*,#14856,.F.);
#20071=ORIENTED_EDGE('',*,*,#14859,.F.);
#20072=ORIENTED_EDGE('',*,*,#14862,.F.);
#20073=ORIENTED_EDGE('',*,*,#14865,.F.);
#20074=ORIENTED_EDGE('',*,*,#14868,.F.);
#20075=ORIENTED_EDGE('',*,*,#14871,.F.);
#20076=ORIENTED_EDGE('',*,*,#14874,.F.);
#20077=ORIENTED_EDGE('',*,*,#14877,.F.);
#20078=ORIENTED_EDGE('',*,*,#14880,.F.);
#20079=ORIENTED_EDGE('',*,*,#14883,.F.);
#20080=ORIENTED_EDGE('',*,*,#14886,.F.);
#20081=ORIENTED_EDGE('',*,*,#14889,.F.);
#20082=ORIENTED_EDGE('',*,*,#14892,.F.);
#20083=ORIENTED_EDGE('',*,*,#14895,.F.);
#20084=ORIENTED_EDGE('',*,*,#14908,.F.);
#20085=ORIENTED_EDGE('',*,*,#14906,.F.);
#20086=ORIENTED_EDGE('',*,*,#14782,.F.);
#20087=ORIENTED_EDGE('',*,*,#14786,.F.);
#20088=ORIENTED_EDGE('',*,*,#14789,.F.);
#20089=ORIENTED_EDGE('',*,*,#14792,.F.);
#20090=ORIENTED_EDGE('',*,*,#14795,.F.);
#20091=ORIENTED_EDGE('',*,*,#14798,.F.);
#20092=ORIENTED_EDGE('',*,*,#14801,.F.);
#20093=ORIENTED_EDGE('',*,*,#14804,.F.);
#20094=ORIENTED_EDGE('',*,*,#14807,.F.);
#20095=ORIENTED_EDGE('',*,*,#14810,.F.);
#20096=ORIENTED_EDGE('',*,*,#14813,.F.);
#20097=ORIENTED_EDGE('',*,*,#14816,.F.);
#20098=ORIENTED_EDGE('',*,*,#14819,.F.);
#20099=ORIENTED_EDGE('',*,*,#14822,.F.);
#20100=ORIENTED_EDGE('',*,*,#14825,.F.);
#20101=ORIENTED_EDGE('',*,*,#14828,.F.);
#20102=ORIENTED_EDGE('',*,*,#14831,.F.);
#20103=ORIENTED_EDGE('',*,*,#14834,.F.);
#20104=ORIENTED_EDGE('',*,*,#14837,.F.);
#20105=ORIENTED_EDGE('',*,*,#14909,.F.);
#20106=ORIENTED_EDGE('',*,*,#14910,.F.);
#20107=ORIENTED_EDGE('',*,*,#14911,.F.);
#20108=ORIENTED_EDGE('',*,*,#14912,.F.);
#20109=ORIENTED_EDGE('',*,*,#14913,.F.);
#20110=ORIENTED_EDGE('',*,*,#14914,.F.);
#20111=ORIENTED_EDGE('',*,*,#14915,.F.);
#20112=ORIENTED_EDGE('',*,*,#14916,.F.);
#20113=ORIENTED_EDGE('',*,*,#14917,.F.);
#20114=ORIENTED_EDGE('',*,*,#14918,.F.);
#20115=ORIENTED_EDGE('',*,*,#14919,.F.);
#20116=ORIENTED_EDGE('',*,*,#14920,.F.);
#20117=ORIENTED_EDGE('',*,*,#14921,.F.);
#20118=ORIENTED_EDGE('',*,*,#14922,.T.);
#20119=ORIENTED_EDGE('',*,*,#14923,.F.);
#20120=ORIENTED_EDGE('',*,*,#14924,.F.);
#20121=ORIENTED_EDGE('',*,*,#14913,.T.);
#20122=ORIENTED_EDGE('',*,*,#14925,.F.);
#20123=ORIENTED_EDGE('',*,*,#14926,.F.);
#20124=ORIENTED_EDGE('',*,*,#14927,.F.);
#20125=ORIENTED_EDGE('',*,*,#14911,.T.);
#20126=ORIENTED_EDGE('',*,*,#14928,.F.);
#20127=ORIENTED_EDGE('',*,*,#14929,.F.);
#20128=ORIENTED_EDGE('',*,*,#14930,.F.);
#20129=ORIENTED_EDGE('',*,*,#14921,.T.);
#20130=ORIENTED_EDGE('',*,*,#14931,.F.);
#20131=ORIENTED_EDGE('',*,*,#14932,.F.);
#20132=ORIENTED_EDGE('',*,*,#14933,.F.);
#20133=ORIENTED_EDGE('',*,*,#14919,.T.);
#20134=ORIENTED_EDGE('',*,*,#14934,.F.);
#20135=ORIENTED_EDGE('',*,*,#14935,.F.);
#20136=ORIENTED_EDGE('',*,*,#14936,.F.);
#20137=ORIENTED_EDGE('',*,*,#14917,.T.);
#20138=ORIENTED_EDGE('',*,*,#14937,.F.);
#20139=ORIENTED_EDGE('',*,*,#14938,.F.);
#20140=ORIENTED_EDGE('',*,*,#14939,.F.);
#20141=ORIENTED_EDGE('',*,*,#14915,.T.);
#20142=ORIENTED_EDGE('',*,*,#14940,.F.);
#20143=ORIENTED_EDGE('',*,*,#14941,.F.);
#20144=ORIENTED_EDGE('',*,*,#14922,.F.);
#20145=ORIENTED_EDGE('',*,*,#14914,.T.);
#20146=ORIENTED_EDGE('',*,*,#14942,.F.);
#20147=ORIENTED_EDGE('',*,*,#14943,.F.);
#20148=ORIENTED_EDGE('',*,*,#14944,.T.);
#20149=ORIENTED_EDGE('',*,*,#14940,.T.);
#20150=ORIENTED_EDGE('',*,*,#14945,.T.);
#20151=ORIENTED_EDGE('',*,*,#14946,.T.);
#20152=ORIENTED_EDGE('',*,*,#14916,.T.);
#20153=ORIENTED_EDGE('',*,*,#14947,.F.);
#20154=ORIENTED_EDGE('',*,*,#14948,.F.);
#20155=ORIENTED_EDGE('',*,*,#14942,.T.);
#20156=ORIENTED_EDGE('',*,*,#14936,.T.);
#20157=ORIENTED_EDGE('',*,*,#14949,.T.);
#20158=ORIENTED_EDGE('',*,*,#14950,.F.);
#20159=ORIENTED_EDGE('',*,*,#14937,.T.);
#20160=ORIENTED_EDGE('',*,*,#14951,.T.);
#20161=ORIENTED_EDGE('',*,*,#14952,.T.);
#20162=ORIENTED_EDGE('',*,*,#14912,.T.);
#20163=ORIENTED_EDGE('',*,*,#14944,.F.);
#20164=ORIENTED_EDGE('',*,*,#14953,.F.);
#20165=ORIENTED_EDGE('',*,*,#14954,.T.);
#20166=ORIENTED_EDGE('',*,*,#14925,.T.);
#20167=ORIENTED_EDGE('',*,*,#14955,.T.);
#20168=ORIENTED_EDGE('',*,*,#14956,.T.);
#20169=ORIENTED_EDGE('',*,*,#14918,.T.);
#20170=ORIENTED_EDGE('',*,*,#14957,.F.);
#20171=ORIENTED_EDGE('',*,*,#14958,.F.);
#20172=ORIENTED_EDGE('',*,*,#14947,.T.);
#20173=ORIENTED_EDGE('',*,*,#14933,.T.);
#20174=ORIENTED_EDGE('',*,*,#14959,.T.);
#20175=ORIENTED_EDGE('',*,*,#14960,.F.);
#20176=ORIENTED_EDGE('',*,*,#14934,.T.);
#20177=ORIENTED_EDGE('',*,*,#14950,.T.);
#20178=ORIENTED_EDGE('',*,*,#14961,.T.);
#20179=ORIENTED_EDGE('',*,*,#14938,.T.);
#20180=ORIENTED_EDGE('',*,*,#14952,.F.);
#20181=ORIENTED_EDGE('',*,*,#14962,.F.);
#20182=ORIENTED_EDGE('',*,*,#14935,.T.);
#20183=ORIENTED_EDGE('',*,*,#14961,.F.);
#20184=ORIENTED_EDGE('',*,*,#14949,.F.);
#20185=ORIENTED_EDGE('',*,*,#14932,.T.);
#20186=ORIENTED_EDGE('',*,*,#14963,.F.);
#20187=ORIENTED_EDGE('',*,*,#14959,.F.);
#20188=ORIENTED_EDGE('',*,*,#14929,.T.);
#20189=ORIENTED_EDGE('',*,*,#14964,.F.);
#20190=ORIENTED_EDGE('',*,*,#14965,.F.);
#20191=ORIENTED_EDGE('',*,*,#14926,.T.);
#20192=ORIENTED_EDGE('',*,*,#14956,.F.);
#20193=ORIENTED_EDGE('',*,*,#14966,.F.);
#20194=ORIENTED_EDGE('',*,*,#14923,.T.);
#20195=ORIENTED_EDGE('',*,*,#14941,.T.);
#20196=ORIENTED_EDGE('',*,*,#14946,.F.);
#20197=ORIENTED_EDGE('',*,*,#14967,.F.);
#20198=ORIENTED_EDGE('',*,*,#14920,.T.);
#20199=ORIENTED_EDGE('',*,*,#14968,.F.);
#20200=ORIENTED_EDGE('',*,*,#14969,.F.);
#20201=ORIENTED_EDGE('',*,*,#14957,.T.);
#20202=ORIENTED_EDGE('',*,*,#14930,.T.);
#20203=ORIENTED_EDGE('',*,*,#14965,.T.);
#20204=ORIENTED_EDGE('',*,*,#14970,.F.);
#20205=ORIENTED_EDGE('',*,*,#14931,.T.);
#20206=ORIENTED_EDGE('',*,*,#14960,.T.);
#20207=ORIENTED_EDGE('',*,*,#14963,.T.);
#20208=ORIENTED_EDGE('',*,*,#14928,.T.);
#20209=ORIENTED_EDGE('',*,*,#14970,.T.);
#20210=ORIENTED_EDGE('',*,*,#14964,.T.);
#20211=ORIENTED_EDGE('',*,*,#14910,.T.);
#20212=ORIENTED_EDGE('',*,*,#14954,.F.);
#20213=ORIENTED_EDGE('',*,*,#14971,.F.);
#20214=ORIENTED_EDGE('',*,*,#14968,.T.);
#20215=ORIENTED_EDGE('',*,*,#14939,.T.);
#20216=ORIENTED_EDGE('',*,*,#14962,.T.);
#20217=ORIENTED_EDGE('',*,*,#14951,.F.);
#20218=ORIENTED_EDGE('',*,*,#14924,.T.);
#20219=ORIENTED_EDGE('',*,*,#14967,.T.);
#20220=ORIENTED_EDGE('',*,*,#14945,.F.);
#20221=ORIENTED_EDGE('',*,*,#14927,.T.);
#20222=ORIENTED_EDGE('',*,*,#14966,.T.);
#20223=ORIENTED_EDGE('',*,*,#14955,.F.);
#20224=ORIENTED_EDGE('',*,*,#14972,.F.);
#20225=ORIENTED_EDGE('',*,*,#14904,.F.);
#20226=ORIENTED_EDGE('',*,*,#14783,.F.);
#20227=ORIENTED_EDGE('',*,*,#14905,.F.);
#20228=ORIENTED_EDGE('',*,*,#14973,.T.);
#20229=ORIENTED_EDGE('',*,*,#14972,.T.);
#20230=ORIENTED_EDGE('',*,*,#14973,.F.);
#20231=ORIENTED_EDGE('',*,*,#14836,.T.);
#20232=ORIENTED_EDGE('',*,*,#14901,.T.);
#20233=ORIENTED_EDGE('',*,*,#14974,.F.);
#20234=ORIENTED_EDGE('',*,*,#14909,.T.);
#20235=ORIENTED_EDGE('',*,*,#14975,.F.);
#20236=ORIENTED_EDGE('',*,*,#14976,.T.);
#20237=ORIENTED_EDGE('',*,*,#14898,.T.);
#20238=ORIENTED_EDGE('',*,*,#14974,.T.);
#20239=ORIENTED_EDGE('',*,*,#14899,.T.);
#20240=ORIENTED_EDGE('',*,*,#14976,.F.);
#20241=ORIENTED_EDGE('',*,*,#14975,.T.);
#20242=ORIENTED_EDGE('',*,*,#14958,.T.);
#20243=ORIENTED_EDGE('',*,*,#14969,.T.);
#20244=ORIENTED_EDGE('',*,*,#14971,.T.);
#20245=ORIENTED_EDGE('',*,*,#14953,.T.);
#20246=ORIENTED_EDGE('',*,*,#14943,.T.);
#20247=ORIENTED_EDGE('',*,*,#14948,.T.);
#25337=CONICAL_SURFACE('',#27751,0.23094010767585,1.02878638855047);
#25338=CONICAL_SURFACE('',#27785,0.7,0.785398163397448);
#25339=CONICAL_SURFACE('',#27788,0.76,0.785398163397449);
#25837=ADVANCED_FACE('',(#3024),#683,.T.);
#25838=ADVANCED_FACE('',(#3025),#684,.T.);
#25839=ADVANCED_FACE('',(#3026),#685,.T.);
#25840=ADVANCED_FACE('',(#3027),#686,.T.);
#25841=ADVANCED_FACE('',(#3028),#687,.T.);
#25842=ADVANCED_FACE('',(#3029),#688,.T.);
#25843=ADVANCED_FACE('',(#3030),#689,.T.);
#25844=ADVANCED_FACE('',(#3031),#690,.T.);
#25845=ADVANCED_FACE('',(#3032),#691,.T.);
#25846=ADVANCED_FACE('',(#3033),#692,.T.);
#25847=ADVANCED_FACE('',(#3034),#693,.T.);
#25848=ADVANCED_FACE('',(#3035),#694,.T.);
#25849=ADVANCED_FACE('',(#3036),#695,.T.);
#25850=ADVANCED_FACE('',(#3037),#696,.T.);
#25851=ADVANCED_FACE('',(#3038),#697,.T.);
#25852=ADVANCED_FACE('',(#3039),#698,.T.);
#25853=ADVANCED_FACE('',(#3040),#699,.T.);
#25854=ADVANCED_FACE('',(#3041),#700,.T.);
#25855=ADVANCED_FACE('',(#3042),#701,.T.);
#25856=ADVANCED_FACE('',(#3043),#702,.T.);
#25857=ADVANCED_FACE('',(#3044),#703,.T.);
#25858=ADVANCED_FACE('',(#3045),#704,.T.);
#25859=ADVANCED_FACE('',(#3046),#705,.T.);
#25860=ADVANCED_FACE('',(#3047),#706,.T.);
#25861=ADVANCED_FACE('',(#3048),#707,.T.);
#25862=ADVANCED_FACE('',(#3049),#708,.T.);
#25863=ADVANCED_FACE('',(#3050),#709,.T.);
#25864=ADVANCED_FACE('',(#3051),#710,.T.);
#25865=ADVANCED_FACE('',(#3052),#711,.T.);
#25866=ADVANCED_FACE('',(#3053),#712,.T.);
#25867=ADVANCED_FACE('',(#3054),#713,.T.);
#25868=ADVANCED_FACE('',(#3055),#714,.T.);
#25869=ADVANCED_FACE('',(#3056),#715,.T.);
#25870=ADVANCED_FACE('',(#3057),#716,.T.);
#25871=ADVANCED_FACE('',(#3058),#717,.T.);
#25872=ADVANCED_FACE('',(#3059),#718,.T.);
#25873=ADVANCED_FACE('',(#3060),#719,.T.);
#25874=ADVANCED_FACE('',(#3061),#720,.T.);
#25875=ADVANCED_FACE('',(#3062),#1877,.F.);
#25876=ADVANCED_FACE('',(#3063),#278,.F.);
#25877=ADVANCED_FACE('',(#3064),#1878,.T.);
#25878=ADVANCED_FACE('',(#3065),#721,.T.);
#25879=ADVANCED_FACE('',(#3066),#279,.F.);
#25880=ADVANCED_FACE('',(#3067),#1879,.F.);
#25881=ADVANCED_FACE('',(#3068),#1880,.F.);
#25882=ADVANCED_FACE('',(#3069),#1881,.F.);
#25883=ADVANCED_FACE('',(#3070),#1882,.F.);
#25884=ADVANCED_FACE('',(#3071),#1883,.F.);
#25885=ADVANCED_FACE('',(#3072),#1884,.F.);
#25886=ADVANCED_FACE('',(#3073),#25337,.F.);
#25887=ADVANCED_FACE('',(#3074),#1885,.F.);
#25888=ADVANCED_FACE('',(#3075),#1886,.F.);
#25889=ADVANCED_FACE('',(#3076),#1887,.F.);
#25890=ADVANCED_FACE('',(#3077),#1888,.F.);
#25891=ADVANCED_FACE('',(#3078),#1889,.F.);
#25892=ADVANCED_FACE('',(#3079),#1890,.F.);
#25893=ADVANCED_FACE('',(#3080),#1891,.F.);
#25894=ADVANCED_FACE('',(#3081),#1892,.F.);
#25895=ADVANCED_FACE('',(#3082),#1893,.F.);
#25896=ADVANCED_FACE('',(#3083),#1894,.F.);
#25897=ADVANCED_FACE('',(#3084),#1895,.F.);
#25898=ADVANCED_FACE('',(#3085),#1896,.F.);
#25899=ADVANCED_FACE('',(#3086),#1897,.F.);
#25900=ADVANCED_FACE('',(#3087),#1898,.F.);
#25901=ADVANCED_FACE('',(#3088),#1899,.F.);
#25902=ADVANCED_FACE('',(#3089),#1900,.F.);
#25903=ADVANCED_FACE('',(#3090),#1901,.F.);
#25904=ADVANCED_FACE('',(#3091),#1902,.F.);
#25905=ADVANCED_FACE('',(#3092),#1903,.F.);
#25906=ADVANCED_FACE('',(#3093),#1904,.F.);
#25907=ADVANCED_FACE('',(#3094),#1905,.F.);
#25908=ADVANCED_FACE('',(#3095),#1906,.F.);
#25909=ADVANCED_FACE('',(#3096),#1907,.F.);
#25910=ADVANCED_FACE('',(#3097),#1908,.F.);
#25911=ADVANCED_FACE('',(#3098),#1909,.T.);
#25912=ADVANCED_FACE('',(#3099),#25338,.T.);
#25913=ADVANCED_FACE('',(#3100),#722,.T.);
#25914=ADVANCED_FACE('',(#3101),#25339,.T.);
#25915=ADVANCED_FACE('',(#3102,#867),#1910,.T.);
#26881=CLOSED_SHELL('',(#25837,#25838,#25839,#25840,#25841,#25842,#25843,
#25844,#25845,#25846,#25847,#25848,#25849,#25850,#25851,#25852,#25853,#25854,
#25855,#25856,#25857,#25858,#25859,#25860,#25861,#25862,#25863,#25864,#25865,
#25866,#25867,#25868,#25869,#25870,#25871,#25872,#25873,#25874,#25875,#25876,
#25877,#25878,#25879,#25880,#25881,#25882,#25883,#25884,#25885,#25886,#25887,
#25888,#25889,#25890,#25891,#25892,#25893,#25894,#25895,#25896,#25897,#25898,
#25899,#25900,#25901,#25902,#25903,#25904,#25905,#25906,#25907,#25908,#25909,
#25910,#25911,#25912,#25913,#25914,#25915));
#27689=AXIS2_PLACEMENT_3D('',#54710,#30784,#30785);
#27690=AXIS2_PLACEMENT_3D('',#54711,#30786,#30787);
#27691=AXIS2_PLACEMENT_3D('',#54733,#30789,#30790);
#27692=AXIS2_PLACEMENT_3D('',#54744,#30791,#30792);
#27693=AXIS2_PLACEMENT_3D('',#54828,#30794,#30795);
#27694=AXIS2_PLACEMENT_3D('',#54918,#30797,#30798);
#27695=AXIS2_PLACEMENT_3D('',#55008,#30800,#30801);
#27696=AXIS2_PLACEMENT_3D('',#55092,#30803,#30804);
#27697=AXIS2_PLACEMENT_3D('',#55182,#30806,#30807);
#27698=AXIS2_PLACEMENT_3D('',#55266,#30809,#30810);
#27699=AXIS2_PLACEMENT_3D('',#55356,#30812,#30813);
#27700=AXIS2_PLACEMENT_3D('',#55446,#30815,#30816);
#27701=AXIS2_PLACEMENT_3D('',#55530,#30818,#30819);
#27702=AXIS2_PLACEMENT_3D('',#55620,#30821,#30822);
#27703=AXIS2_PLACEMENT_3D('',#55710,#30824,#30825);
#27704=AXIS2_PLACEMENT_3D('',#55794,#30827,#30828);
#27705=AXIS2_PLACEMENT_3D('',#55884,#30830,#30831);
#27706=AXIS2_PLACEMENT_3D('',#55968,#30833,#30834);
#27707=AXIS2_PLACEMENT_3D('',#56058,#30836,#30837);
#27708=AXIS2_PLACEMENT_3D('',#56148,#30839,#30840);
#27709=AXIS2_PLACEMENT_3D('',#56232,#30842,#30843);
#27710=AXIS2_PLACEMENT_3D('',#56322,#30845,#30846);
#27711=AXIS2_PLACEMENT_3D('',#56331,#30848,#30849);
#27712=AXIS2_PLACEMENT_3D('',#56332,#30850,#30851);
#27713=AXIS2_PLACEMENT_3D('',#56354,#30853,#30854);
#27714=AXIS2_PLACEMENT_3D('',#56369,#30855,#30856);
#27715=AXIS2_PLACEMENT_3D('',#56406,#30858,#30859);
#27716=AXIS2_PLACEMENT_3D('',#56443,#30861,#30862);
#27717=AXIS2_PLACEMENT_3D('',#56481,#30864,#30865);
#27718=AXIS2_PLACEMENT_3D('',#56518,#30867,#30868);
#27719=AXIS2_PLACEMENT_3D('',#56555,#30870,#30871);
#27720=AXIS2_PLACEMENT_3D('',#56592,#30873,#30874);
#27721=AXIS2_PLACEMENT_3D('',#56629,#30876,#30877);
#27722=AXIS2_PLACEMENT_3D('',#56667,#30879,#30880);
#27723=AXIS2_PLACEMENT_3D('',#56704,#30882,#30883);
#27724=AXIS2_PLACEMENT_3D('',#56741,#30885,#30886);
#27725=AXIS2_PLACEMENT_3D('',#56779,#30888,#30889);
#27726=AXIS2_PLACEMENT_3D('',#56816,#30891,#30892);
#27727=AXIS2_PLACEMENT_3D('',#56853,#30894,#30895);
#27728=AXIS2_PLACEMENT_3D('',#56890,#30897,#30898);
#27729=AXIS2_PLACEMENT_3D('',#56927,#30900,#30901);
#27730=AXIS2_PLACEMENT_3D('',#56965,#30903,#30904);
#27731=AXIS2_PLACEMENT_3D('',#57002,#30906,#30907);
#27732=AXIS2_PLACEMENT_3D('',#57078,#30908,#30909);
#27733=AXIS2_PLACEMENT_3D('',#57080,#30910,#30911);
#27734=AXIS2_PLACEMENT_3D('',#58239,#30912,#30913);
#27735=AXIS2_PLACEMENT_3D('',#58241,#30914,#30915);
#27736=AXIS2_PLACEMENT_3D('',#58242,#30916,#30917);
#27737=AXIS2_PLACEMENT_3D('',#58320,#30918,#30919);
#27738=AXIS2_PLACEMENT_3D('',#58321,#30920,#30921);
#27739=AXIS2_PLACEMENT_3D('',#59322,#30922,#30923);
#27740=AXIS2_PLACEMENT_3D('',#59326,#30925,#30926);
#27741=AXIS2_PLACEMENT_3D('',#59327,#30927,#30928);
#27742=AXIS2_PLACEMENT_3D('',#59330,#30930,#30931);
#27743=AXIS2_PLACEMENT_3D('',#59331,#30932,#30933);
#27744=AXIS2_PLACEMENT_3D('',#59334,#30935,#30936);
#27745=AXIS2_PLACEMENT_3D('',#59335,#30937,#30938);
#27746=AXIS2_PLACEMENT_3D('',#59338,#30940,#30941);
#27747=AXIS2_PLACEMENT_3D('',#59339,#30942,#30943);
#27748=AXIS2_PLACEMENT_3D('',#59342,#30945,#30946);
#27749=AXIS2_PLACEMENT_3D('',#59343,#30947,#30948);
#27750=AXIS2_PLACEMENT_3D('',#59345,#30950,#30951);
#27751=AXIS2_PLACEMENT_3D('',#59346,#30952,#30953);
#27752=AXIS2_PLACEMENT_3D('',#59351,#30955,#30956);
#27753=AXIS2_PLACEMENT_3D('',#59360,#30957,#30958);
#27754=AXIS2_PLACEMENT_3D('',#59369,#30959,#30960);
#27755=AXIS2_PLACEMENT_3D('',#59378,#30961,#30962);
#27756=AXIS2_PLACEMENT_3D('',#59387,#30963,#30964);
#27757=AXIS2_PLACEMENT_3D('',#59396,#30965,#30966);
#27758=AXIS2_PLACEMENT_3D('',#59404,#30967,#30968);
#27759=AXIS2_PLACEMENT_3D('',#59405,#30969,#30970);
#27760=AXIS2_PLACEMENT_3D('',#59411,#30974,#30975);
#27761=AXIS2_PLACEMENT_3D('',#59415,#30978,#30979);
#27762=AXIS2_PLACEMENT_3D('',#59419,#30982,#30983);
#27763=AXIS2_PLACEMENT_3D('',#59423,#30986,#30987);
#27764=AXIS2_PLACEMENT_3D('',#59427,#30990,#30991);
#27765=AXIS2_PLACEMENT_3D('',#59431,#30994,#30995);
#27766=AXIS2_PLACEMENT_3D('',#59435,#30998,#30999);
#27767=AXIS2_PLACEMENT_3D('',#59439,#31002,#31003);
#27768=AXIS2_PLACEMENT_3D('',#59443,#31006,#31007);
#27769=AXIS2_PLACEMENT_3D('',#59445,#31009,#31010);
#27770=AXIS2_PLACEMENT_3D('',#59447,#31012,#31013);
#27771=AXIS2_PLACEMENT_3D('',#59448,#31014,#31015);
#27772=AXIS2_PLACEMENT_3D('',#59450,#31017,#31018);
#27773=AXIS2_PLACEMENT_3D('',#59454,#31021,#31022);
#27774=AXIS2_PLACEMENT_3D('',#59456,#31024,#31025);
#27775=AXIS2_PLACEMENT_3D('',#59458,#31027,#31028);
#27776=AXIS2_PLACEMENT_3D('',#59462,#31031,#31032);
#27777=AXIS2_PLACEMENT_3D('',#59464,#31034,#31035);
#27778=AXIS2_PLACEMENT_3D('',#59465,#31036,#31037);
#27779=AXIS2_PLACEMENT_3D('',#59466,#31038,#31039);
#27780=AXIS2_PLACEMENT_3D('',#59468,#31041,#31042);
#27781=AXIS2_PLACEMENT_3D('',#59469,#31043,#31044);
#27782=AXIS2_PLACEMENT_3D('',#59470,#31045,#31046);
#27783=AXIS2_PLACEMENT_3D('',#59471,#31047,#31048);
#27784=AXIS2_PLACEMENT_3D('',#59473,#31049,#31050);
#27785=AXIS2_PLACEMENT_3D('',#59474,#31051,#31052);
#27786=AXIS2_PLACEMENT_3D('',#59476,#31054,#31055);
#27787=AXIS2_PLACEMENT_3D('',#59477,#31056,#31057);
#27788=AXIS2_PLACEMENT_3D('',#59478,#31058,#31059);
#27789=AXIS2_PLACEMENT_3D('',#59480,#31060,#31061);
#27790=AXIS2_PLACEMENT_3D('',#59482,#31063,#31064);
#30784=DIRECTION('axis',(0.,0.,1.));
#30785=DIRECTION('refdir',(1.,0.,0.));
#30786=DIRECTION('center_axis',(0.,0.,1.));
#30787=DIRECTION('ref_axis',(1.,0.,0.));
#30788=DIRECTION('',(0.,0.,-1.));
#30789=DIRECTION('center_axis',(0.,0.,1.));
#30790=DIRECTION('ref_axis',(1.,0.,0.));
#30791=DIRECTION('center_axis',(0.,0.,1.));
#30792=DIRECTION('ref_axis',(1.,0.,0.));
#30793=DIRECTION('',(0.,0.,-1.));
#30794=DIRECTION('center_axis',(0.,0.,1.));
#30795=DIRECTION('ref_axis',(1.,0.,0.));
#30796=DIRECTION('',(0.,0.,-1.));
#30797=DIRECTION('center_axis',(0.,0.,1.));
#30798=DIRECTION('ref_axis',(1.,0.,0.));
#30799=DIRECTION('',(0.,0.,-1.));
#30800=DIRECTION('center_axis',(0.,0.,1.));
#30801=DIRECTION('ref_axis',(1.,0.,0.));
#30802=DIRECTION('',(0.,0.,-1.));
#30803=DIRECTION('center_axis',(0.,0.,1.));
#30804=DIRECTION('ref_axis',(1.,0.,0.));
#30805=DIRECTION('',(0.,0.,-1.));
#30806=DIRECTION('center_axis',(0.,0.,1.));
#30807=DIRECTION('ref_axis',(1.,0.,0.));
#30808=DIRECTION('',(0.,0.,-1.));
#30809=DIRECTION('center_axis',(0.,0.,1.));
#30810=DIRECTION('ref_axis',(1.,0.,0.));
#30811=DIRECTION('',(0.,0.,-1.));
#30812=DIRECTION('center_axis',(0.,0.,1.));
#30813=DIRECTION('ref_axis',(1.,0.,0.));
#30814=DIRECTION('',(0.,0.,-1.));
#30815=DIRECTION('center_axis',(0.,0.,1.));
#30816=DIRECTION('ref_axis',(1.,0.,0.));
#30817=DIRECTION('',(0.,0.,-1.));
#30818=DIRECTION('center_axis',(0.,0.,1.));
#30819=DIRECTION('ref_axis',(1.,0.,0.));
#30820=DIRECTION('',(0.,0.,-1.));
#30821=DIRECTION('center_axis',(0.,0.,1.));
#30822=DIRECTION('ref_axis',(1.,0.,0.));
#30823=DIRECTION('',(0.,0.,-1.));
#30824=DIRECTION('center_axis',(0.,0.,1.));
#30825=DIRECTION('ref_axis',(1.,0.,0.));
#30826=DIRECTION('',(0.,0.,-1.));
#30827=DIRECTION('center_axis',(0.,0.,1.));
#30828=DIRECTION('ref_axis',(1.,0.,0.));
#30829=DIRECTION('',(0.,0.,-1.));
#30830=DIRECTION('center_axis',(0.,0.,1.));
#30831=DIRECTION('ref_axis',(1.,0.,0.));
#30832=DIRECTION('',(0.,0.,-1.));
#30833=DIRECTION('center_axis',(0.,0.,1.));
#30834=DIRECTION('ref_axis',(1.,0.,0.));
#30835=DIRECTION('',(0.,0.,-1.));
#30836=DIRECTION('center_axis',(0.,0.,1.));
#30837=DIRECTION('ref_axis',(1.,0.,0.));
#30838=DIRECTION('',(0.,0.,-1.));
#30839=DIRECTION('center_axis',(0.,0.,1.));
#30840=DIRECTION('ref_axis',(1.,0.,0.));
#30841=DIRECTION('',(0.,0.,-1.));
#30842=DIRECTION('center_axis',(0.,0.,1.));
#30843=DIRECTION('ref_axis',(1.,0.,0.));
#30844=DIRECTION('',(0.,0.,-1.));
#30845=DIRECTION('center_axis',(0.,0.,1.));
#30846=DIRECTION('ref_axis',(-0.993035084685104,-0.117819016225942,0.));
#30847=DIRECTION('',(0.,0.,1.));
#30848=DIRECTION('center_axis',(0.,0.,1.));
#30849=DIRECTION('ref_axis',(1.,1.24885942597212E-13,0.));
#30850=DIRECTION('center_axis',(0.,0.,1.));
#30851=DIRECTION('ref_axis',(1.,1.24885942597212E-13,0.));
#30852=DIRECTION('',(0.,0.,1.));
#30853=DIRECTION('center_axis',(0.,0.,1.));
#30854=DIRECTION('ref_axis',(1.,1.24885942597212E-13,0.));
#30855=DIRECTION('center_axis',(0.,0.,1.));
#30856=DIRECTION('ref_axis',(1.,1.24885942597212E-13,0.));
#30857=DIRECTION('',(0.,0.,1.));
#30858=DIRECTION('center_axis',(0.,0.,1.));
#30859=DIRECTION('ref_axis',(1.,1.24885942597212E-13,0.));
#30860=DIRECTION('',(0.,0.,1.));
#30861=DIRECTION('center_axis',(0.,0.,1.));
#30862=DIRECTION('ref_axis',(1.,1.24885942597212E-13,0.));
#30863=DIRECTION('',(0.,0.,1.));
#30864=DIRECTION('center_axis',(0.,0.,1.));
#30865=DIRECTION('ref_axis',(1.,1.24885942597212E-13,0.));
#30866=DIRECTION('',(0.,0.,1.));
#30867=DIRECTION('center_axis',(0.,0.,1.));
#30868=DIRECTION('ref_axis',(1.,1.24885942597212E-13,0.));
#30869=DIRECTION('',(0.,0.,1.));
#30870=DIRECTION('center_axis',(0.,0.,1.));
#30871=DIRECTION('ref_axis',(1.,1.24885942597212E-13,0.));
#30872=DIRECTION('',(0.,0.,1.));
#30873=DIRECTION('center_axis',(0.,0.,1.));
#30874=DIRECTION('ref_axis',(1.,1.24885942597212E-13,0.));
#30875=DIRECTION('',(0.,0.,1.));
#30876=DIRECTION('center_axis',(0.,0.,1.));
#30877=DIRECTION('ref_axis',(1.,1.24885942597212E-13,0.));
#30878=DIRECTION('',(0.,0.,1.));
#30879=DIRECTION('center_axis',(0.,0.,1.));
#30880=DIRECTION('ref_axis',(1.,1.24885942597212E-13,0.));
#30881=DIRECTION('',(0.,0.,1.));
#30882=DIRECTION('center_axis',(0.,0.,1.));
#30883=DIRECTION('ref_axis',(1.,1.24885942597212E-13,0.));
#30884=DIRECTION('',(0.,0.,1.));
#30885=DIRECTION('center_axis',(0.,0.,1.));
#30886=DIRECTION('ref_axis',(1.,1.24885942597212E-13,0.));
#30887=DIRECTION('',(0.,0.,1.));
#30888=DIRECTION('center_axis',(0.,0.,1.));
#30889=DIRECTION('ref_axis',(1.,1.24885942597212E-13,0.));
#30890=DIRECTION('',(0.,0.,1.));
#30891=DIRECTION('center_axis',(0.,0.,1.));
#30892=DIRECTION('ref_axis',(1.,1.24885942597212E-13,0.));
#30893=DIRECTION('',(0.,0.,1.));
#30894=DIRECTION('center_axis',(0.,0.,1.));
#30895=DIRECTION('ref_axis',(1.,1.24885942597212E-13,0.));
#30896=DIRECTION('',(0.,0.,1.));
#30897=DIRECTION('center_axis',(0.,0.,1.));
#30898=DIRECTION('ref_axis',(1.,1.24885942597212E-13,0.));
#30899=DIRECTION('',(0.,0.,1.));
#30900=DIRECTION('center_axis',(0.,0.,1.));
#30901=DIRECTION('ref_axis',(1.,1.24885942597212E-13,0.));
#30902=DIRECTION('',(0.,0.,1.));
#30903=DIRECTION('center_axis',(0.,0.,1.));
#30904=DIRECTION('ref_axis',(1.,1.24885942597212E-13,0.));
#30905=DIRECTION('',(0.,0.,1.));
#30906=DIRECTION('center_axis',(0.,0.,1.));
#30907=DIRECTION('ref_axis',(1.,0.,0.));
#30908=DIRECTION('center_axis',(0.,0.,-1.));
#30909=DIRECTION('ref_axis',(1.,0.,0.));
#30910=DIRECTION('center_axis',(0.,0.,-1.));
#30911=DIRECTION('ref_axis',(1.,0.,0.));
#30912=DIRECTION('center_axis',(0.,0.,1.));
#30913=DIRECTION('ref_axis',(1.,0.,0.));
#30914=DIRECTION('center_axis',(0.,0.,1.));
#30915=DIRECTION('ref_axis',(1.,0.,0.));
#30916=DIRECTION('center_axis',(0.,0.,1.));
#30917=DIRECTION('ref_axis',(1.,0.,0.));
#30918=DIRECTION('center_axis',(0.,0.,-1.));
#30919=DIRECTION('ref_axis',(1.,1.24885942597212E-13,0.));
#30920=DIRECTION('center_axis',(0.,0.,1.));
#30921=DIRECTION('ref_axis',(0.88898726725207,0.457931914877853,0.));
#30922=DIRECTION('center_axis',(0.,0.,1.));
#30923=DIRECTION('ref_axis',(1.,0.,0.));
#30924=DIRECTION('',(-1.,2.40370335797945E-16,0.));
#30925=DIRECTION('center_axis',(0.,0.,1.));
#30926=DIRECTION('ref_axis',(1.,0.,0.));
#30927=DIRECTION('center_axis',(0.,0.,1.));
#30928=DIRECTION('ref_axis',(1.,0.,0.));
#30929=DIRECTION('',(-0.5,0.866025403784439,0.));
#30930=DIRECTION('center_axis',(0.,0.,1.));
#30931=DIRECTION('ref_axis',(1.,0.,0.));
#30932=DIRECTION('center_axis',(0.,0.,1.));
#30933=DIRECTION('ref_axis',(1.,0.,0.));
#30934=DIRECTION('',(0.5,0.866025403784439,0.));
#30935=DIRECTION('center_axis',(0.,0.,1.));
#30936=DIRECTION('ref_axis',(1.,0.,0.));
#30937=DIRECTION('center_axis',(0.,0.,1.));
#30938=DIRECTION('ref_axis',(1.,0.,0.));
#30939=DIRECTION('',(1.,-1.20185167898973E-16,0.));
#30940=DIRECTION('center_axis',(0.,0.,1.));
#30941=DIRECTION('ref_axis',(1.,0.,0.));
#30942=DIRECTION('center_axis',(0.,0.,1.));
#30943=DIRECTION('ref_axis',(1.,0.,0.));
#30944=DIRECTION('',(0.5,-0.866025403784439,0.));
#30945=DIRECTION('center_axis',(0.,0.,1.));
#30946=DIRECTION('ref_axis',(1.,0.,0.));
#30947=DIRECTION('center_axis',(0.,0.,1.));
#30948=DIRECTION('ref_axis',(1.,0.,0.));
#30949=DIRECTION('',(-0.5,-0.866025403784439,0.));
#30950=DIRECTION('center_axis',(0.,0.,1.));
#30951=DIRECTION('ref_axis',(1.,0.,0.));
#30952=DIRECTION('center_axis',(0.,0.,1.));
#30953=DIRECTION('ref_axis',(1.,0.,0.));
#30954=DIRECTION('',(-0.856673567959776,-1.04912254291608E-16,0.515858893457375));
#30955=DIRECTION('center_axis',(0.,0.,-1.));
#30956=DIRECTION('ref_axis',(1.,0.,0.));
#30957=DIRECTION('center_axis',(0.,0.,-1.));
#30958=DIRECTION('ref_axis',(1.,0.,0.));
#30959=DIRECTION('center_axis',(0.,0.,-1.));
#30960=DIRECTION('ref_axis',(1.,0.,0.));
#30961=DIRECTION('center_axis',(0.,0.,-1.));
#30962=DIRECTION('ref_axis',(1.,0.,0.));
#30963=DIRECTION('center_axis',(0.,0.,-1.));
#30964=DIRECTION('ref_axis',(1.,0.,0.));
#30965=DIRECTION('center_axis',(0.,0.,-1.));
#30966=DIRECTION('ref_axis',(1.,0.,0.));
#30967=DIRECTION('center_axis',(0.,0.,-1.));
#30968=DIRECTION('ref_axis',(1.,0.,0.));
#30969=DIRECTION('center_axis',(-0.866025403784439,0.5,0.));
#30970=DIRECTION('ref_axis',(0.5,0.866025403784439,0.));
#30971=DIRECTION('',(0.,0.,-1.));
#30972=DIRECTION('',(0.5,0.866025403784439,0.));
#30973=DIRECTION('',(0.,0.,-1.));
#30974=DIRECTION('center_axis',(-0.866025403784439,0.5,0.));
#30975=DIRECTION('ref_axis',(0.5,0.866025403784439,0.));
#30976=DIRECTION('',(0.,0.,-1.));
#30977=DIRECTION('',(0.5,0.866025403784439,0.));
#30978=DIRECTION('center_axis',(1.20185167898973E-16,1.,0.));
#30979=DIRECTION('ref_axis',(1.,-1.20185167898973E-16,0.));
#30980=DIRECTION('',(0.,0.,-1.));
#30981=DIRECTION('',(1.,-1.20185167898973E-16,0.));
#30982=DIRECTION('center_axis',(1.20185167898973E-16,1.,0.));
#30983=DIRECTION('ref_axis',(1.,-1.20185167898973E-16,0.));
#30984=DIRECTION('',(1.,-1.20185167898973E-16,0.));
#30985=DIRECTION('',(0.,0.,-1.));
#30986=DIRECTION('center_axis',(1.20185167898973E-16,1.,0.));
#30987=DIRECTION('ref_axis',(1.,-1.20185167898973E-16,0.));
#30988=DIRECTION('',(0.,0.,-1.));
#30989=DIRECTION('',(1.,-1.20185167898973E-16,0.));
#30990=DIRECTION('center_axis',(-0.866025403784439,-0.5,0.));
#30991=DIRECTION('ref_axis',(-0.5,0.866025403784439,0.));
#30992=DIRECTION('',(-0.5,0.866025403784439,0.));
#30993=DIRECTION('',(0.,0.,-1.));
#30994=DIRECTION('center_axis',(-0.866025403784439,-0.5,0.));
#30995=DIRECTION('ref_axis',(-0.5,0.866025403784439,0.));
#30996=DIRECTION('',(0.,0.,-1.));
#30997=DIRECTION('',(-0.5,0.866025403784439,0.));
#30998=DIRECTION('center_axis',(0.866025403784439,0.5,0.));
#30999=DIRECTION('ref_axis',(0.5,-0.866025403784439,0.));
#31000=DIRECTION('',(0.,0.,-1.));
#31001=DIRECTION('',(0.5,-0.866025403784439,0.));
#31002=DIRECTION('center_axis',(0.866025403784439,0.5,0.));
#31003=DIRECTION('ref_axis',(0.5,-0.866025403784439,0.));
#31004=DIRECTION('',(0.5,-0.866025403784439,0.));
#31005=DIRECTION('',(0.,0.,-1.));
#31006=DIRECTION('center_axis',(0.866025403784439,0.5,0.));
#31007=DIRECTION('ref_axis',(0.5,-0.866025403784439,0.));
#31008=DIRECTION('',(0.5,-0.866025403784439,0.));
#31009=DIRECTION('center_axis',(0.,0.,-1.));
#31010=DIRECTION('ref_axis',(-1.,0.,0.));
#31011=DIRECTION('',(0.5,0.866025403784439,0.));
#31012=DIRECTION('center_axis',(0.,0.,-1.));
#31013=DIRECTION('ref_axis',(-1.,0.,0.));
#31014=DIRECTION('center_axis',(0.,0.,-1.));
#31015=DIRECTION('ref_axis',(-1.,0.,0.));
#31016=DIRECTION('',(-0.5,-0.866025403784439,0.));
#31017=DIRECTION('center_axis',(0.,0.,-1.));
#31018=DIRECTION('ref_axis',(-1.,0.,0.));
#31019=DIRECTION('',(-1.,2.40370335797945E-16,0.));
#31020=DIRECTION('',(-0.5,-0.866025403784439,0.));
#31021=DIRECTION('center_axis',(0.,0.,-1.));
#31022=DIRECTION('ref_axis',(-1.,0.,0.));
#31023=DIRECTION('',(-1.,2.40370335797945E-16,0.));
#31024=DIRECTION('center_axis',(0.,0.,-1.));
#31025=DIRECTION('ref_axis',(-1.,0.,0.));
#31026=DIRECTION('',(-0.5,0.866025403784439,0.));
#31027=DIRECTION('center_axis',(0.866025403784439,-0.5,0.));
#31028=DIRECTION('ref_axis',(-0.5,-0.866025403784439,0.));
#31029=DIRECTION('',(0.,0.,-1.));
#31030=DIRECTION('',(-0.5,-0.866025403784439,0.));
#31031=DIRECTION('center_axis',(0.866025403784439,-0.5,0.));
#31032=DIRECTION('ref_axis',(-0.5,-0.866025403784439,0.));
#31033=DIRECTION('',(0.,0.,-1.));
#31034=DIRECTION('center_axis',(0.866025403784439,-0.5,0.));
#31035=DIRECTION('ref_axis',(-0.5,-0.866025403784439,0.));
#31036=DIRECTION('center_axis',(-2.40370335797945E-16,-1.,0.));
#31037=DIRECTION('ref_axis',(-1.,2.40370335797945E-16,0.));
#31038=DIRECTION('center_axis',(-2.40370335797945E-16,-1.,0.));
#31039=DIRECTION('ref_axis',(-1.,2.40370335797945E-16,0.));
#31040=DIRECTION('',(-1.,2.40370335797945E-16,0.));
#31041=DIRECTION('center_axis',(-0.866025403784439,0.5,0.));
#31042=DIRECTION('ref_axis',(0.5,0.866025403784439,0.));
#31043=DIRECTION('center_axis',(-0.866025403784439,-0.5,0.));
#31044=DIRECTION('ref_axis',(-0.5,0.866025403784439,0.));
#31045=DIRECTION('center_axis',(-2.40370335797945E-16,-1.,0.));
#31046=DIRECTION('ref_axis',(-1.,2.40370335797945E-16,0.));
#31047=DIRECTION('center_axis',(0.,0.,-1.));
#31048=DIRECTION('ref_axis',(-1.,0.,0.));
#31049=DIRECTION('center_axis',(0.,0.,1.));
#31050=DIRECTION('ref_axis',(1.,0.,0.));
#31051=DIRECTION('center_axis',(0.,0.,1.));
#31052=DIRECTION('ref_axis',(1.,0.,0.));
#31053=DIRECTION('',(0.707106781186547,8.65956056235493E-17,-0.707106781186548));
#31054=DIRECTION('center_axis',(0.,0.,1.));
#31055=DIRECTION('ref_axis',(0.0319324117378754,-0.999490030505859,0.));
#31056=DIRECTION('center_axis',(0.,0.,-1.));
#31057=DIRECTION('ref_axis',(1.,0.,0.));
#31058=DIRECTION('center_axis',(0.,0.,-1.));
#31059=DIRECTION('ref_axis',(1.,0.,0.));
#31060=DIRECTION('center_axis',(0.,0.,1.));
#31061=DIRECTION('ref_axis',(1.,0.,0.));
#31062=DIRECTION('',(-0.707106781186548,-8.65956056235494E-17,-0.707106781186547));
#31063=DIRECTION('center_axis',(0.,0.,1.));
#31064=DIRECTION('ref_axis',(1.,0.,0.));
#54710=CARTESIAN_POINT('',(0.,0.,0.));
#54711=CARTESIAN_POINT('Origin',(0.,0.,-1.94));
#54712=CARTESIAN_POINT('',(-0.791104428578755,2.03359169429485E-5,-3.7446668491763));
#54713=CARTESIAN_POINT('',(-0.791090383745199,1.30219247384927E-5,-3.77313315082371));
#54714=CARTESIAN_POINT('',(-0.7911,-9.68818082805471E-17,-1.94));
#54715=CARTESIAN_POINT('',(0.342081771909262,0.713331083684022,-3.8089));
#54716=CARTESIAN_POINT('Ctrl Pts',(-0.791104428578755,2.03359169429485E-5,
-3.7446668491763));
#54717=CARTESIAN_POINT('Ctrl Pts',(-0.791134076001446,0.0289074239465487,
-3.74582920226268));
#54718=CARTESIAN_POINT('Ctrl Pts',(-0.789582317070316,0.0577913339263522,
-3.74699155534907));
#54719=CARTESIAN_POINT('Ctrl Pts',(-0.786424813073281,0.0864986137826184,
-3.74815390843545));
#54720=CARTESIAN_POINT('Ctrl Pts',(-0.772073336273596,0.216978847925223,
-3.75343703186711));
#54721=CARTESIAN_POINT('Ctrl Pts',(-0.724549072123798,0.343810113341632,
-3.75872015529877));
#54722=CARTESIAN_POINT('Ctrl Pts',(-0.649622613351398,0.451592994815809,
-3.76400327873043));
#54723=CARTESIAN_POINT('Ctrl Pts',(-0.574696154578998,0.559375876289986,
-3.76928640216209));
#54724=CARTESIAN_POINT('Ctrl Pts',(-0.472367501183996,0.648110373821931,
-3.77456952559375));
#54725=CARTESIAN_POINT('Ctrl Pts',(-0.355061677451252,0.707020342729974,
-3.77985264902541));
#54726=CARTESIAN_POINT('Ctrl Pts',(-0.237755853718509,0.765930311638017,
-3.78513577245707));
#54727=CARTESIAN_POINT('Ctrl Pts',(-0.105472859648023,0.795015751922158,
-3.79041889588873));
#54728=CARTESIAN_POINT('Ctrl Pts',(0.0257249193947987,0.790748341450471,
-3.79570201932039));
#54729=CARTESIAN_POINT('Ctrl Pts',(0.134975048629466,0.787194812199209,
-3.8001013462136));
#54730=CARTESIAN_POINT('Ctrl Pts',(0.243472677435947,0.760514037346664,
-3.8045006731068));
#54731=CARTESIAN_POINT('Ctrl Pts',(0.342095581308745,0.713339856610551,
-3.8089));
#54732=CARTESIAN_POINT('',(-0.342067962509748,0.713322310757507,-3.8089));
#54733=CARTESIAN_POINT('Origin',(0.,0.,-3.8089));
#54734=CARTESIAN_POINT('Ctrl Pts',(-0.342067962509747,0.713322310757508,
-3.8089));
#54735=CARTESIAN_POINT('Ctrl Pts',(-0.460461074940846,0.65654784831081,
-3.80361687656834));
#54736=CARTESIAN_POINT('Ctrl Pts',(-0.564388400447012,0.569759817632143,
-3.79833375313668));
#54737=CARTESIAN_POINT('Ctrl Pts',(-0.641269208406438,0.463381943464528,
-3.79305062970502));
#54738=CARTESIAN_POINT('Ctrl Pts',(-0.718150016365868,0.357004069296908,
-3.78776750627336));
#54739=CARTESIAN_POINT('Ctrl Pts',(-0.767984306778557,0.231036351640338,
-3.7824843828417));
#54740=CARTESIAN_POINT('Ctrl Pts',(-0.784715742391765,0.100833355385061,
-3.77720125941004));
#54741=CARTESIAN_POINT('Ctrl Pts',(-0.789010253505645,0.0674137357298711,
-3.7758452232146));
#54742=CARTESIAN_POINT('Ctrl Pts',(-0.791123911091846,0.0337150911286863,
-3.77448918701915));
#54743=CARTESIAN_POINT('Ctrl Pts',(-0.791090383745199,1.30219247384927E-5,
-3.77313315082371));
#54744=CARTESIAN_POINT('Origin',(0.,0.,-1.94));
#54745=CARTESIAN_POINT('',(-0.791128448098422,-1.786362598305E-5,-3.5446668491763));
#54746=CARTESIAN_POINT('',(-0.791142152082714,-1.50645020713617E-5,-3.57313315082371));
#54747=CARTESIAN_POINT('',(-0.7911,-9.68818082805471E-17,-1.94));
#54748=CARTESIAN_POINT('Ctrl Pts',(-0.791128448098422,-1.786362598305E-5,
-3.5446668491763));
#54749=CARTESIAN_POINT('Ctrl Pts',(-0.791020967662586,0.110106180651968,
-3.54909838774943));
#54750=CARTESIAN_POINT('Ctrl Pts',(-0.767821030540255,0.220274089461432,
-3.55352992632255));
#54751=CARTESIAN_POINT('Ctrl Pts',(-0.723158334650058,0.320917426638007,
-3.55796146489568));
#54752=CARTESIAN_POINT('Ctrl Pts',(-0.669913049455132,0.440900850928166,
-3.56324458832734));
#54753=CARTESIAN_POINT('Ctrl Pts',(-0.586163680035589,0.547347416399969,
-3.56852771175901));
#54754=CARTESIAN_POINT('Ctrl Pts',(-0.482079359508604,0.627332019525317,
-3.57381083519067));
#54755=CARTESIAN_POINT('Ctrl Pts',(-0.37799503898162,0.707316622650663,
-3.57909395862233));
#54756=CARTESIAN_POINT('Ctrl Pts',(-0.253575767347198,0.760839263429553,
-3.58437708205399));
#54757=CARTESIAN_POINT('Ctrl Pts',(-0.123928955457381,0.781401040356963,
-3.58966020548565));
#54758=CARTESIAN_POINT('Ctrl Pts',(0.00571785643243594,0.801962817284373,
-3.59494332891731));
#54759=CARTESIAN_POINT('Ctrl Pts',(0.140592208577647,0.789563730360299,
-3.60022645234897));
#54760=CARTESIAN_POINT('Ctrl Pts',(0.264317198649155,0.745709319909767,
-3.60550957578063));
#54761=CARTESIAN_POINT('Ctrl Pts',(0.388042188720661,0.701854909459236,
-3.61079269921229));
#54762=CARTESIAN_POINT('Ctrl Pts',(0.500617816718466,0.626545175482247,
-3.61607582264395));
#54763=CARTESIAN_POINT('Ctrl Pts',(0.588374767319508,0.528924479815501,
-3.62135894607561));
#54764=CARTESIAN_POINT('Ctrl Pts',(0.67613171792055,0.431303784148756,-3.62664206950727));
#54765=CARTESIAN_POINT('Ctrl Pts',(0.739069991124828,0.311372126792253,
-3.63192519293893));
#54766=CARTESIAN_POINT('Ctrl Pts',(0.76954740770552,0.183692021249386,-3.63720831637059));
#54767=CARTESIAN_POINT('Ctrl Pts',(0.800024824286212,0.0560119157065181,
-3.64249143980225));
#54768=CARTESIAN_POINT('Ctrl Pts',(0.798041384243317,-0.0794166380227145,
-3.64777456323391));
#54769=CARTESIAN_POINT('Ctrl Pts',(0.763837923925609,-0.206149452463652,
-3.65305768666557));
#54770=CARTESIAN_POINT('Ctrl Pts',(0.729634463607901,-0.33288226690459,
-3.65834081009723));
#54771=CARTESIAN_POINT('Ctrl Pts',(0.66321098301538,-0.450919342057233,
-3.66362393352889));
#54772=CARTESIAN_POINT('Ctrl Pts',(0.572632846320033,-0.54592819965897,
-3.66890705696055));
#54773=CARTESIAN_POINT('Ctrl Pts',(0.482054709624687,-0.640937057260705,
-3.67419018039221));
#54774=CARTESIAN_POINT('Ctrl Pts',(0.367321916826515,-0.712917697311535,
-3.67947330382387));
#54775=CARTESIAN_POINT('Ctrl Pts',(0.242365714829211,-0.753130015950053,
-3.68475642725553));
#54776=CARTESIAN_POINT('Ctrl Pts',(0.117409512831907,-0.793342334588571,
-3.69003955068719));
#54777=CARTESIAN_POINT('Ctrl Pts',(-0.0177700983645308,-0.801786331814778,
-3.69532267411885));
#54778=CARTESIAN_POINT('Ctrl Pts',(-0.146759153262384,-0.777436649787474,
-3.70060579755051));
#54779=CARTESIAN_POINT('Ctrl Pts',(-0.275748208160238,-0.753086967760169,
-3.70588892098217));
#54780=CARTESIAN_POINT('Ctrl Pts',(-0.398546706759508,-0.695943606479353,
-3.71117204441383));
#54781=CARTESIAN_POINT('Ctrl Pts',(-0.500244033294698,-0.612945222655453,
-3.71645516784549));
#54782=CARTESIAN_POINT('Ctrl Pts',(-0.601941359829888,-0.529946838831553,
-3.72173829127715));
#54783=CARTESIAN_POINT('Ctrl Pts',(-0.682537514300998,-0.421093432464569,
-3.72702141470881));
#54784=CARTESIAN_POINT('Ctrl Pts',(-0.732246246811768,-0.299602127846677,
-3.73230453814047));
#54785=CARTESIAN_POINT('Ctrl Pts',(-0.771018437823636,-0.20484042641111,
-3.73642530848574));
#54786=CARTESIAN_POINT('Ctrl Pts',(-0.790999322633179,-0.10239007371512,
-3.74054607883102));
#54787=CARTESIAN_POINT('Ctrl Pts',(-0.791104428578755,2.03359169429485E-5,
-3.7446668491763));
#54788=CARTESIAN_POINT('Ctrl Pts',(-0.791090383745199,1.30219247384927E-5,
-3.77313315082371));
#54789=CARTESIAN_POINT('Ctrl Pts',(-0.790993288390722,-0.0975883299045687,
-3.76920606358749));
#54790=CARTESIAN_POINT('Ctrl Pts',(-0.772888089260372,-0.195218403340946,
-3.76527897635128));
#54791=CARTESIAN_POINT('Ctrl Pts',(-0.737592540570363,-0.286183324054275,
-3.76135188911506));
#54792=CARTESIAN_POINT('Ctrl Pts',(-0.690109322322024,-0.408558732384351,
-3.7560687656834));
#54793=CARTESIAN_POINT('Ctrl Pts',(-0.611514305011616,-0.518871274190519,
-3.75078564225174));
#54794=CARTESIAN_POINT('Ctrl Pts',(-0.511349099416939,-0.603713633894183,
-3.74550251882008));
#54795=CARTESIAN_POINT('Ctrl Pts',(-0.411183893822262,-0.688555993597846,
-3.74021939538842));
#54796=CARTESIAN_POINT('Ctrl Pts',(-0.289448499943316,-0.747928171199005,
-3.73493627195676));
#54797=CARTESIAN_POINT('Ctrl Pts',(-0.160925296224211,-0.774627492756042,
-3.7296531485251));
#54798=CARTESIAN_POINT('Ctrl Pts',(-0.0324020925051069,-0.80132681431308,
-3.72437002509344));
#54799=CARTESIAN_POINT('Ctrl Pts',(0.102908921054156,-0.795353279825997,
-3.71908690166178));
#54800=CARTESIAN_POINT('Ctrl Pts',(0.228578257335151,-0.75742890064077,
-3.71380377823012));
#54801=CARTESIAN_POINT('Ctrl Pts',(0.354247593616146,-0.719504521455543,
-3.70852065479846));
#54802=CARTESIAN_POINT('Ctrl Pts',(0.470275252618875,-0.649629297572173,
-3.7032375313668));
#54803=CARTESIAN_POINT('Ctrl Pts',(0.562572538830204,-0.556289409358392,
-3.69795440793514));
#54804=CARTESIAN_POINT('Ctrl Pts',(0.654869825041534,-0.462949521144612,
-3.69267128450348));
#54805=CARTESIAN_POINT('Ctrl Pts',(0.723436738461466,-0.34614496860042,
-3.68738816107182));
#54806=CARTESIAN_POINT('Ctrl Pts',(0.759947765185156,-0.220057692724725,
-3.68210503764016));
#54807=CARTESIAN_POINT('Ctrl Pts',(0.796458791908846,-0.0939704168490289,
-3.6768219142085));
#54808=CARTESIAN_POINT('Ctrl Pts',(0.800913931936294,0.0413995823581705,
-3.67153879077684));
#54809=CARTESIAN_POINT('Ctrl Pts',(0.77277216890208,0.16961477774449,-3.66625566734518));
#54810=CARTESIAN_POINT('Ctrl Pts',(0.744630405867867,0.297829973130809,
-3.66097254391352));
#54811=CARTESIAN_POINT('Ctrl Pts',(0.683891739771991,0.418890364696249,
-3.65568942048186));
#54812=CARTESIAN_POINT('Ctrl Pts',(0.597931295593872,0.518096613818281,
-3.6504062970502));
#54813=CARTESIAN_POINT('Ctrl Pts',(0.511970851415752,0.617302862940314,
-3.64512317361854));
#54814=CARTESIAN_POINT('Ctrl Pts',(0.400788629155388,0.694654969618939,
-3.63984005018688));
#54815=CARTESIAN_POINT('Ctrl Pts',(0.277884736994597,0.740760462896105,
-3.63455692675522));
#54816=CARTESIAN_POINT('Ctrl Pts',(0.154980844833807,0.786865956173271,
-3.62927380332356));
#54817=CARTESIAN_POINT('Ctrl Pts',(0.0203552827725882,0.801724836048977,
-3.6239906798919));
#54818=CARTESIAN_POINT('Ctrl Pts',(-0.109645248094981,0.783532945683037,
-3.61870755646024));
#54819=CARTESIAN_POINT('Ctrl Pts',(-0.239645778962551,0.765341055317096,
-3.61342443302858));
#54820=CARTESIAN_POINT('Ctrl Pts',(-0.365021278636471,0.714098394709508,
-3.60814130959692));
#54821=CARTESIAN_POINT('Ctrl Pts',(-0.470548231740154,0.636026991824806,
-3.60285818616526));
#54822=CARTESIAN_POINT('Ctrl Pts',(-0.576075184843836,0.557955588940104,
-3.5975750627336));
#54823=CARTESIAN_POINT('Ctrl Pts',(-0.66175359137728,0.453055443778288,
-3.59229193930193));
#54824=CARTESIAN_POINT('Ctrl Pts',(-0.717180085970426,0.334063903885682,
-3.58700881587028));
#54825=CARTESIAN_POINT('Ctrl Pts',(-0.765704378063189,0.229890254068931,
-3.58238359418809));
#54826=CARTESIAN_POINT('Ctrl Pts',(-0.791042104935038,0.114916260669801,
-3.5777583725059));
#54827=CARTESIAN_POINT('Ctrl Pts',(-0.791142152082714,-1.50645020713617E-5,
-3.57313315082371));
#54828=CARTESIAN_POINT('Origin',(0.,0.,-1.94));
#54829=CARTESIAN_POINT('',(-0.791034765442454,5.10246101870227E-6,-3.3446668491763));
#54830=CARTESIAN_POINT('',(-0.791032851165218,6.96852469137922E-7,-3.3731331508237));
#54831=CARTESIAN_POINT('',(-0.7911,-9.68818082805471E-17,-1.94));
#54832=CARTESIAN_POINT('Ctrl Pts',(-0.791034765442454,5.10246101870227E-6,
-3.3446668491763));
#54833=CARTESIAN_POINT('Ctrl Pts',(-0.791048344631556,0.0601030927221048,
-3.34708444980451));
#54834=CARTESIAN_POINT('Ctrl Pts',(-0.784287366750522,0.120198076074771,
-3.34950205043273));
#54835=CARTESIAN_POINT('Ctrl Pts',(-0.770718569515641,0.178714460170998,
-3.35191965106094));
#54836=CARTESIAN_POINT('Ctrl Pts',(-0.74106700929745,0.306588880928024,
-3.3572027744926));
#54837=CARTESIAN_POINT('Ctrl Pts',(-0.678905190912391,0.426924812970615,
-3.36248589792426));
#54838=CARTESIAN_POINT('Ctrl Pts',(-0.591781013642106,0.525110658398002,
-3.36776902135592));
#54839=CARTESIAN_POINT('Ctrl Pts',(-0.50465683637182,0.623296503825389,
-3.37305214478758));
#54840=CARTESIAN_POINT('Ctrl Pts',(-0.392570300216308,0.699332262637573,
-3.37833526821924));
#54841=CARTESIAN_POINT('Ctrl Pts',(-0.269131333387287,0.743985414547624,
-3.3836183916509));
#54842=CARTESIAN_POINT('Ctrl Pts',(-0.145692366558263,0.788638566457676,
-3.38890151508256));
#54843=CARTESIAN_POINT('Ctrl Pts',(-0.0109009690557307,0.801909111465594,
-3.39418463851422));
#54844=CARTESIAN_POINT('Ctrl Pts',(0.118876029468087,0.782185694888634,
-3.39946776194588));
#54845=CARTESIAN_POINT('Ctrl Pts',(0.248653027991902,0.762462278311674,
-3.40475088537754));
#54846=CARTESIAN_POINT('Ctrl Pts',(0.373415627537002,0.709744900149836,
-3.4100340088092));
#54847=CARTESIAN_POINT('Ctrl Pts',(0.478014729187874,0.630434683650731,
-3.41531713224086));
#54848=CARTESIAN_POINT('Ctrl Pts',(0.582613830838747,0.551124467151625,
-3.42060025567252));
#54849=CARTESIAN_POINT('Ctrl Pts',(0.667049434595391,0.445221412315251,
-3.42588337910418));
#54850=CARTESIAN_POINT('Ctrl Pts',(0.721069082445871,0.325584628032729,
-3.43116650253584));
#54851=CARTESIAN_POINT('Ctrl Pts',(0.77508873029635,0.205947843750209,-3.4364496259675));
#54852=CARTESIAN_POINT('Ctrl Pts',(0.798692422240667,0.0725773300215417,
-3.44173274939916));
#54853=CARTESIAN_POINT('Ctrl Pts',(0.789014117771925,-0.0583326120373118,
-3.44701587283082));
#54854=CARTESIAN_POINT('Ctrl Pts',(0.779335813303183,-0.189242554096167,
-3.45229899626248));
#54855=CARTESIAN_POINT('Ctrl Pts',(0.736375512421381,-0.317691924485209,
-3.45758211969414));
#54856=CARTESIAN_POINT('Ctrl Pts',(0.665349600885421,-0.42808396404388,
-3.4628652431258));
#54857=CARTESIAN_POINT('Ctrl Pts',(0.594323689349462,-0.538476003602551,
-3.46814836655746));
#54858=CARTESIAN_POINT('Ctrl Pts',(0.495232167159344,-0.630810712330852,
-3.47343148998912));
#54859=CARTESIAN_POINT('Ctrl Pts',(0.380107063759745,-0.693876496036605,
-3.47871461342078));
#54860=CARTESIAN_POINT('Ctrl Pts',(0.264981960360147,-0.756942279742356,
-3.48399773685244));
#54861=CARTESIAN_POINT('Ctrl Pts',(0.13382327575107,-0.79073913842556,-3.4892808602841));
#54862=CARTESIAN_POINT('Ctrl Pts',(0.00255674323769956,-0.791163342635944,
-3.49456398371576));
#54863=CARTESIAN_POINT('Ctrl Pts',(-0.128709789275672,-0.791587546846327,
-3.49984710714743));
#54864=CARTESIAN_POINT('Ctrl Pts',(-0.260084169693336,-0.75863909658389,
-3.50513023057909));
#54865=CARTESIAN_POINT('Ctrl Pts',(-0.375614474192984,-0.69631870465558,
-3.51041335401075));
#54866=CARTESIAN_POINT('Ctrl Pts',(-0.491144778692633,-0.633998312727271,
-3.51569647744241));
#54867=CARTESIAN_POINT('Ctrl Pts',(-0.590831007274266,-0.542305979133088,
-3.52097960087406));
#54868=CARTESIAN_POINT('Ctrl Pts',(-0.662568919220032,-0.432375298724376,
-3.52626272430572));
#54869=CARTESIAN_POINT('Ctrl Pts',(-0.734306831165799,-0.322444618315663,
-3.53154584773739));
#54870=CARTESIAN_POINT('Ctrl Pts',(-0.778096426475699,-0.194275591092421,
-3.53682897116905));
#54871=CARTESIAN_POINT('Ctrl Pts',(-0.788620623645495,-0.0634309359265427,
-3.54211209460071));
#54872=CARTESIAN_POINT('Ctrl Pts',(-0.790317015386842,-0.0423401307238582,
-3.54296367945924));
#54873=CARTESIAN_POINT('Ctrl Pts',(-0.791149102033898,-0.0211798070728596,
-3.54381526431777));
#54874=CARTESIAN_POINT('Ctrl Pts',(-0.791128448098422,-1.786362598305E-5,
-3.5446668491763));
#54875=CARTESIAN_POINT('Ctrl Pts',(-0.791142152082714,-1.50645020713617E-5,
-3.57313315082371));
#54876=CARTESIAN_POINT('Ctrl Pts',(-0.791156383010009,-0.0163631500847965,
-3.57247524907424));
#54877=CARTESIAN_POINT('Ctrl Pts',(-0.790659983849077,-0.0327103723678489,
-3.57181734732477));
#54878=CARTESIAN_POINT('Ctrl Pts',(-0.789647051564748,-0.049025525545824,
-3.5711594455753));
#54879=CARTESIAN_POINT('Ctrl Pts',(-0.781512939913075,-0.18004048046133,
-3.56587632214364));
#54880=CARTESIAN_POINT('Ctrl Pts',(-0.740070133956881,-0.308987455668947,
-3.56059319871197));
#54881=CARTESIAN_POINT('Ctrl Pts',(-0.670350759535863,-0.420209267130899,
-3.55531007528031));
#54882=CARTESIAN_POINT('Ctrl Pts',(-0.600631385114846,-0.531431078592849,
-3.55002695184865));
#54883=CARTESIAN_POINT('Ctrl Pts',(-0.502635442229007,-0.624927726309134,
-3.544743828417));
#54884=CARTESIAN_POINT('Ctrl Pts',(-0.388261931629374,-0.689346531557255,
-3.53946070498534));
#54885=CARTESIAN_POINT('Ctrl Pts',(-0.273888421029741,-0.753765336805377,
-3.53417758155368));
#54886=CARTESIAN_POINT('Ctrl Pts',(-0.143137342716314,-0.789106299585334,
-3.52889445812201));
#54887=CARTESIAN_POINT('Ctrl Pts',(-0.011884936914468,-0.791078199024235,
-3.52361133469035));
#54888=CARTESIAN_POINT('Ctrl Pts',(0.119367468887379,-0.793050098463135,
-3.51832821125869));
#54889=CARTESIAN_POINT('Ctrl Pts',(0.251121202177644,-0.761652934560978,
-3.51304508782703));
#54890=CARTESIAN_POINT('Ctrl Pts',(0.367378276747785,-0.700699058214266,
-3.50776196439537));
#54891=CARTESIAN_POINT('Ctrl Pts',(0.483635351317926,-0.639745181867554,
-3.50247884096371));
#54892=CARTESIAN_POINT('Ctrl Pts',(0.584395767167944,-0.549234593076287,
-3.49719571753205));
#54893=CARTESIAN_POINT('Ctrl Pts',(0.657424852147946,-0.440157394912042,
-3.49191259410039));
#54894=CARTESIAN_POINT('Ctrl Pts',(0.730453937127948,-0.331080196747798,
-3.48662947066873));
#54895=CARTESIAN_POINT('Ctrl Pts',(0.775751691237936,-0.203436389210576,
-3.48134634723707));
#54896=CARTESIAN_POINT('Ctrl Pts',(0.787817907184613,-0.0727249174230299,
-3.47606322380541));
#54897=CARTESIAN_POINT('Ctrl Pts',(0.79988412313129,0.0579865543645165,
-3.47078010037375));
#54898=CARTESIAN_POINT('Ctrl Pts',(0.778718800914655,0.191765690402387,
-3.46549697694209));
#54899=CARTESIAN_POINT('Ctrl Pts',(0.726891905910353,0.312368573337293,
-3.46021385351043));
#54900=CARTESIAN_POINT('Ctrl Pts',(0.67506501090605,0.432971456272199,-3.45493073007877));
#54901=CARTESIAN_POINT('Ctrl Pts',(0.592576543114078,0.54039808610414,-3.44964760664711));
#54902=CARTESIAN_POINT('Ctrl Pts',(0.489442532674306,0.621604356250294,
-3.44436448321545));
#54903=CARTESIAN_POINT('Ctrl Pts',(0.386308522234534,0.702810626396448,
-3.43908135978379));
#54904=CARTESIAN_POINT('Ctrl Pts',(0.262528969146962,0.757796536856814,
-3.43379823635213));
#54905=CARTESIAN_POINT('Ctrl Pts',(0.133133607487199,0.779885511500048,
-3.42851511292047));
#54906=CARTESIAN_POINT('Ctrl Pts',(0.00373824582743582,0.801974486143282,
-3.42323198948881));
#54907=CARTESIAN_POINT('Ctrl Pts',(-0.131272924404518,0.791166524969384,
-3.41794886605715));
#54908=CARTESIAN_POINT('Ctrl Pts',(-0.255506388005845,0.748773967351791,
-3.41266574262549));
#54909=CARTESIAN_POINT('Ctrl Pts',(-0.379739851607171,0.706381409734199,
-3.40738261919383));
#54910=CARTESIAN_POINT('Ctrl Pts',(-0.493195608577871,0.632404255672914,
-3.40209949576217));
#54911=CARTESIAN_POINT('Ctrl Pts',(-0.582097475260115,0.535825062673564,
-3.39681637233051));
#54912=CARTESIAN_POINT('Ctrl Pts',(-0.670999341942359,0.439245869674214,
-3.39153324889885));
#54913=CARTESIAN_POINT('Ctrl Pts',(-0.735347318336148,0.3200646377368,-3.38625012546719));
#54914=CARTESIAN_POINT('Ctrl Pts',(-0.767328054423804,0.192752757147877,
-3.38096700203553));
#54915=CARTESIAN_POINT('Ctrl Pts',(-0.78313513845885,0.129826450836074,
-3.37835571829825));
#54916=CARTESIAN_POINT('Ctrl Pts',(-0.791034848401665,0.0649138126686076,
-3.37574443456098));
#54917=CARTESIAN_POINT('Ctrl Pts',(-0.791032851165218,6.96852469137922E-7,
-3.3731331508237));
#54918=CARTESIAN_POINT('Origin',(0.,0.,-1.94));
#54919=CARTESIAN_POINT('',(-0.791156898220181,1.00405986563634E-5,-3.1446668491763));
#54920=CARTESIAN_POINT('',(-0.791146063621827,1.39968631027903E-5,-3.17313315082371));
#54921=CARTESIAN_POINT('',(-0.7911,-9.68818082805471E-17,-1.94));
#54922=CARTESIAN_POINT('Ctrl Pts',(-0.791156898220181,1.00405986563634E-5,
-3.1446668491763));
#54923=CARTESIAN_POINT('Ctrl Pts',(-0.791163256457482,0.0100400424277527,
-3.1450705118596));
#54924=CARTESIAN_POINT('Ctrl Pts',(-0.790976464647033,0.0200698071486357,
-3.1454741745429));
#54925=CARTESIAN_POINT('Ctrl Pts',(-0.790594987006842,0.0300921616056704,
-3.1458778372262));
#54926=CARTESIAN_POINT('Ctrl Pts',(-0.78560222066274,0.161264394915736,
-3.15116096065786));
#54927=CARTESIAN_POINT('Ctrl Pts',(-0.747260774074463,0.291167288182243,
-3.15644408408952));
#54928=CARTESIAN_POINT('Ctrl Pts',(-0.68022619601261,0.404027590553744,
-3.16172720752118));
#54929=CARTESIAN_POINT('Ctrl Pts',(-0.613191617950758,0.516887892925243,
-3.16701033095284));
#54930=CARTESIAN_POINT('Ctrl Pts',(-0.517463908415333,0.612705604401734,
-3.1722934543845));
#54931=CARTESIAN_POINT('Ctrl Pts',(-0.404666651284786,0.679846212763156,
-3.17757657781616));
#54932=CARTESIAN_POINT('Ctrl Pts',(-0.291869394154238,0.74698682112458,
-3.18285970124782));
#54933=CARTESIAN_POINT('Ctrl Pts',(-0.162002589428568,0.785450326370933,
-3.18814282467948));
#54934=CARTESIAN_POINT('Ctrl Pts',(-0.0308351059659308,0.790566358954465,
-3.19342594811114));
#54935=CARTESIAN_POINT('Ctrl Pts',(0.100332377496707,0.795682391537996,
-3.1987090715428));
#54936=CARTESIAN_POINT('Ctrl Pts',(0.232800539696312,0.767450951458705,
-3.20399219497446));
#54937=CARTESIAN_POINT('Ctrl Pts',(0.350484646108009,0.709299996132096,
-3.20927531840612));
#54938=CARTESIAN_POINT('Ctrl Pts',(0.468168752519706,0.651149040805489,
-3.21455844183778));
#54939=CARTESIAN_POINT('Ctrl Pts',(0.571068803143495,0.563078570231564,
-3.21984156526944));
#54940=CARTESIAN_POINT('Ctrl Pts',(0.646690324066575,0.45578240030646,-3.2251246887011));
#54941=CARTESIAN_POINT('Ctrl Pts',(0.722311844989655,0.348486230381356,
-3.23040781213276));
#54942=CARTESIAN_POINT('Ctrl Pts',(0.770654836212026,0.221964361105069,
-3.23569093556442));
#54943=CARTESIAN_POINT('Ctrl Pts',(0.785849327417509,0.0915795079037739,
-3.24097405899608));
#54944=CARTESIAN_POINT('Ctrl Pts',(0.801043818622993,-0.0388053452975232,
-3.24625718242774));
#54945=CARTESIAN_POINT('Ctrl Pts',(0.783089809811589,-0.173053182423831,
-3.2515403058594));
#54946=CARTESIAN_POINT('Ctrl Pts',(0.734167337760388,-0.294863174771408,
-3.25682342929106));
#54947=CARTESIAN_POINT('Ctrl Pts',(0.685244865709187,-0.416673167118983,
-3.26210655272272));
#54948=CARTESIAN_POINT('Ctrl Pts',(0.605353930418191,-0.526045314687827,
-3.26738967615438));
#54949=CARTESIAN_POINT('Ctrl Pts',(0.504195160806543,-0.609699279554858,
-3.27267279958604));
#54950=CARTESIAN_POINT('Ctrl Pts',(0.403036391194895,-0.693353244421891,
-3.2779559230177));
#54951=CARTESIAN_POINT('Ctrl Pts',(0.280609787262598,-0.75128902658711,
-3.28323904644936));
#54952=CARTESIAN_POINT('Ctrl Pts',(0.151780803397594,-0.776471866451342,
-3.28852216988102));
#54953=CARTESIAN_POINT('Ctrl Pts',(0.0229518195325914,-0.801654706315574,
-3.29380529331268));
#54954=CARTESIAN_POINT('Ctrl Pts',(-0.112279544265117,-0.79408460387882,
-3.29908841674434));
#54955=CARTESIAN_POINT('Ctrl Pts',(-0.237493036140256,-0.754680746710377,
-3.304371540176));
#54956=CARTESIAN_POINT('Ctrl Pts',(-0.362706528015396,-0.715276889541934,
-3.30965466360766));
#54957=CARTESIAN_POINT('Ctrl Pts',(-0.477902147967967,-0.644039277641801,
-3.31493778703932));
#54958=CARTESIAN_POINT('Ctrl Pts',(-0.569092452263575,-0.549617823989616,
-3.32022091047098));
#54959=CARTESIAN_POINT('Ctrl Pts',(-0.660282756559183,-0.455196370337432,
-3.32550403390264));
#54960=CARTESIAN_POINT('Ctrl Pts',(-0.727467745197829,-0.337591074933195,
-3.3307871573343));
#54961=CARTESIAN_POINT('Ctrl Pts',(-0.762489588491491,-0.211081972495344,
-3.33607028076596));
#54962=CARTESIAN_POINT('Ctrl Pts',(-0.781485148953939,-0.142464473288981,
-3.33893580356941));
#54963=CARTESIAN_POINT('Ctrl Pts',(-0.791018670362246,-0.0712275732442067,
-3.34180132637285));
#54964=CARTESIAN_POINT('Ctrl Pts',(-0.791034765442454,5.10246101870227E-6,
-3.3446668491763));
#54965=CARTESIAN_POINT('Ctrl Pts',(-0.791032851165218,6.96852469137922E-7,
-3.3731331508237));
#54966=CARTESIAN_POINT('Ctrl Pts',(-0.791030807612638,-0.0664177612599439,
-3.37046131112932));
#54967=CARTESIAN_POINT('Ctrl Pts',(-0.78275632457385,-0.13283671943135,
-3.36778947143493));
#54968=CARTESIAN_POINT('Ctrl Pts',(-0.766215472424178,-0.19712893829106,
-3.36511763174055));
#54969=CARTESIAN_POINT('Ctrl Pts',(-0.733508658555371,-0.324256223900637,
-3.35983450830889));
#54970=CARTESIAN_POINT('Ctrl Pts',(-0.668481535036233,-0.443068265879359,
-3.35455138487723));
#54971=CARTESIAN_POINT('Ctrl Pts',(-0.579029916237292,-0.539138502238536,
-3.34926826144557));
#54972=CARTESIAN_POINT('Ctrl Pts',(-0.48957829743835,-0.635208738597713,
-3.34398513801391));
#54973=CARTESIAN_POINT('Ctrl Pts',(-0.375702183359603,-0.708537169337344,
-3.33870201458225));
#54974=CARTESIAN_POINT('Ctrl Pts',(-0.251228798847089,-0.750220007147094,
-3.33341889115059));
#54975=CARTESIAN_POINT('Ctrl Pts',(-0.126755414334578,-0.791902844956843,
-3.32813576771893));
#54976=CARTESIAN_POINT('Ctrl Pts',(0.00831524061170164,-0.801940089836712,
-3.32285264428727));
#54977=CARTESIAN_POINT('Ctrl Pts',(0.137582427951453,-0.779112985396101,
-3.31756952085561));
#54978=CARTESIAN_POINT('Ctrl Pts',(0.266849615291207,-0.756285880955491,
-3.31228639742395));
#54979=CARTESIAN_POINT('Ctrl Pts',(0.390313335024435,-0.700594427194401,
-3.30700327399229));
#54980=CARTESIAN_POINT('Ctrl Pts',(0.492982202637408,-0.618800869728425,
-3.30172015056063));
#54981=CARTESIAN_POINT('Ctrl Pts',(0.595651070250382,-0.537007312262449,
-3.29643702712897));
#54982=CARTESIAN_POINT('Ctrl Pts',(0.6775250857431,-0.42911165109159,-3.29115390369731));
#54983=CARTESIAN_POINT('Ctrl Pts',(0.728662827857662,-0.308214944141823,
-3.28587078026565));
#54984=CARTESIAN_POINT('Ctrl Pts',(0.779800569972224,-0.187318237192056,
-3.28058765683399));
#54985=CARTESIAN_POINT('Ctrl Pts',(0.800202038708627,-0.0534204844633812,
-3.27530453340233));
#54986=CARTESIAN_POINT('Ctrl Pts',(0.787390018386567,0.0772199937780057,
-3.27002140997067));
#54987=CARTESIAN_POINT('Ctrl Pts',(0.774577998064506,0.207860472019394,
-3.26473828653901));
#54988=CARTESIAN_POINT('Ctrl Pts',(0.728552488683982,0.335243675773492,
-3.25945516310735));
#54989=CARTESIAN_POINT('Ctrl Pts',(0.654902064038613,0.443902303454082,
-3.25417203967569));
#54990=CARTESIAN_POINT('Ctrl Pts',(0.581251639393244,0.552560931134673,
-3.24888891624403));
#54991=CARTESIAN_POINT('Ctrl Pts',(0.479976299483027,0.642494982741753,
-3.24360579281237));
#54992=CARTESIAN_POINT('Ctrl Pts',(0.363373240323399,0.70278436003567,-3.23832266938071));
#54993=CARTESIAN_POINT('Ctrl Pts',(0.246770181163772,0.763073737329586,
-3.23303954594905));
#54994=CARTESIAN_POINT('Ctrl Pts',(0.114839402754731,0.793718440310342,
-3.22775642251739));
#54995=CARTESIAN_POINT('Ctrl Pts',(-0.0163996113453126,0.790997484978048,
-3.22247329908573));
#54996=CARTESIAN_POINT('Ctrl Pts',(-0.147638625445356,0.788276529645754,
-3.21719017565407));
#54997=CARTESIAN_POINT('Ctrl Pts',(-0.278185875236402,0.752189916000409,
-3.21190705222241));
#54998=CARTESIAN_POINT('Ctrl Pts',(-0.392189869907569,0.687119403332316,
-3.20662392879075));
#54999=CARTESIAN_POINT('Ctrl Pts',(-0.506193864578736,0.622048890664222,
-3.20134080535909));
#55000=CARTESIAN_POINT('Ctrl Pts',(-0.603654604130024,0.52799447897338,
-3.19605768192743));
#55001=CARTESIAN_POINT('Ctrl Pts',(-0.672738074287734,0.416376574626269,
-3.19077455849577));
#55002=CARTESIAN_POINT('Ctrl Pts',(-0.741821544445445,0.304758670279158,
-3.18549143506411));
#55003=CARTESIAN_POINT('Ctrl Pts',(-0.782527745209579,0.17557727327578,
-3.18020831163244));
#55004=CARTESIAN_POINT('Ctrl Pts',(-0.789913991319501,0.0445180279388877,
-3.17492518820079));
#55005=CARTESIAN_POINT('Ctrl Pts',(-0.790749130436005,0.0296995801466835,
-3.17432784240843));
#55006=CARTESIAN_POINT('Ctrl Pts',(-0.791158303975227,0.0148571257566993,
-3.17373049661607));
#55007=CARTESIAN_POINT('Ctrl Pts',(-0.791146063621827,1.39968631027903E-5,
-3.17313315082371));
#55008=CARTESIAN_POINT('Origin',(0.,0.,-1.94));
#55009=CARTESIAN_POINT('',(-0.791071031963789,-1.87933227643877E-5,-2.9446668491763));
#55010=CARTESIAN_POINT('',(-0.791084859053011,-2.00741357560715E-5,-2.97313315082371));
#55011=CARTESIAN_POINT('',(-0.7911,-9.68818082805471E-17,-1.94));
#55012=CARTESIAN_POINT('Ctrl Pts',(-0.791071031963789,-1.87933227643877E-5,
-2.9446668491763));
#55013=CARTESIAN_POINT('Ctrl Pts',(-0.790990147666244,0.0912708088080257,
-2.94833969734634));
#55014=CARTESIAN_POINT('Ctrl Pts',(-0.7752003893603,0.182587668557959,-2.95201254551639));
#55015=CARTESIAN_POINT('Ctrl Pts',(-0.744238000845016,0.268432058012198,
-2.95568539368643));
#55016=CARTESIAN_POINT('Ctrl Pts',(-0.69970086979795,0.39191293290954,-2.96096851711809));
#55017=CARTESIAN_POINT('Ctrl Pts',(-0.623770477316596,0.504070873792558,
-2.96625164054975));
#55018=CARTESIAN_POINT('Ctrl Pts',(-0.525666549749928,0.591287282244812,
-2.97153476398141));
#55019=CARTESIAN_POINT('Ctrl Pts',(-0.427562622183257,0.678503690697069,
-2.97681788741307));
#55020=CARTESIAN_POINT('Ctrl Pts',(-0.307285159531272,0.740778566718563,
-2.98210101084473));
#55021=CARTESIAN_POINT('Ctrl Pts',(-0.179438660142546,0.770550283185138,
-2.98738413427639));
#55022=CARTESIAN_POINT('Ctrl Pts',(-0.0515921607538247,0.800321999651714,
-2.99266725770805));
#55023=CARTESIAN_POINT('Ctrl Pts',(0.0838233753716368,0.797590556563374,
-2.99795038113971));
#55024=CARTESIAN_POINT('Ctrl Pts',(0.210365333548509,0.762687615024313,
-3.00323350457137));
#55025=CARTESIAN_POINT('Ctrl Pts',(0.336907291725384,0.727784673485251,
-3.00851662800303));
#55026=CARTESIAN_POINT('Ctrl Pts',(0.45457567195367,0.660710233495468,-3.01379975143469));
#55027=CARTESIAN_POINT('Ctrl Pts',(0.549082779541173,0.569608701550274,
-3.01908287486635));
#55028=CARTESIAN_POINT('Ctrl Pts',(0.643589887128676,0.47850716960508,-3.02436599829801));
#55029=CARTESIAN_POINT('Ctrl Pts',(0.714935722075396,0.363378545704475,
-3.02964912172967));
#55030=CARTESIAN_POINT('Ctrl Pts',(0.754457230591514,0.238202138694498,
-3.03493224516133));
#55031=CARTESIAN_POINT('Ctrl Pts',(0.793978739107632,0.113025731684523,
-3.04021536859299));
#55032=CARTESIAN_POINT('Ctrl Pts',(0.801675921193149,-0.0221984584348243,
-3.04549849202465));
#55033=CARTESIAN_POINT('Ctrl Pts',(0.776614158835862,-0.151051050860679,
-3.05078161545631));
#55034=CARTESIAN_POINT('Ctrl Pts',(0.751552396478576,-0.279903643286535,
-3.05606473888798));
#55035=CARTESIAN_POINT('Ctrl Pts',(0.693731689678487,-0.402384638018896,
-3.06134786231963));
#55036=CARTESIAN_POINT('Ctrl Pts',(0.610172825192782,-0.503621976354,-3.06663098575129));
#55037=CARTESIAN_POINT('Ctrl Pts',(0.526613960707075,-0.604859314689106,
-3.07191410918295));
#55038=CARTESIAN_POINT('Ctrl Pts',(0.417316938535751,-0.684852996626952,
-3.07719723261461));
#55039=CARTESIAN_POINT('Ctrl Pts',(0.295552974620768,-0.733889917401286,
-3.08248035604627));
#55040=CARTESIAN_POINT('Ctrl Pts',(0.173789010705789,-0.782926838175618,
-3.08776347947793));
#55041=CARTESIAN_POINT('Ctrl Pts',(0.0395581050471505,-0.801006997786439,
-3.09304660290959));
#55042=CARTESIAN_POINT('Ctrl Pts',(-0.0908409695277596,-0.785935041797798,
-3.09832972634125));
#55043=CARTESIAN_POINT('Ctrl Pts',(-0.221240044102672,-0.770863085809156,
-3.10361284977292));
#55044=CARTESIAN_POINT('Ctrl Pts',(-0.347807287593856,-0.722639014221051,
-3.10889597320458));
#55045=CARTESIAN_POINT('Ctrl Pts',(-0.455174475083741,-0.647118357723447,
-3.11417909663624));
#55046=CARTESIAN_POINT('Ctrl Pts',(-0.562541662573625,-0.571597701225844,
-3.11946222006789));
#55047=CARTESIAN_POINT('Ctrl Pts',(-0.65070879406221,-0.468780459818742,
-3.12474534349956));
#55048=CARTESIAN_POINT('Ctrl Pts',(-0.708970316756539,-0.35115105243838,
-3.13002846693122));
#55049=CARTESIAN_POINT('Ctrl Pts',(-0.762780305639831,-0.242509245448644,
-3.13490792767958));
#55050=CARTESIAN_POINT('Ctrl Pts',(-0.791080040064552,-0.121232279427034,
-3.13978738842794));
#55051=CARTESIAN_POINT('Ctrl Pts',(-0.791156898220181,1.00405986563634E-5,
-3.1446668491763));
#55052=CARTESIAN_POINT('Ctrl Pts',(-0.791146063621827,1.39968631027903E-5,
-3.17313315082371));
#55053=CARTESIAN_POINT('Ctrl Pts',(-0.791050046247981,-0.116420407390624,
-3.16844737318441));
#55054=CARTESIAN_POINT('Ctrl Pts',(-0.765022950244057,-0.232896316223373,
-3.16376159554511));
#55055=CARTESIAN_POINT('Ctrl Pts',(-0.715261824728976,-0.33815157929433,
-3.15907581790581));
#55056=CARTESIAN_POINT('Ctrl Pts',(-0.659157120572815,-0.456824847520252,
-3.15379269447415));
#55057=CARTESIAN_POINT('Ctrl Pts',(-0.57288142080478,-0.561234290301691,
-3.14850957104249));
#55058=CARTESIAN_POINT('Ctrl Pts',(-0.466910614149181,-0.638702158199507,
-3.14322644761082));
#55059=CARTESIAN_POINT('Ctrl Pts',(-0.360939807493583,-0.716170026097323,
-3.13794332417916));
#55060=CARTESIAN_POINT('Ctrl Pts',(-0.235273893950421,-0.766696319111518,
-3.13266020074751));
#55061=CARTESIAN_POINT('Ctrl Pts',(-0.105171655891279,-0.784145963001124,
-3.12737707731584));
#55062=CARTESIAN_POINT('Ctrl Pts',(0.0249305821678641,-0.80159560689073,
-3.12209395388418));
#55063=CARTESIAN_POINT('Ctrl Pts',(0.159469144742986,-0.785968601655745,
-3.11681083045252));
#55064=CARTESIAN_POINT('Ctrl Pts',(0.28210790225815,-0.739162431389326,
-3.11152770702086));
#55065=CARTESIAN_POINT('Ctrl Pts',(0.404746659773314,-0.692356261122907,
-3.1062445835892));
#55066=CARTESIAN_POINT('Ctrl Pts',(0.515485612228519,-0.614370925825055,
-3.10096146015754));
#55067=CARTESIAN_POINT('Ctrl Pts',(0.600878459605494,-0.514675669986451,
-3.09567833672588));
#55068=CARTESIAN_POINT('Ctrl Pts',(0.686271306982469,-0.414980414147849,
-3.09039521329422));
#55069=CARTESIAN_POINT('Ctrl Pts',(0.746318049281215,-0.293575237768495,
-3.08511208986256));
#55070=CARTESIAN_POINT('Ctrl Pts',(0.773727606947812,-0.165201570030935,
-3.0798289664309));
#55071=CARTESIAN_POINT('Ctrl Pts',(0.801137164614409,-0.0368279022933761,
-3.07454584299924));
#55072=CARTESIAN_POINT('Ctrl Pts',(0.795909537648858,0.0985142568023888,
-3.06926271956758));
#55073=CARTESIAN_POINT('Ctrl Pts',(0.758679482286466,0.224391202259391,
-3.06397959613592));
#55074=CARTESIAN_POINT('Ctrl Pts',(0.721449426924073,0.350268147716393,
-3.05869647270426));
#55075=CARTESIAN_POINT('Ctrl Pts',(0.652216943164838,0.466679879534633,
-3.0534133492726));
#55076=CARTESIAN_POINT('Ctrl Pts',(0.559388474513935,0.559491289543318,
-3.04813022584094));
#55077=CARTESIAN_POINT('Ctrl Pts',(0.466560005863032,0.652302699552004,
-3.04284710240928));
#55078=CARTESIAN_POINT('Ctrl Pts',(0.350135552320461,0.721513787751136,
-3.03756397897762));
#55079=CARTESIAN_POINT('Ctrl Pts',(0.224251766772022,0.758720708557174,
-3.03228085554596));
#55080=CARTESIAN_POINT('Ctrl Pts',(0.0983679812235839,0.795927629363212,
-3.0269977321143));
#55081=CARTESIAN_POINT('Ctrl Pts',(-0.0369751363307216,0.801130382776156,
-3.02171460868264));
#55082=CARTESIAN_POINT('Ctrl Pts',(-0.165343764514632,0.773697232792003,
-3.01643148525098));
#55083=CARTESIAN_POINT('Ctrl Pts',(-0.293712392698542,0.746264082807851,
-3.01114836181932));
#55084=CARTESIAN_POINT('Ctrl Pts',(-0.415106531512058,0.686195029426602,
-3.00586523838766));
#55085=CARTESIAN_POINT('Ctrl Pts',(-0.514786091991394,0.600783861289651,
-3.000582114956));
#55086=CARTESIAN_POINT('Ctrl Pts',(-0.614465652470729,0.5153726931527,-2.99529899152434));
#55087=CARTESIAN_POINT('Ctrl Pts',(-0.692430634615885,0.404619410260047,
-2.99001586809268));
#55088=CARTESIAN_POINT('Ctrl Pts',(-0.739214265285162,0.281972052680388,
-2.98473274466102));
#55089=CARTESIAN_POINT('Ctrl Pts',(-0.773453550751941,0.192210787301005,
-2.98086621338191));
#55090=CARTESIAN_POINT('Ctrl Pts',(-0.790991297852172,0.0960787478750471,
-2.97699968210281));
#55091=CARTESIAN_POINT('Ctrl Pts',(-0.791084859053011,-2.00741357560715E-5,
-2.97313315082371));
#55092=CARTESIAN_POINT('Origin',(0.,0.,-1.94));
#55093=CARTESIAN_POINT('',(-0.791067783107607,1.83219459327505E-5,-2.7446668491763));
#55094=CARTESIAN_POINT('',(-0.79105596750504,1.59022465970799E-5,-2.77313315082371));
#55095=CARTESIAN_POINT('',(-0.7911,-9.68818082805471E-17,-1.94));
#55096=CARTESIAN_POINT('Ctrl Pts',(-0.791067783107607,1.83219459327505E-5,
-2.7446668491763));
#55097=CARTESIAN_POINT('Ctrl Pts',(-0.791103178687645,0.0412514554789803,
-2.74632575940143));
#55098=CARTESIAN_POINT('Ctrl Pts',(-0.787935332404873,0.0824792023563481,
-2.74798466962656));
#55099=CARTESIAN_POINT('Ctrl Pts',(-0.7815171568035,0.1231945830474,-2.74964357985169));
#55100=CARTESIAN_POINT('Ctrl Pts',(-0.761077223771279,0.252860660511613,
-2.75492670328335));
#55101=CARTESIAN_POINT('Ctrl Pts',(-0.707671529260795,0.377330174848837,
-2.76020982671501));
#55102=CARTESIAN_POINT('Ctrl Pts',(-0.62778477423003,0.481489614545734,
-2.76549295014667));
#55103=CARTESIAN_POINT('Ctrl Pts',(-0.547898019199265,0.585649054242631,
-2.77077607357833));
#55104=CARTESIAN_POINT('Ctrl Pts',(-0.441530203648218,0.669498419299202,
-2.77605919700999));
#55105=CARTESIAN_POINT('Ctrl Pts',(-0.321596869294389,0.722856434799122,
-2.78134232044165));
#55106=CARTESIAN_POINT('Ctrl Pts',(-0.201663534940562,0.776214450299041,
-2.78662544387331));
#55107=CARTESIAN_POINT('Ctrl Pts',(-0.0681646817839529,0.799081116242312,
-2.79190856730497));
#55108=CARTESIAN_POINT('Ctrl Pts',(0.0626898056511569,0.78867988432435,
-2.79719169073663));
#55109=CARTESIAN_POINT('Ctrl Pts',(0.193544293086269,0.778278652406388,
-2.80247481416829));
#55110=CARTESIAN_POINT('Ctrl Pts',(0.321754414799881,0.734609522627193,
-2.80775793759995));
#55111=CARTESIAN_POINT('Ctrl Pts',(0.431752462016372,0.662974949159658,
-2.81304106103161));
#55112=CARTESIAN_POINT('Ctrl Pts',(0.541750509232863,0.591340375692123,
-2.81832418446327));
#55113=CARTESIAN_POINT('Ctrl Pts',(0.633536481952231,0.491740358536247,
-2.82360730789493));
#55114=CARTESIAN_POINT('Ctrl Pts',(0.695965415378531,0.376268670324063,
-2.82889043132659));
#55115=CARTESIAN_POINT('Ctrl Pts',(0.758394348804829,0.260796982111881,
-2.83417355475825));
#55116=CARTESIAN_POINT('Ctrl Pts',(0.79146624293806,0.129453622843392,-2.83945667818991));
#55117=CARTESIAN_POINT('Ctrl Pts',(0.791165395978371,-0.00181325035172657,
-2.84473980162157));
#55118=CARTESIAN_POINT('Ctrl Pts',(0.790864549018682,-0.133080123546847,
-2.85002292505323));
#55119=CARTESIAN_POINT('Ctrl Pts',(0.757190960966073,-0.264270510668598,
-2.85530604848489));
#55120=CARTESIAN_POINT('Ctrl Pts',(0.694233393341295,-0.379454828985322,
-2.86058917191655));
#55121=CARTESIAN_POINT('Ctrl Pts',(0.631275825716517,-0.494639147302047,
-2.86587229534821));
#55122=CARTESIAN_POINT('Ctrl Pts',(0.53903427851957,-0.593817396813745,
-2.87115541877987));
#55123=CARTESIAN_POINT('Ctrl Pts',(0.428709033948005,-0.664947017349366,
-2.87643854221153));
#55124=CARTESIAN_POINT('Ctrl Pts',(0.31838378937644,-0.736076637884986,
-2.88172166564319));
#55125=CARTESIAN_POINT('Ctrl Pts',(0.189974847430256,-0.779157629444529,
-2.88700478907485));
#55126=CARTESIAN_POINT('Ctrl Pts',(0.0590740583135238,-0.788958951596863,
-2.89228791250651));
#55127=CARTESIAN_POINT('Ctrl Pts',(-0.0718267308032067,-0.798760273749196,
-2.89757103593817));
#55128=CARTESIAN_POINT('Ctrl Pts',(-0.205219367090492,-0.77528192649432,
-2.90285415936983));
#55129=CARTESIAN_POINT('Ctrl Pts',(-0.324906863237354,-0.721374730560832,
-2.90813728280149));
#55130=CARTESIAN_POINT('Ctrl Pts',(-0.444594359384217,-0.667467534627343,
-2.91342040623315));
#55131=CARTESIAN_POINT('Ctrl Pts',(-0.550576715390659,-0.583131490015245,
-2.91870352966481));
#55132=CARTESIAN_POINT('Ctrl Pts',(-0.629985193347303,-0.478606965926751,
-2.92398665309647));
#55133=CARTESIAN_POINT('Ctrl Pts',(-0.709393671303948,-0.374082441838257,
-2.92926977652813));
#55134=CARTESIAN_POINT('Ctrl Pts',(-0.762228271210791,-0.249369438273371,
-2.93455289995979));
#55135=CARTESIAN_POINT('Ctrl Pts',(-0.782073636357824,-0.119611032035093,
-2.93983602339145));
#55136=CARTESIAN_POINT('Ctrl Pts',(-0.788122425671071,-0.0800611797072125,
-2.94144629865307));
#55137=CARTESIAN_POINT('Ctrl Pts',(-0.79110649381175,-0.0400426062189334,
-2.94305657391468));
#55138=CARTESIAN_POINT('Ctrl Pts',(-0.791071031963789,-1.87933227643877E-5,
-2.9446668491763));
#55139=CARTESIAN_POINT('Ctrl Pts',(-0.791084859053011,-2.00741357560715E-5,
-2.97313315082371));
#55140=CARTESIAN_POINT('Ctrl Pts',(-0.791119137338463,-0.0352280751329303,
-2.97171655867115));
#55141=CARTESIAN_POINT('Ctrl Pts',(-0.788811898631655,-0.0704316173870898,
-2.9702999665186));
#55142=CARTESIAN_POINT('Ctrl Pts',(-0.784126621092215,-0.105315766095962,
-2.96888337436604));
#55143=CARTESIAN_POINT('Ctrl Pts',(-0.766653067036593,-0.235414795025995,
-2.96360025093438));
#55144=CARTESIAN_POINT('Ctrl Pts',(-0.71610367973195,-0.361071420619393,
-2.95831712750272));
#55145=CARTESIAN_POINT('Ctrl Pts',(-0.638616337606501,-0.467027988279004,
-2.95303400407106));
#55146=CARTESIAN_POINT('Ctrl Pts',(-0.561128995481052,-0.572984555938614,
-2.9477508806394));
#55147=CARTESIAN_POINT('Ctrl Pts',(-0.456703698534796,-0.659241065664438,
-2.94246775720774));
#55148=CARTESIAN_POINT('Ctrl Pts',(-0.338020121273455,-0.715323958852318,
-2.93718463377608));
#55149=CARTESIAN_POINT('Ctrl Pts',(-0.219336544012115,-0.771406852040197,
-2.93190151034442));
#55150=CARTESIAN_POINT('Ctrl Pts',(-0.0863946864356892,-0.797316128690136,
-2.92661838691276));
#55151=CARTESIAN_POINT('Ctrl Pts',(0.0446631992281643,-0.789905796363452,
-2.9213352634811));
#55152=CARTESIAN_POINT('Ctrl Pts',(0.17572108489202,-0.782495464036769,
-2.91605214004944));
#55153=CARTESIAN_POINT('Ctrl Pts',(0.304894998643301,-0.741765522733463,
-2.91076901661778));
#55154=CARTESIAN_POINT('Ctrl Pts',(0.416500204801163,-0.672661540371131,
-2.90548589318612));
#55155=CARTESIAN_POINT('Ctrl Pts',(0.528105410959024,-0.6035575580088,-2.90020276975446));
#55156=CARTESIAN_POINT('Ctrl Pts',(0.622141909523464,-0.506079534587444,
-2.8949196463228));
#55157=CARTESIAN_POINT('Ctrl Pts',(0.687191469200697,-0.392063583047012,
-2.88963652289114));
#55158=CARTESIAN_POINT('Ctrl Pts',(0.75224102887793,-0.27804763150658,-2.88435339945948));
#55159=CARTESIAN_POINT('Ctrl Pts',(0.788303649667956,-0.147493751847073,
-2.87907027602782));
#55160=CARTESIAN_POINT('Ctrl Pts',(0.791000485574522,-0.0162542399005356,
-2.87378715259616));
#55161=CARTESIAN_POINT('Ctrl Pts',(0.793697321481088,0.114985272046,-2.8685040291645));
#55162=CARTESIAN_POINT('Ctrl Pts',(0.763028372504193,0.246910416279567,
-2.86322090573284));
#55163=CARTESIAN_POINT('Ctrl Pts',(0.702717566674989,0.363502393362486,
-2.85793778230118));
#55164=CARTESIAN_POINT('Ctrl Pts',(0.642406760845787,0.480094370445405,
-2.85265465886952));
#55165=CARTESIAN_POINT('Ctrl Pts',(0.552454098164276,0.581353180377678,
-2.84737153543785));
#55166=CARTESIAN_POINT('Ctrl Pts',(0.443781936690031,0.654983634269986,
-2.84208841200619));
#55167=CARTESIAN_POINT('Ctrl Pts',(0.335109775215785,0.728614088162294,
-2.83680528857453));
#55168=CARTESIAN_POINT('Ctrl Pts',(0.207718114948804,0.774616186014636,
-2.83152216514288));
#55169=CARTESIAN_POINT('Ctrl Pts',(0.0770752842938398,0.787404196740719,
-2.82623904171122));
#55170=CARTESIAN_POINT('Ctrl Pts',(-0.0535675463611245,0.800192207466803,
-2.82095591827956));
#55171=CARTESIAN_POINT('Ctrl Pts',(-0.187461547404071,0.779766131066627,
-2.8156727948479));
#55172=CARTESIAN_POINT('Ctrl Pts',(-0.308348854111219,0.728606171166682,
-2.81038967141623));
#55173=CARTESIAN_POINT('Ctrl Pts',(-0.429236160818364,0.677446211266737,
-2.80510654798457));
#55174=CARTESIAN_POINT('Ctrl Pts',(-0.537116773189712,0.595552367867022,
-2.79982342455292));
#55175=CARTESIAN_POINT('Ctrl Pts',(-0.618891460575715,0.4928684697973,-2.79454030112126));
#55176=CARTESIAN_POINT('Ctrl Pts',(-0.700666147961719,0.390184571727577,
-2.7892571776896));
#55177=CARTESIAN_POINT('Ctrl Pts',(-0.756334910362378,0.266710618987845,
-2.78397405425794));
#55178=CARTESIAN_POINT('Ctrl Pts',(-0.779138257424125,0.137439238618277,
-2.77869093082627));
#55179=CARTESIAN_POINT('Ctrl Pts',(-0.787134536388695,0.0921086116374632,
-2.77683833749209));
#55180=CARTESIAN_POINT('Ctrl Pts',(-0.791089545934546,0.0460651086212764,
-2.7749857441579));
#55181=CARTESIAN_POINT('Ctrl Pts',(-0.79105596750504,1.59022465970799E-5,
-2.77313315082371));
#55182=CARTESIAN_POINT('Origin',(0.,0.,-1.94));
#55183=CARTESIAN_POINT('',(-0.791159134504794,-8.93421506220626E-6,-2.5446668491763));
#55184=CARTESIAN_POINT('',(-0.791165616430847,-4.19399107163473E-6,-2.57313315082371));
#55185=CARTESIAN_POINT('',(-0.7911,-9.68818082805471E-17,-1.94));
#55186=CARTESIAN_POINT('Ctrl Pts',(-0.791159134504794,-8.93421506220626E-6,
-2.5446668491763));
#55187=CARTESIAN_POINT('Ctrl Pts',(-0.791088724556594,0.12244083710649,
-2.54959494488817));
#55188=CARTESIAN_POINT('Ctrl Pts',(-0.762201994881393,0.244922676356341,
-2.55452304060005));
#55189=CARTESIAN_POINT('Ctrl Pts',(-0.70735329025823,0.354397085810968,
-2.55945113631192));
#55190=CARTESIAN_POINT('Ctrl Pts',(-0.64855319920225,0.47175820287759,-2.56473425974358));
#55191=CARTESIAN_POINT('Ctrl Pts',(-0.559915708359819,0.574170230602118,
-2.57001738317524));
#55192=CARTESIAN_POINT('Ctrl Pts',(-0.452203483155427,0.649197952471008,
-2.5753005066069));
#55193=CARTESIAN_POINT('Ctrl Pts',(-0.344491257951037,0.724225674339897,
-2.58058363003856));
#55194=CARTESIAN_POINT('Ctrl Pts',(-0.217704298384688,0.771869090353149,
-2.58586675347022));
#55195=CARTESIAN_POINT('Ctrl Pts',(-0.0872375080466301,0.786343174994394,
-2.59114987690188));
#55196=CARTESIAN_POINT('Ctrl Pts',(0.0432292822914291,0.800817259635639,
-2.59643300033354));
#55197=CARTESIAN_POINT('Ctrl Pts',(0.177375903401196,0.782122012904877,
-2.6017161237652));
#55198=CARTESIAN_POINT('Ctrl Pts',(0.298913816571699,0.732527475206897,
-2.60699924719686));
#55199=CARTESIAN_POINT('Ctrl Pts',(0.420451729742201,0.682932937508916,
-2.61228237062852));
#55200=CARTESIAN_POINT('Ctrl Pts',(0.52938093497344,0.602439108843718,-2.61756549406018));
#55201=CARTESIAN_POINT('Ctrl Pts',(0.612474877906563,0.50081982349323,-2.62284861749184));
#55202=CARTESIAN_POINT('Ctrl Pts',(0.695568820839685,0.399200538142744,
-2.6281317409235));
#55203=CARTESIAN_POINT('Ctrl Pts',(0.752827501474693,0.276455796106968,
-2.63341486435516));
#55204=CARTESIAN_POINT('Ctrl Pts',(0.777298376181737,0.14748968118375,-2.63869798778682));
#55205=CARTESIAN_POINT('Ctrl Pts',(0.801769250888782,0.018523566260528,
-2.64398111121848));
#55206=CARTESIAN_POINT('Ctrl Pts',(0.793452319667862,-0.116663921550136,
-2.64926423465014));
#55207=CARTESIAN_POINT('Ctrl Pts',(0.75335745257778,-0.241657857964453,
-2.6545473580818));
#55208=CARTESIAN_POINT('Ctrl Pts',(0.713262585487699,-0.366651794378766,
-2.65983048151346));
#55209=CARTESIAN_POINT('Ctrl Pts',(0.641389782528459,-0.481452179396731,
-2.66511360494513));
#55210=CARTESIAN_POINT('Ctrl Pts',(0.546466083737166,-0.572119560053153,
-2.67039672837679));
#55211=CARTESIAN_POINT('Ctrl Pts',(0.451542384945872,-0.662786940709577,
-2.67567985180845));
#55212=CARTESIAN_POINT('Ctrl Pts',(0.333567790322526,-0.729321317004456,
-2.6809629752401));
#55213=CARTESIAN_POINT('Ctrl Pts',(0.206867176152018,-0.763643858812038,
-2.68624609867176));
#55214=CARTESIAN_POINT('Ctrl Pts',(0.0801665619815108,-0.79796640061962,
-2.69152922210342));
#55215=CARTESIAN_POINT('Ctrl Pts',(-0.055260071736158,-0.800077107939904,
-2.69681234553509));
#55216=CARTESIAN_POINT('Ctrl Pts',(-0.182968762808292,-0.769719691515588,
-2.70209546896675));
#55217=CARTESIAN_POINT('Ctrl Pts',(-0.310677453880424,-0.739362275091273,
-2.70737859239841));
#55218=CARTESIAN_POINT('Ctrl Pts',(-0.430668202307021,-0.676536734922358,
-2.71266171583007));
#55219=CARTESIAN_POINT('Ctrl Pts',(-0.528371323555323,-0.588871561645531,
-2.71794483926173));
#55220=CARTESIAN_POINT('Ctrl Pts',(-0.626074444803625,-0.501206388368703,
-2.72322796269339));
#55221=CARTESIAN_POINT('Ctrl Pts',(-0.701489938873631,-0.388701581983963,
-2.72851108612505));
#55222=CARTESIAN_POINT('Ctrl Pts',(-0.745460600131655,-0.265017858495993,
-2.73379420955671));
#55223=CARTESIAN_POINT('Ctrl Pts',(-0.77562439495731,-0.180171045829891,
-2.73741842276324));
#55224=CARTESIAN_POINT('Ctrl Pts',(-0.790990454553786,-0.0900635069760673,
-2.74104263596977));
#55225=CARTESIAN_POINT('Ctrl Pts',(-0.791067783107607,1.83219459327505E-5,
-2.7446668491763));
#55226=CARTESIAN_POINT('Ctrl Pts',(-0.79105596750504,1.59022465970799E-5,
-2.77313315082371));
#55227=CARTESIAN_POINT('Ctrl Pts',(-0.790993788822369,-0.0852554768075867,
-2.76970262072624));
#55228=CARTESIAN_POINT('Ctrl Pts',(-0.777254906090452,-0.170546412443365,
-2.76627209062877));
#55229=CARTESIAN_POINT('Ctrl Pts',(-0.750173823124674,-0.251366671602233,
-2.7628415605313));
#55230=CARTESIAN_POINT('Ctrl Pts',(-0.70846811004064,-0.375832393453771,
-2.75755843709963));
#55231=CARTESIAN_POINT('Ctrl Pts',(-0.635118752149737,-0.489695029157441,
-2.75227531366797));
#55232=CARTESIAN_POINT('Ctrl Pts',(-0.539032077807812,-0.579128990457279,
-2.74699219023631));
#55233=CARTESIAN_POINT('Ctrl Pts',(-0.442945403465885,-0.668562951757118,
-2.74170906680465));
#55234=CARTESIAN_POINT('Ctrl Pts',(-0.324121412672936,-0.733568238653124,
-2.73642594337299));
#55235=CARTESIAN_POINT('Ctrl Pts',(-0.196988118283939,-0.766251688251861,
-2.73114281994133));
#55236=CARTESIAN_POINT('Ctrl Pts',(-0.0698548238949439,-0.798935137850597,
-2.72585969650967));
#55237=CARTESIAN_POINT('Ctrl Pts',(0.0655877740900931,-0.799296750152065,
-2.72057657307801));
#55238=CARTESIAN_POINT('Ctrl Pts',(0.192893775042879,-0.76729261696147,
-2.71529344964635));
#55239=CARTESIAN_POINT('Ctrl Pts',(0.320199775995663,-0.735288483770875,
-2.71001032621469));
#55240=CARTESIAN_POINT('Ctrl Pts',(0.439369179916195,-0.670918605088214,
-2.70472720278303));
#55241=CARTESIAN_POINT('Ctrl Pts',(0.535932032713452,-0.581998990381858,
-2.69944407935137));
#55242=CARTESIAN_POINT('Ctrl Pts',(0.632494885510708,-0.493079375675501,
-2.69416095591971));
#55243=CARTESIAN_POINT('Ctrl Pts',(0.706451187184694,-0.379610024945445,
-2.68887783248805));
#55244=CARTESIAN_POINT('Ctrl Pts',(0.748820912202367,-0.255368772449351,
-2.68359470905639));
#55245=CARTESIAN_POINT('Ctrl Pts',(0.791190637220041,-0.131127519953255,
-2.67831158562473));
#55246=CARTESIAN_POINT('Ctrl Pts',(0.801973785581401,0.0038856343088754,
-2.67302846219307));
#55247=CARTESIAN_POINT('Ctrl Pts',(0.77986103075957,0.133276934225298,-2.66774533876141));
#55248=CARTESIAN_POINT('Ctrl Pts',(0.757748275937739,0.26266823414172,-2.66246221532975));
#55249=CARTESIAN_POINT('Ctrl Pts',(0.702739617932715,0.38643767971243,-2.65717909189809));
#55250=CARTESIAN_POINT('Ctrl Pts',(0.621514394978597,0.489556764153312,
-2.65189596846643));
#55251=CARTESIAN_POINT('Ctrl Pts',(0.540289172024479,0.592675848594195,
-2.64661284503477));
#55252=CARTESIAN_POINT('Ctrl Pts',(0.432847384121266,0.67514457190525,-2.64132972160311));
#55253=CARTESIAN_POINT('Ctrl Pts',(0.312234978359981,0.726949301383814,
-2.63604659817145));
#55254=CARTESIAN_POINT('Ctrl Pts',(0.191622572598698,0.778754030862378,
-2.63076347473979));
#55255=CARTESIAN_POINT('Ctrl Pts',(0.0578395489793438,0.799894766508452,
-2.62548035130813));
#55256=CARTESIAN_POINT('Ctrl Pts',(-0.0728697030302944,0.787804528340724,
-2.62019722787647));
#55257=CARTESIAN_POINT('Ctrl Pts',(-0.203578955039934,0.775714290172996,
-2.61491410444481));
#55258=CARTESIAN_POINT('Ctrl Pts',(-0.331214435439859,0.730393078191463,
-2.60963098101315));
#55259=CARTESIAN_POINT('Ctrl Pts',(-0.440278210356008,0.657343948005596,
-2.60434785758149));
#55260=CARTESIAN_POINT('Ctrl Pts',(-0.549341985272158,0.584294817819729,
-2.59906473414983));
#55261=CARTESIAN_POINT('Ctrl Pts',(-0.639834054704532,0.483517769429526,
-2.59378161071817));
#55262=CARTESIAN_POINT('Ctrl Pts',(-0.700766563992376,0.367249494600322,
-2.58849848728651));
#55263=CARTESIAN_POINT('Ctrl Pts',(-0.759838217269807,0.254532009334278,
-2.58337670846557));
#55264=CARTESIAN_POINT('Ctrl Pts',(-0.79112821691516,0.127255041952799,
-2.57825492964464));
#55265=CARTESIAN_POINT('Ctrl Pts',(-0.791165616430847,-4.19399107163473E-6,
-2.57313315082371));
#55266=CARTESIAN_POINT('Origin',(0.,0.,-1.94));
#55267=CARTESIAN_POINT('',(-0.791035698195336,-6.17953886133949E-6,-2.3446668491763));
#55268=CARTESIAN_POINT('',(-0.791041154687578,-1.02586427583964E-5,-2.3731331508237));
#55269=CARTESIAN_POINT('',(-0.7911,-9.68818082805471E-17,-1.94));
#55270=CARTESIAN_POINT('Ctrl Pts',(-0.791035698195336,-6.17953886133949E-6,
-2.3446668491763));
#55271=CARTESIAN_POINT('Ctrl Pts',(-0.791015846145582,0.0724352453097401,
-2.34758100694326));
#55272=CARTESIAN_POINT('Ctrl Pts',(-0.7811516579661,0.144881969211618,-2.35049516471022));
#55273=CARTESIAN_POINT('Ctrl Pts',(-0.761514037378075,0.214574794760694,
-2.35340932247718));
#55274=CARTESIAN_POINT('Ctrl Pts',(-0.725912679535712,0.340922037813706,
-2.35869244590884));
#55275=CARTESIAN_POINT('Ctrl Pts',(-0.65818932680173,0.458218140476839,
-2.3639755693405));
#55276=CARTESIAN_POINT('Ctrl Pts',(-0.566567178862551,0.552220611265262,
-2.36925869277216));
#55277=CARTESIAN_POINT('Ctrl Pts',(-0.474945030923373,0.646223082053685,
-2.37454181620382));
#55278=CARTESIAN_POINT('Ctrl Pts',(-0.359424087778997,0.716931920967397,
-2.37982493963548));
#55279=CARTESIAN_POINT('Ctrl Pts',(-0.234031295011568,0.755761420440113,
-2.38510806306714));
#55280=CARTESIAN_POINT('Ctrl Pts',(-0.108638502244139,0.794590919912829,
-2.3903911864988));
#55281=CARTESIAN_POINT('Ctrl Pts',(0.0266261401463434,0.801541079944549,
-2.39567430993046));
#55282=CARTESIAN_POINT('Ctrl Pts',(0.155338339504752,0.775767988480032,
-2.40095743336212));
#55283=CARTESIAN_POINT('Ctrl Pts',(0.284050538863158,0.749994897015517,
-2.40624055679378));
#55284=CARTESIAN_POINT('Ctrl Pts',(0.406210295189492,0.691498554054766,
-2.41152368022544));
#55285=CARTESIAN_POINT('Ctrl Pts',(0.506984555639162,0.607381784394141,
-2.4168068036571));
#55286=CARTESIAN_POINT('Ctrl Pts',(0.607758816088832,0.523265014733517,
-2.42208992708876));
#55287=CARTESIAN_POINT('Ctrl Pts',(0.687147580661839,0.413527818373018,
-2.42737305052042));
#55288=CARTESIAN_POINT('Ctrl Pts',(0.735511195714536,0.291494858700841,
-2.43265617395208));
#55289=CARTESIAN_POINT('Ctrl Pts',(0.783874810767234,0.16946189902866,-2.43793929738374));
#55290=CARTESIAN_POINT('Ctrl Pts',(0.80121327629962,0.035133176044802,-2.4432224208154));
#55291=CARTESIAN_POINT('Ctrl Pts',(0.785421296891827,-0.0951806601112308,
-2.44850554424706));
#55292=CARTESIAN_POINT('Ctrl Pts',(0.769629317484034,-0.22549449626726,
-2.45378866767872));
#55293=CARTESIAN_POINT('Ctrl Pts',(0.720706893136064,-0.351793445595463,
-2.45907179111038));
#55294=CARTESIAN_POINT('Ctrl Pts',(0.644594350903746,-0.458741860367493,
-2.46435491454204));
#55295=CARTESIAN_POINT('Ctrl Pts',(0.568481808671427,-0.565690275139524,
-2.4696380379737));
#55296=CARTESIAN_POINT('Ctrl Pts',(0.465179148554758,-0.653288155355381,
-2.47492116140536));
#55297=CARTESIAN_POINT('Ctrl Pts',(0.347229730679673,-0.710899068646577,
-2.48020428483702));
#55298=CARTESIAN_POINT('Ctrl Pts',(0.229280312804588,-0.768509981937773,
-2.48548740826868));
#55299=CARTESIAN_POINT('Ctrl Pts',(0.0966841371710874,-0.796133928304308,
-2.49077053170034));
#55300=CARTESIAN_POINT('Ctrl Pts',(-0.0344585178696828,-0.790416714282204,
-2.496053655132));
#55301=CARTESIAN_POINT('Ctrl Pts',(-0.165601172910451,-0.784699500260099,
-2.50133677856366));
#55302=CARTESIAN_POINT('Ctrl Pts',(-0.295290307358489,-0.745641125849356,
-2.50661990199532));
#55303=CARTESIAN_POINT('Ctrl Pts',(-0.407778625684669,-0.677984191633678,
-2.51190302542698));
#55304=CARTESIAN_POINT('Ctrl Pts',(-0.520266944010852,-0.610327257417999,
-2.51718614885864));
#55305=CARTESIAN_POINT('Ctrl Pts',(-0.615554446215177,-0.514071763397382,
-2.5224692722903));
#55306=CARTESIAN_POINT('Ctrl Pts',(-0.682070999889633,-0.40090537883646,
-2.52775239572196));
#55307=CARTESIAN_POINT('Ctrl Pts',(-0.748587553564088,-0.28773899427554,
-2.53303551915362));
#55308=CARTESIAN_POINT('Ctrl Pts',(-0.786333158708677,-0.157661719174315,
-2.53831864258528));
#55309=CARTESIAN_POINT('Ctrl Pts',(-0.790724615646208,-0.0264679784193449,
-2.54360176601694));
#55310=CARTESIAN_POINT('Ctrl Pts',(-0.79101972306954,-0.017651713716691,
-2.54395679373673));
#55311=CARTESIAN_POINT('Ctrl Pts',(-0.791164206947543,-0.00883040718193987,
-2.54431182145651));
#55312=CARTESIAN_POINT('Ctrl Pts',(-0.791159134504794,-8.93421506220626E-6,
-2.5446668491763));
#55313=CARTESIAN_POINT('Ctrl Pts',(-0.791165616430847,-4.19399107163473E-6,
-2.57313315082371));
#55314=CARTESIAN_POINT('Ctrl Pts',(-0.791166794578228,-0.00401307305485152,
-2.57297180621298));
#55315=CARTESIAN_POINT('Ctrl Pts',(-0.791136959035539,-0.00802193452274154,
-2.57281046160226));
#55316=CARTESIAN_POINT('Ctrl Pts',(-0.791076001298007,-0.0120303226984998,
-2.57264911699153));
#55317=CARTESIAN_POINT('Ctrl Pts',(-0.789079980172478,-0.143282363899915,
-2.56736599355987));
#55318=CARTESIAN_POINT('Ctrl Pts',(-0.753714988778105,-0.274026945034545,
-2.56208287012821));
#55319=CARTESIAN_POINT('Ctrl Pts',(-0.689275164578622,-0.388388614649023,
-2.55679974669655));
#55320=CARTESIAN_POINT('Ctrl Pts',(-0.624835340379137,-0.502750284263503,
-2.55151662326489));
#55321=CARTESIAN_POINT('Ctrl Pts',(-0.531320683374539,-0.600729042357833,
-2.54623349983323));
#55322=CARTESIAN_POINT('Ctrl Pts',(-0.420086061082635,-0.670427975086027,
-2.54095037640157));
#55323=CARTESIAN_POINT('Ctrl Pts',(-0.308851438790733,-0.74012690781422,
-2.53566725296991));
#55324=CARTESIAN_POINT('Ctrl Pts',(-0.179896851211523,-0.781546015176281,
-2.53038412953825));
#55325=CARTESIAN_POINT('Ctrl Pts',(-0.0488804026965334,-0.789656048369224,
-2.52510100610659));
#55326=CARTESIAN_POINT('Ctrl Pts',(0.0821360458184596,-0.797766081562167,
-2.51981788267493));
#55327=CARTESIAN_POINT('Ctrl Pts',(0.215214355269229,-0.772567040585991,
-2.51453475924327));
#55328=CARTESIAN_POINT('Ctrl Pts',(0.334195704977728,-0.717118678649715,
-2.50925163581161));
#55329=CARTESIAN_POINT('Ctrl Pts',(0.453177054686225,-0.66167031671344,
-2.50396851237995));
#55330=CARTESIAN_POINT('Ctrl Pts',(0.558061444652449,-0.575972633817065,
-2.49868538894829));
#55331=CARTESIAN_POINT('Ctrl Pts',(0.636113455735699,-0.470431333911614,
-2.49340226551663));
#55332=CARTESIAN_POINT('Ctrl Pts',(0.714165466818948,-0.364890034006163,
-2.48811914208497));
#55333=CARTESIAN_POINT('Ctrl Pts',(0.765385099019224,-0.239505117091636,
-2.48283601865331));
#55334=CARTESIAN_POINT('Ctrl Pts',(0.783553090494863,-0.109501245973838,
-2.47755289522165));
#55335=CARTESIAN_POINT('Ctrl Pts',(0.801721081970502,0.0205026251439623,
-2.47226977178999));
#55336=CARTESIAN_POINT('Ctrl Pts',(0.786837432721503,0.155125450465034,
-2.46698664835833));
#55337=CARTESIAN_POINT('Ctrl Pts',(0.740709366030476,0.278020868944409,
-2.46170352492667));
#55338=CARTESIAN_POINT('Ctrl Pts',(0.69458129933945,0.40091628742378,-2.45642040149501));
#55339=CARTESIAN_POINT('Ctrl Pts',(0.617208815206396,0.512084299061456,
-2.45113727806335));
#55340=CARTESIAN_POINT('Ctrl Pts',(0.517986743650434,0.59802650601482,-2.44585415463169));
#55341=CARTESIAN_POINT('Ctrl Pts',(0.418764672094471,0.683968712968185,
-2.44057103120003));
#55342=CARTESIAN_POINT('Ctrl Pts',(0.297693013115599,0.74468511523724,-2.43528790776837));
#55343=CARTESIAN_POINT('Ctrl Pts',(0.169472699079944,0.772803320878238,
-2.43000478433671));
#55344=CARTESIAN_POINT('Ctrl Pts',(0.0412523850442884,0.800921526519236,
-2.42472166090505));
#55345=CARTESIAN_POINT('Ctrl Pts',(-0.0941165840481511,0.796441535532177,
-2.41943853747339));
#55346=CARTESIAN_POINT('Ctrl Pts',(-0.220197247839481,0.759907323650583,
-2.41415541404173));
#55347=CARTESIAN_POINT('Ctrl Pts',(-0.346277911630814,0.723373111768988,
-2.40887229061007));
#55348=CARTESIAN_POINT('Ctrl Pts',(-0.463070270121033,0.654784678992858,
-2.40358916717841));
#55349=CARTESIAN_POINT('Ctrl Pts',(-0.55639299815506,0.562470265967808,
-2.39830604374674));
#55350=CARTESIAN_POINT('Ctrl Pts',(-0.649715726189086,0.47015585294276,
-2.39302292031508));
#55351=CARTESIAN_POINT('Ctrl Pts',(-0.719568823766917,0.354115459668794,
-2.38773979688343));
#55352=CARTESIAN_POINT('Ctrl Pts',(-0.757470490344006,0.228439105128446,
-2.38245667345177));
#55353=CARTESIAN_POINT('Ctrl Pts',(-0.779766457905857,0.154508954367816,
-2.37934883257575));
#55354=CARTESIAN_POINT('Ctrl Pts',(-0.791005704550203,0.0772443008585653,
-2.37624099169973));
#55355=CARTESIAN_POINT('Ctrl Pts',(-0.791041154687578,-1.02586427583964E-5,
-2.3731331508237));
#55356=CARTESIAN_POINT('Origin',(0.,0.,-1.94));
#55357=CARTESIAN_POINT('',(-0.791124794068662,1.84093985718808E-5,-2.1446668491763));
#55358=CARTESIAN_POINT('',(-0.791109792329072,1.99241595253492E-5,-2.17313315082371));
#55359=CARTESIAN_POINT('',(-0.7911,-9.68818082805471E-17,-1.94));
#55360=CARTESIAN_POINT('Ctrl Pts',(-0.791124794068662,1.84093985718808E-5,
-2.1446668491763));
#55361=CARTESIAN_POINT('Ctrl Pts',(-0.791147010981146,0.0223892334141203,
-2.14556706899834));
#55362=CARTESIAN_POINT('Ctrl Pts',(-0.790217040500928,0.0447582160969252,
-2.14646728882039));
#55363=CARTESIAN_POINT('Ctrl Pts',(-0.788321589215395,0.0670450866757845,
-2.14736750864243));
#55364=CARTESIAN_POINT('Ctrl Pts',(-0.777197747177103,0.197840127276048,
-2.15265063207409));
#55365=CARTESIAN_POINT('Ctrl Pts',(-0.732821120792358,0.325807088778621,
-2.15793375550575));
#55366=CARTESIAN_POINT('Ctrl Pts',(-0.660580070876739,0.435407787747225,
-2.16321687893741));
#55367=CARTESIAN_POINT('Ctrl Pts',(-0.58833902096112,0.545008486715829,
-2.16850000236907));
#55368=CARTESIAN_POINT('Ctrl Pts',(-0.488233547514627,0.636242923150465,
-2.17378312580073));
#55369=CARTESIAN_POINT('Ctrl Pts',(-0.372418797390191,0.698033101665596,
-2.17906624923239));
#55370=CARTESIAN_POINT('Ctrl Pts',(-0.256604047265758,0.759823280180726,
-2.18434937266405));
#55371=CARTESIAN_POINT('Ctrl Pts',(-0.125080020463381,0.792169200776354,
-2.18963249609571));
#55372=CARTESIAN_POINT('Ctrl Pts',(0.00618318862119299,0.791143311827209,
-2.19491561952737));
#55373=CARTESIAN_POINT('Ctrl Pts',(0.13744639770577,0.790117422878065,-2.20019874295903));
#55374=CARTESIAN_POINT('Ctrl Pts',(0.26844878907254,0.755719724384149,-2.20548186639069));
#55375=CARTESIAN_POINT('Ctrl Pts',(0.383283607073439,0.692126901817306,
-2.21076498982235));
#55376=CARTESIAN_POINT('Ctrl Pts',(0.498118425074332,0.628534079250467,
-2.21604811325401));
#55377=CARTESIAN_POINT('Ctrl Pts',(0.596785669709354,0.535746132610701,
-2.22133123668567));
#55378=CARTESIAN_POINT('Ctrl Pts',(0.667304828756521,0.425029689773172,
-2.22661436011733));
#55379=CARTESIAN_POINT('Ctrl Pts',(0.737823987803694,0.314313246935636,
-2.23189748354899));
#55380=CARTESIAN_POINT('Ctrl Pts',(0.780195061263012,0.185668307900335,
-2.23718060698065));
#55381=CARTESIAN_POINT('Ctrl Pts',(0.789273209372148,0.0547153784400642,
-2.24246373041231));
#55382=CARTESIAN_POINT('Ctrl Pts',(0.798351357481284,-0.0762375510202047,
-2.24774685384397));
#55383=CARTESIAN_POINT('Ctrl Pts',(0.774136580240238,-0.209498470905439,
-2.25302997727563));
#55384=CARTESIAN_POINT('Ctrl Pts',(0.719569118209714,-0.32888638735792,
-2.25831310070729));
#55385=CARTESIAN_POINT('Ctrl Pts',(0.665001656179192,-0.448274303810399,
-2.26359622413895));
#55386=CARTESIAN_POINT('Ctrl Pts',(0.580081509359193,-0.553789216830127,
-2.26887934757061));
#55387=CARTESIAN_POINT('Ctrl Pts',(0.475119970627436,-0.632619147024047,
-2.27416247100227));
#55388=CARTESIAN_POINT('Ctrl Pts',(0.370158431895679,-0.711449077217968,
-2.27944559443393));
#55389=CARTESIAN_POINT('Ctrl Pts',(0.245155501252162,-0.763594024586081,
-2.2847287178656));
#55390=CARTESIAN_POINT('Ctrl Pts',(0.115289459431262,-0.782722372373818,
-2.29001184129726));
#55391=CARTESIAN_POINT('Ctrl Pts',(-0.0145765823896404,-0.801850720161556,
-2.29529496472892));
#55392=CARTESIAN_POINT('Ctrl Pts',(-0.149305735387928,-0.787962468368917,
-2.30057808816058));
#55393=CARTESIAN_POINT('Ctrl Pts',(-0.272538727850647,-0.74274397573592,
-2.30586121159224));
#55394=CARTESIAN_POINT('Ctrl Pts',(-0.395771720313366,-0.697525483102923,
-2.3111443350239));
#55395=CARTESIAN_POINT('Ctrl Pts',(-0.507508552240518,-0.620976749629566,
-2.31642745845556));
#55396=CARTESIAN_POINT('Ctrl Pts',(-0.59418175769647,-0.522392582729869,
-2.32171058188722));
#55397=CARTESIAN_POINT('Ctrl Pts',(-0.680854963152421,-0.423808415830174,
-2.32699370531888));
#55398=CARTESIAN_POINT('Ctrl Pts',(-0.742464542137174,-0.303188815504138,
-2.33227682875054));
#55399=CARTESIAN_POINT('Ctrl Pts',(-0.771529650154178,-0.175179823619676,
-2.3375599521822));
#55400=CARTESIAN_POINT('Ctrl Pts',(-0.784562516757381,-0.11778027381361,
-2.3399289178469));
#55401=CARTESIAN_POINT('Ctrl Pts',(-0.791051836245505,-0.0588949775696238,
-2.3422978835116));
#55402=CARTESIAN_POINT('Ctrl Pts',(-0.791035698195336,-6.17953886133949E-6,
-2.3446668491763));
#55403=CARTESIAN_POINT('Ctrl Pts',(-0.791041154687578,-1.02586427583964E-5,
-2.3731331508237));
#55404=CARTESIAN_POINT('Ctrl Pts',(-0.791065967433308,-0.0540833281243991,
-2.37095786826806));
#55405=CARTESIAN_POINT('Ctrl Pts',(-0.785601959816742,-0.108151452479073,
-2.36878258571242));
#55406=CARTESIAN_POINT('Ctrl Pts',(-0.774598699244007,-0.161067760968372,
-2.36660730315678));
#55407=CARTESIAN_POINT('Ctrl Pts',(-0.747875005990574,-0.289585956718112,
-2.36132417972512));
#55408=CARTESIAN_POINT('Ctrl Pts',(-0.68847738390736,-0.411310032410861,
-2.35604105629347));
#55409=CARTESIAN_POINT('Ctrl Pts',(-0.6036180941653,-0.511459837025474,
-2.35075793286181));
#55410=CARTESIAN_POINT('Ctrl Pts',(-0.518758804423239,-0.611609641640088,
-2.34547480943015));
#55411=CARTESIAN_POINT('Ctrl Pts',(-0.408437847022332,-0.690185175176567,
-2.34019168599848));
#55412=CARTESIAN_POINT('Ctrl Pts',(-0.286050767600555,-0.737645529267958,
-2.33490856256682));
#55413=CARTESIAN_POINT('Ctrl Pts',(-0.163663688178782,-0.785105883359348,
-2.32962543913516));
#55414=CARTESIAN_POINT('Ctrl Pts',(-0.0292104867361406,-0.801451058005654,
-2.32434231570351));
#55415=CARTESIAN_POINT('Ctrl Pts',(0.100983071990288,-0.784696366542676,
-2.31905919227185));
#55416=CARTESIAN_POINT('Ctrl Pts',(0.231176630716716,-0.767941675079698,
-2.31377606884019));
#55417=CARTESIAN_POINT('Ctrl Pts',(0.357110546726931,-0.718087117507435,
-2.30849294540852));
#55418=CARTESIAN_POINT('Ctrl Pts',(0.463493495878834,-0.641186203666213,
-2.30320982197686));
#55419=CARTESIAN_POINT('Ctrl Pts',(0.569876445030741,-0.564285289824989,
-2.2979266985452));
#55420=CARTESIAN_POINT('Ctrl Pts',(0.656708427324334,-0.460338019714802,
-2.29264357511354));
#55421=CARTESIAN_POINT('Ctrl Pts',(0.713446008320202,-0.341966024198084,
-2.28736045168189));
#55422=CARTESIAN_POINT('Ctrl Pts',(0.770183589316067,-0.223594028681369,
-2.28207732825022));
#55423=CARTESIAN_POINT('Ctrl Pts',(0.796826769014208,-0.0907973077581235,
-2.27679420481856));
#55424=CARTESIAN_POINT('Ctrl Pts',(0.790140441973232,0.040299509329755,
-2.2715110813869));
#55425=CARTESIAN_POINT('Ctrl Pts',(0.783454114932256,0.171396326417634,
-2.26622795795524));
#55426=CARTESIAN_POINT('Ctrl Pts',(0.743438281152164,0.300793239670145,
-2.26094483452358));
#55427=CARTESIAN_POINT('Ctrl Pts',(0.674951799187771,0.412778436049007,
-2.25566171109192));
#55428=CARTESIAN_POINT('Ctrl Pts',(0.606465317223377,0.524763632427871,
-2.25037858766026));
#55429=CARTESIAN_POINT('Ctrl Pts',(0.509508187074682,0.619337111933087,
-2.2450954642286));
#55430=CARTESIAN_POINT('Ctrl Pts',(0.395853273049907,0.685015441219794,
-2.23981234079694));
#55431=CARTESIAN_POINT('Ctrl Pts',(0.282198359025133,0.750693770506501,
-2.23452921736528));
#55432=CARTESIAN_POINT('Ctrl Pts',(0.151845661124279,0.787476949574701,
-2.22924609393362));
#55433=CARTESIAN_POINT('Ctrl Pts',(0.0206230470064235,0.790898639792764,
-2.22396297050196));
#55434=CARTESIAN_POINT('Ctrl Pts',(-0.110599567111434,0.794320330010827,
-2.2186798470703));
#55435=CARTESIAN_POINT('Ctrl Pts',(-0.242692097446293,0.764380531378753,
-2.21339672363864));
#55436=CARTESIAN_POINT('Ctrl Pts',(-0.359615419971102,0.704714636014381,
-2.20811360020698));
#55437=CARTESIAN_POINT('Ctrl Pts',(-0.476538742495907,0.64504874065001,
-2.20283047677532));
#55438=CARTESIAN_POINT('Ctrl Pts',(-0.578292857210662,0.555656748553344,
-2.19754735334366));
#55439=CARTESIAN_POINT('Ctrl Pts',(-0.652522433635772,0.447392939255776,
-2.192264229912));
#55440=CARTESIAN_POINT('Ctrl Pts',(-0.726752010060884,0.339129129958207,
-2.18698110648034));
#55441=CARTESIAN_POINT('Ctrl Pts',(-0.773457048196351,0.211993503459735,
-2.18169798304868));
#55442=CARTESIAN_POINT('Ctrl Pts',(-0.786966463557351,0.0814232996746597,
-2.17641485961702));
#55443=CARTESIAN_POINT('Ctrl Pts',(-0.789763670408956,0.0543879425638447,
-2.17532095668592));
#55444=CARTESIAN_POINT('Ctrl Pts',(-0.791137706940641,0.0272053374713011,
-2.17422705375481));
#55445=CARTESIAN_POINT('Ctrl Pts',(-0.791109792329072,1.99241595253492E-5,
-2.17313315082371));
#55446=CARTESIAN_POINT('Origin',(0.,0.,-1.94));
#55447=CARTESIAN_POINT('',(-0.791108239651095,-2.00188069073848E-5,-1.9446668491763));
#55448=CARTESIAN_POINT('',(-0.791123285936247,-1.86130038508075E-5,-1.97313315082371));
#55449=CARTESIAN_POINT('',(-0.7911,-9.68818082805471E-17,-1.94));
#55450=CARTESIAN_POINT('Ctrl Pts',(-0.791108239651095,-2.00188069073848E-5,
-1.9446668491763));
#55451=CARTESIAN_POINT('Ctrl Pts',(-0.791001791698214,0.10359762893025,
-1.94883625448509));
#55452=CARTESIAN_POINT('Ctrl Pts',(-0.770534133686574,0.207256088513461,
-1.95300565979388));
#55453=CARTESIAN_POINT('Ctrl Pts',(-0.73086526413353,0.302955338876006,
-1.95717506510267));
#55454=CARTESIAN_POINT('Ctrl Pts',(-0.680600173857629,0.42421746489593,
-1.96245818853433));
#55455=CARTESIAN_POINT('Ctrl Pts',(-0.599505907586774,0.53270040449236,
-1.96774131196599));
#55456=CARTESIAN_POINT('Ctrl Pts',(-0.497429206777909,0.615231790396717,
-1.97302443539765));
#55457=CARTESIAN_POINT('Ctrl Pts',(-0.395352505969043,0.697763176301074,
-1.97830755882931));
#55458=CARTESIAN_POINT('Ctrl Pts',(-0.272293370622168,0.754343008513358,
-1.98359068226097));
#55459=CARTESIAN_POINT('Ctrl Pts',(-0.143194059239612,0.778101171486672,
-1.98887380569263));
#55460=CARTESIAN_POINT('Ctrl Pts',(-0.0140947478570534,0.801859334459987,
-1.99415692912429));
#55461=CARTESIAN_POINT('Ctrl Pts',(0.121044739561186,0.792795828194329,
-1.99944005255595));
#55462=CARTESIAN_POINT('Ctrl Pts',(0.245815307102121,0.752011174428106,
-2.00472317598761));
#55463=CARTESIAN_POINT('Ctrl Pts',(0.370585874643055,0.711226520661884,
-2.01000629941927));
#55464=CARTESIAN_POINT('Ctrl Pts',(0.484987522306685,0.638720719395097,
-2.01528942285093));
#55465=CARTESIAN_POINT('Ctrl Pts',(0.575129213172718,0.543297671470971,
-2.02057254628259));
#55466=CARTESIAN_POINT('Ctrl Pts',(0.665270904038749,0.447874623546849,
-2.02585566971425));
#55467=CARTESIAN_POINT('Ctrl Pts',(0.731152638107186,0.329534328965388,
-2.03113879314591));
#55468=CARTESIAN_POINT('Ctrl Pts',(0.764774831289796,0.202646068543442,
-2.03642191657757));
#55469=CARTESIAN_POINT('Ctrl Pts',(0.798397024472407,0.0757578081214934,
-2.04170504000923));
#55470=CARTESIAN_POINT('Ctrl Pts',(0.799759676769191,-0.0596784181409368,
-2.04698816344089));
#55471=CARTESIAN_POINT('Ctrl Pts',(0.768697330306502,-0.187217483291771,
-2.05227128687255));
#55472=CARTESIAN_POINT('Ctrl Pts',(0.737634983843813,-0.314756548442608,
-2.05755441030421));
#55473=CARTESIAN_POINT('Ctrl Pts',(0.674147638621649,-0.434398452481844,
-2.06283753373587));
#55474=CARTESIAN_POINT('Ctrl Pts',(0.585944143895796,-0.531615868747983,
-2.06812065716753));
#55475=CARTESIAN_POINT('Ctrl Pts',(0.497740649169944,-0.628833285014119,
-2.07340378059919));
#55476=CARTESIAN_POINT('Ctrl Pts',(0.384821004940404,-0.70362621350716,
-2.07868690403085));
#55477=CARTESIAN_POINT('Ctrl Pts',(0.260896298233043,-0.746913042621927,
-2.08397002746251));
#55478=CARTESIAN_POINT('Ctrl Pts',(0.136971591525681,-0.790199871736694,
-2.08925315089417));
#55479=CARTESIAN_POINT('Ctrl Pts',(0.00204182234049846,-0.801980601473188,
-2.09453627432583));
#55480=CARTESIAN_POINT('Ctrl Pts',(-0.127509378110229,-0.780824775583096,
-2.09981939775749));
#55481=CARTESIAN_POINT('Ctrl Pts',(-0.25706057856096,-0.759668949693004,
-2.10510252118915));
#55482=CARTESIAN_POINT('Ctrl Pts',(-0.381233210277237,-0.705576568176324,
-2.11038564462081));
#55483=CARTESIAN_POINT('Ctrl Pts',(-0.484949810242685,-0.625115711861438,
-2.11566876805247));
#55484=CARTESIAN_POINT('Ctrl Pts',(-0.588666410208131,-0.544654855546555,
-2.12095189148413));
#55485=CARTESIAN_POINT('Ctrl Pts',(-0.671926978422749,-0.437825524433467,
-2.12623501491579));
#55486=CARTESIAN_POINT('Ctrl Pts',(-0.724621733684138,-0.317599299027947,
-2.13151813834745));
#55487=CARTESIAN_POINT('Ctrl Pts',(-0.768337546125482,-0.217859066925389,
-2.13590104195707));
#55488=CARTESIAN_POINT('Ctrl Pts',(-0.791016626503881,-0.108898505033576,
-2.14028394556668));
#55489=CARTESIAN_POINT('Ctrl Pts',(-0.791124794068662,1.84093985718808E-5,
-2.1446668491763));
#55490=CARTESIAN_POINT('Ctrl Pts',(-0.791109792329072,1.99241595253492E-5,
-2.17313315082371));
#55491=CARTESIAN_POINT('Ctrl Pts',(-0.791002890281618,-0.104089579091132,
-2.16894393032315));
#55492=CARTESIAN_POINT('Ctrl Pts',(-0.770335105915875,-0.208240267418343,
-2.1647547098226));
#55493=CARTESIAN_POINT('Ctrl Pts',(-0.730298207536194,-0.304319727528954,
-2.16056548932204));
#55494=CARTESIAN_POINT('Ctrl Pts',(-0.679806743567504,-0.425487769875812,
-2.15528236589038));
#55495=CARTESIAN_POINT('Ctrl Pts',(-0.598510023043591,-0.533819073497853,
-2.14999924245872));
#55496=CARTESIAN_POINT('Ctrl Pts',(-0.496279370104967,-0.616159683281932,
-2.14471611902706));
#55497=CARTESIAN_POINT('Ctrl Pts',(-0.394048717166343,-0.698500293066012,
-2.1394329955954));
#55498=CARTESIAN_POINT('Ctrl Pts',(-0.270884131813007,-0.754850209012131,
-2.13414987216374));
#55499=CARTESIAN_POINT('Ctrl Pts',(-0.141740676645508,-0.778367232787935,
-2.12886674873208));
#55500=CARTESIAN_POINT('Ctrl Pts',(-0.012597221478007,-0.801884256563738,
-2.12358362530042));
#55501=CARTESIAN_POINT('Ctrl Pts',(0.122525103503658,-0.792568388169225,
-2.11830050186876));
#55502=CARTESIAN_POINT('Ctrl Pts',(0.247219286307887,-0.751550792010289,
-2.1130173784371));
#55503=CARTESIAN_POINT('Ctrl Pts',(0.371913469112115,-0.710533195851353,
-2.10773425500544));
#55504=CARTESIAN_POINT('Ctrl Pts',(0.486179509738909,-0.637813871927994,
-2.10245113157378));
#55505=CARTESIAN_POINT('Ctrl Pts',(0.576142837135329,-0.542222647730181,
-2.09716800814212));
#55506=CARTESIAN_POINT('Ctrl Pts',(0.666106164531748,-0.446631423532368,
-2.09188488471046));
#55507=CARTESIAN_POINT('Ctrl Pts',(0.731766778697792,-0.328168299060104,
-2.0866017612788));
#55508=CARTESIAN_POINT('Ctrl Pts',(0.765151944675387,-0.201217469553084,
-2.08131863784714));
#55509=CARTESIAN_POINT('Ctrl Pts',(0.798537110652983,-0.0742666400460645,
-2.07603551441548));
#55510=CARTESIAN_POINT('Ctrl Pts',(0.799646828442127,0.0611718944957136,
-2.07075239098382));
#55511=CARTESIAN_POINT('Ctrl Pts',(0.768346352336834,0.188652726841028,
-2.06546926755216));
#55512=CARTESIAN_POINT('Ctrl Pts',(0.737045876231541,0.316133559186346,
-2.0601861441205));
#55513=CARTESIAN_POINT('Ctrl Pts',(0.673335206231814,0.4356566893352,-2.05490302068884));
#55514=CARTESIAN_POINT('Ctrl Pts',(0.584950308447026,0.532709212555596,
-2.04961989725718));
#55515=CARTESIAN_POINT('Ctrl Pts',(0.496565410662241,0.629761735775988,
-2.04433677382552));
#55516=CARTESIAN_POINT('Ctrl Pts',(0.383506285092399,0.704343652067918,
-2.03905365039386));
#55517=CARTESIAN_POINT('Ctrl Pts',(0.259500955061815,0.747398971644917,
-2.0337705269622));
#55518=CARTESIAN_POINT('Ctrl Pts',(0.135495625031231,0.790454291221916,
-2.02848740353054));
#55519=CARTESIAN_POINT('Ctrl Pts',(0.000544090539904729,0.801983014083983,
-2.02320428009888));
#55520=CARTESIAN_POINT('Ctrl Pts',(-0.128967374382433,0.780585283514092,
-2.01792115666722));
#55521=CARTESIAN_POINT('Ctrl Pts',(-0.25847883930477,0.759187552944201,
-2.01263803323556));
#55522=CARTESIAN_POINT('Ctrl Pts',(-0.38255023465812,0.704863368942352,
-2.0073549098039));
#55523=CARTESIAN_POINT('Ctrl Pts',(-0.486116389889406,0.624208958582592,
-2.00207178637224));
#55524=CARTESIAN_POINT('Ctrl Pts',(-0.589682545120693,0.543554548222831,
-1.99678866294058));
#55525=CARTESIAN_POINT('Ctrl Pts',(-0.672743460229917,0.43656991150516,
-1.99150553950892));
#55526=CARTESIAN_POINT('Ctrl Pts',(-0.72521359657337,0.316245486669755,
-1.98622241607726));
#55527=CARTESIAN_POINT('Ctrl Pts',(-0.768546266560072,0.216875083692276,
-1.98185932765941));
#55528=CARTESIAN_POINT('Ctrl Pts',(-0.791014961891894,0.108406481439749,
-1.97749623924156));
#55529=CARTESIAN_POINT('Ctrl Pts',(-0.791123285936247,-1.86130038508075E-5,
-1.97313315082371));
#55530=CARTESIAN_POINT('Origin',(0.,0.,-1.94));
#55531=CARTESIAN_POINT('',(-0.791041867722209,1.06520765539853E-5,-1.74466684917629));
#55532=CARTESIAN_POINT('',(-0.791036127465933,6.61336014326832E-6,-1.77313315082371));
#55533=CARTESIAN_POINT('',(-0.7911,-9.68818082805471E-17,-1.94));
#55534=CARTESIAN_POINT('Ctrl Pts',(-0.791041867722209,1.06520765539853E-5,
-1.74466684917629));
#55535=CARTESIAN_POINT('Ctrl Pts',(-0.791067426481375,0.0535910187405824,
-1.74682231654017));
#55536=CARTESIAN_POINT('Ctrl Pts',(-0.785703237583341,0.107166337835382,
-1.74897778390405));
#55537=CARTESIAN_POINT('Ctrl Pts',(-0.774898150389007,0.159620888965527,
-1.75113325126792));
#55538=CARTESIAN_POINT('Ctrl Pts',(-0.74841451612285,0.288188768404265,
-1.75641637469958));
#55539=CARTESIAN_POINT('Ctrl Pts',(-0.689244321653519,0.410023559379395,
-1.76169949813124));
#55540=CARTESIAN_POINT('Ctrl Pts',(-0.604572213118025,0.510331667443853,
-1.7669826215629));
#55541=CARTESIAN_POINT('Ctrl Pts',(-0.519900104582533,0.610639775508309,
-1.77226574499456));
#55542=CARTESIAN_POINT('Ctrl Pts',(-0.40972608198088,0.689421200662094,
-1.77754886842622));
#55543=CARTESIAN_POINT('Ctrl Pts',(-0.287427849628273,0.737110034478243,
-1.78283199185788));
#55544=CARTESIAN_POINT('Ctrl Pts',(-0.165129617275666,0.784798868294392,
-1.78811511528954));
#55545=CARTESIAN_POINT('Ctrl Pts',(-0.0307071751721049,0.801395110772904,
-1.7933982387212));
#55546=CARTESIAN_POINT('Ctrl Pts',(0.0995174468488339,0.784883589739994,
-1.79868136215286));
#55547=CARTESIAN_POINT('Ctrl Pts',(0.229742068869776,0.768372068707083,
-1.80396448558452));
#55548=CARTESIAN_POINT('Ctrl Pts',(0.355768870808095,0.718752784162747,
-1.80924760901618));
#55549=CARTESIAN_POINT('Ctrl Pts',(0.462295249996574,0.642050678296546,
-1.81453073244784));
#55550=CARTESIAN_POINT('Ctrl Pts',(0.568821629185048,0.565348572430349,
-1.8198138558795));
#55551=CARTESIAN_POINT('Ctrl Pts',(0.655847585623682,0.461563645242291,
-1.82509697931116));
#55552=CARTESIAN_POINT('Ctrl Pts',(0.712806131873042,0.343297815365377,
-1.83038010274282));
#55553=CARTESIAN_POINT('Ctrl Pts',(0.769764678122405,0.225031985488458,
-1.83566322617448));
#55554=CARTESIAN_POINT('Ctrl Pts',(0.796655814182489,0.0922852529226771,
-1.84094634960614));
#55555=CARTESIAN_POINT('Ctrl Pts',(0.790214326907609,-0.0388238228463354,
-1.8462294730378));
#55556=CARTESIAN_POINT('Ctrl Pts',(0.78377283963273,-0.16993289861535,-1.85151259646946));
#55557=CARTESIAN_POINT('Ctrl Pts',(0.743998729022887,-0.2994043175876,-1.85679571990112));
#55558=CARTESIAN_POINT('Ctrl Pts',(0.675721502783927,-0.411517219987063,
-1.86207884333278));
#55559=CARTESIAN_POINT('Ctrl Pts',(0.60744427654497,-0.523630122386523,
-1.86736196676444));
#55560=CARTESIAN_POINT('Ctrl Pts',(0.510663934676898,-0.618384508213195,
-1.87264509019611));
#55561=CARTESIAN_POINT('Ctrl Pts',(0.397131875253981,-0.684274977861756,
-1.87792821362777));
#55562=CARTESIAN_POINT('Ctrl Pts',(0.283599815831065,-0.750165447510315,
-1.88321133705943));
#55563=CARTESIAN_POINT('Ctrl Pts',(0.153316038853301,-0.787192000980764,
-1.88849446049108));
#55564=CARTESIAN_POINT('Ctrl Pts',(0.0221000433670234,-0.790858748294299,
-1.89377758392274));
#55565=CARTESIAN_POINT('Ctrl Pts',(-0.10911595211926,-0.794525495607834,
-1.8990607073544));
#55566=CARTESIAN_POINT('Ctrl Pts',(-0.24126416611406,-0.764832436764455,
-1.90434383078606));
#55567=CARTESIAN_POINT('Ctrl Pts',(-0.358298713291062,-0.705385003898168,
-1.90962695421773));
#55568=CARTESIAN_POINT('Ctrl Pts',(-0.475333260468061,-0.645937571031883,
-1.91491007764939));
#55569=CARTESIAN_POINT('Ctrl Pts',(-0.57725414082726,-0.556735764142692,
-1.92019320108105));
#55570=CARTESIAN_POINT('Ctrl Pts',(-0.65168577463767,-0.448610769827642,
-1.92547632451271));
#55571=CARTESIAN_POINT('Ctrl Pts',(-0.726117408448082,-0.340485775512588,
-1.93075944794437));
#55572=CARTESIAN_POINT('Ctrl Pts',(-0.773059795709701,-0.213437593771675,
-1.93604257137603));
#55573=CARTESIAN_POINT('Ctrl Pts',(-0.786813032200038,-0.0828928466795056,
-1.94132569480769));
#55574=CARTESIAN_POINT('Ctrl Pts',(-0.789712307396905,-0.055373131767919,
-1.94243941293056));
#55575=CARTESIAN_POINT('Ctrl Pts',(-0.791136673685564,-0.0276980312780681,
-1.94355313105343));
#55576=CARTESIAN_POINT('Ctrl Pts',(-0.791108239651095,-2.00188069073848E-5,
-1.9446668491763));
#55577=CARTESIAN_POINT('Ctrl Pts',(-0.791123285936247,-1.86130038508075E-5,
-1.97313315082371));
#55578=CARTESIAN_POINT('Ctrl Pts',(-0.791146127993088,-0.0228819780586756,
-1.9722131158099));
#55579=CARTESIAN_POINT('Ctrl Pts',(-0.790174710677041,-0.0457434085281455,
-1.97129308079609));
#55580=CARTESIAN_POINT('Ctrl Pts',(-0.788195003339531,-0.0685171891168216,
-1.97037304578228));
#55581=CARTESIAN_POINT('Ctrl Pts',(-0.776826916184554,-0.199291227114849,
-1.96508992235062));
#55582=CARTESIAN_POINT('Ctrl Pts',(-0.732211384296917,-0.32717509015776,
-1.95980679891896));
#55583=CARTESIAN_POINT('Ctrl Pts',(-0.659765777210421,-0.436640684906712,
-1.9545236754873));
#55584=CARTESIAN_POINT('Ctrl Pts',(-0.587320170123928,-0.54610627965566,
-1.94924055205564));
#55585=CARTESIAN_POINT('Ctrl Pts',(-0.487044487838577,-0.637153606110648,
-1.94395742862397));
#55586=CARTESIAN_POINT('Ctrl Pts',(-0.371114544543066,-0.698727388415873,
-1.93867430519231));
#55587=CARTESIAN_POINT('Ctrl Pts',(-0.255184601247555,-0.760301170721097,
-1.93339118176065));
#55588=CARTESIAN_POINT('Ctrl Pts',(-0.123600396941884,-0.792401408876558,
-1.92810805832899));
#55589=CARTESIAN_POINT('Ctrl Pts',(0.00766066702120217,-0.791130382853967,
-1.92282493489733));
#55590=CARTESIAN_POINT('Ctrl Pts',(0.138921730984293,-0.789859356831376,
-1.91754181146567));
#55591=CARTESIAN_POINT('Ctrl Pts',(0.269859654604797,-0.755217066630731,
-1.91225868803401));
#55592=CARTESIAN_POINT('Ctrl Pts',(0.384575510127528,-0.691409896880299,
-1.90697556460235));
#55593=CARTESIAN_POINT('Ctrl Pts',(0.499291365650253,-0.62760272712987,
-1.90169244117069));
#55594=CARTESIAN_POINT('Ctrl Pts',(0.597785153075204,-0.534630677829657,
-1.89640931773903));
#55595=CARTESIAN_POINT('Ctrl Pts',(0.66809742194445,-0.423782731225629,
-1.89112619430737));
#55596=CARTESIAN_POINT('Ctrl Pts',(0.738409690813698,-0.312934784621595,
-1.88584307087571));
#55597=CARTESIAN_POINT('Ctrl Pts',(0.780540441127239,-0.18421094071374,
-1.88055994744405));
#55598=CARTESIAN_POINT('Ctrl Pts',(0.789374013975979,-0.0532412861727047,
-1.87527682401239));
#55599=CARTESIAN_POINT('Ctrl Pts',(0.79820758682472,0.0777283683683321,
-1.86999370058073));
#55600=CARTESIAN_POINT('Ctrl Pts',(0.773743982208662,0.210943833542553,
-1.86471057714907));
#55601=CARTESIAN_POINT('Ctrl Pts',(0.718953654154168,0.330229634757758,
-1.85942745371741));
#55602=CARTESIAN_POINT('Ctrl Pts',(0.664163326099674,0.449515435972964,
-1.85414433028575));
#55603=CARTESIAN_POINT('Ctrl Pts',(0.579046274606745,0.554871573229153,
-1.84886120685409));
#55604=CARTESIAN_POINT('Ctrl Pts',(0.473937701387782,0.63350534622617,-1.84357808342243));
#55605=CARTESIAN_POINT('Ctrl Pts',(0.368829128168824,0.712139119223182,
-1.83829495999077));
#55606=CARTESIAN_POINT('Ctrl Pts',(0.243729033223835,0.764050527961024,
-1.83301183655911));
#55607=CARTESIAN_POINT('Ctrl Pts',(0.113827495306941,0.782936312739435,
-1.82772871312745));
#55608=CARTESIAN_POINT('Ctrl Pts',(-0.0160740426099603,0.801822097517847,
-1.82244558969579));
#55609=CARTESIAN_POINT('Ctrl Pts',(-0.150777023498765,0.787682258336824,
-1.81716246626413));
#55610=CARTESIAN_POINT('Ctrl Pts',(-0.273925353553017,0.742233702532247,
-1.81187934283247));
#55611=CARTESIAN_POINT('Ctrl Pts',(-0.397073683607268,0.696785146727671,
-1.80659621940081));
#55612=CARTESIAN_POINT('Ctrl Pts',(-0.508667362826965,0.620027874299541,
-1.80131309596915));
#55613=CARTESIAN_POINT('Ctrl Pts',(-0.595156307364805,0.521282014170606,
-1.79602997253749));
#55614=CARTESIAN_POINT('Ctrl Pts',(-0.681645251902642,0.422536154041674,
-1.79074684910583));
#55615=CARTESIAN_POINT('Ctrl Pts',(-0.743029461758622,0.30180170621194,
-1.78546372567417));
#55616=CARTESIAN_POINT('Ctrl Pts',(-0.771855457521859,0.17373865772359,
-1.78018060224251));
#55617=CARTESIAN_POINT('Ctrl Pts',(-0.784672989130951,0.116795189562486,
-1.77783145176958));
#55618=CARTESIAN_POINT('Ctrl Pts',(-0.79105326546298,0.0584027453264418,
-1.77548230129664));
#55619=CARTESIAN_POINT('Ctrl Pts',(-0.791036127465933,6.61336014326832E-6,
-1.77313315082371));
#55620=CARTESIAN_POINT('Origin',(0.,0.,-1.94));
#55621=CARTESIAN_POINT('',(-0.791166035532024,3.68633254679493E-6,-1.5446668491763));
#55622=CARTESIAN_POINT('',(-0.791159979474253,8.47231515970201E-6,-1.5731331508237));
#55623=CARTESIAN_POINT('',(-0.7911,-9.68818082805471E-17,-1.94));
#55624=CARTESIAN_POINT('Ctrl Pts',(-0.791166035532024,3.68633254679493E-6,
-1.5446668491763));
#55625=CARTESIAN_POINT('Ctrl Pts',(-0.791166952605422,0.00352021813421264,
-1.54480837859526));
#55626=CARTESIAN_POINT('Ctrl Pts',(-0.79114399565106,0.007036737919245,
-1.54494990801422));
#55627=CARTESIAN_POINT('Ctrl Pts',(-0.791097090858486,0.0105529382491046,
-1.54509143743318));
#55628=CARTESIAN_POINT('Ctrl Pts',(-0.789346191218509,0.141808478542717,
-1.55037456086484));
#55629=CARTESIAN_POINT('Ctrl Pts',(-0.754225431715114,0.272618877431325,
-1.5556576842965));
#55630=CARTESIAN_POINT('Ctrl Pts',(-0.689999294345667,0.387100691646154,
-1.56094080772816));
#55631=CARTESIAN_POINT('Ctrl Pts',(-0.625773156976222,0.501582505860979,
-1.56622393115982));
#55632=CARTESIAN_POINT('Ctrl Pts',(-0.532441641740725,0.599735735402025,
-1.57150705459148));
#55633=CARTESIAN_POINT('Ctrl Pts',(-0.421337378460864,0.669642281507206,
-1.57679017802314));
#55634=CARTESIAN_POINT('Ctrl Pts',(-0.310233115181003,0.739548827612388,
-1.5820733014548));
#55635=CARTESIAN_POINT('Ctrl Pts',(-0.181356103856777,0.781208690281705,
-1.58735642488646));
#55636=CARTESIAN_POINT('Ctrl Pts',(-0.0503550292671448,0.789563387384417,
-1.59263954831812));
#55637=CARTESIAN_POINT('Ctrl Pts',(0.0806460453224916,0.797918084487129,
-1.59792267174978));
#55638=CARTESIAN_POINT('Ctrl Pts',(0.213771183177535,0.772967616023235,
-1.60320579518144));
#55639=CARTESIAN_POINT('Ctrl Pts',(0.33285587755591,0.717741552682394,-1.6084889186131));
#55640=CARTESIAN_POINT('Ctrl Pts',(0.451940571934281,0.662515489341555,
-1.61377204204476));
#55641=CARTESIAN_POINT('Ctrl Pts',(0.556984822835985,0.577013831123771,
-1.61905516547642));
#55642=CARTESIAN_POINT('Ctrl Pts',(0.635233800262155,0.471618479997285,
-1.62433828890808));
#55643=CARTESIAN_POINT('Ctrl Pts',(0.713482777688325,0.366223128870799,
-1.62962141233974));
#55644=CARTESIAN_POINT('Ctrl Pts',(0.764936481638961,0.240934084835611,
-1.6349045357714));
#55645=CARTESIAN_POINT('Ctrl Pts',(0.783347228484842,0.110964369486637,
-1.64018765920306));
#55646=CARTESIAN_POINT('Ctrl Pts',(0.801757975330723,-0.0190053458623417,
-1.64547078263472));
#55647=CARTESIAN_POINT('Ctrl Pts',(0.787125765071846,-0.153655732525106,
-1.65075390606638));
#55648=CARTESIAN_POINT('Ctrl Pts',(0.741227290413978,-0.276637082864898,
-1.65603702949804));
#55649=CARTESIAN_POINT('Ctrl Pts',(0.695328815756111,-0.39961843320469,
-1.6613201529297));
#55650=CARTESIAN_POINT('Ctrl Pts',(0.618164076699251,-0.510930747221509,
-1.66660327636136));
#55651=CARTESIAN_POINT('Ctrl Pts',(0.519102678149224,-0.597058105387367,
-1.67188639979302));
#55652=CARTESIAN_POINT('Ctrl Pts',(0.4200412795992,-0.683185463553224,-1.67716952322468));
#55653=CARTESIAN_POINT('Ctrl Pts',(0.299083221556008,-0.744127865868122,
-1.68245264665634));
#55654=CARTESIAN_POINT('Ctrl Pts',(0.170915642574026,-0.772485478694556,
-1.687735770088));
#55655=CARTESIAN_POINT('Ctrl Pts',(0.0427480635920437,-0.80084309152099,
-1.69301889351966));
#55656=CARTESIAN_POINT('Ctrl Pts',(-0.092629036328729,-0.79661591485896,
-1.69830201695132));
#55657=CARTESIAN_POINT('Ctrl Pts',(-0.218777709557586,-0.760317226867303,
-1.70358514038298));
#55658=CARTESIAN_POINT('Ctrl Pts',(-0.344926382786443,-0.724018538875647,
-1.70886826381464));
#55659=CARTESIAN_POINT('Ctrl Pts',(-0.461846629323384,-0.655648339554364,
-1.7141513872463));
#55660=CARTESIAN_POINT('Ctrl Pts',(-0.555341595411988,-0.563508370901193,
-1.71943451067796));
#55661=CARTESIAN_POINT('Ctrl Pts',(-0.648836561500592,-0.471368402248023,
-1.72471763410962));
#55662=CARTESIAN_POINT('Ctrl Pts',(-0.71890624714086,-0.355458664262964,
-1.73000075754128));
#55663=CARTESIAN_POINT('Ctrl Pts',(-0.757042552929503,-0.229853311319263,
-1.73528388097294));
#55664=CARTESIAN_POINT('Ctrl Pts',(-0.779619585199458,-0.155493825049006,
-1.73841153704073));
#55665=CARTESIAN_POINT('Ctrl Pts',(-0.791004781097966,-0.0777362726597893,
-1.74153919310851));
#55666=CARTESIAN_POINT('Ctrl Pts',(-0.791041867722209,1.06520765539853E-5,
-1.74466684917629));
#55667=CARTESIAN_POINT('Ctrl Pts',(-0.791036127465933,6.61336014326832E-6,
-1.77313315082371));
#55668=CARTESIAN_POINT('Ctrl Pts',(-0.791014722953756,-0.0729272723390494,
-1.77019917786498));
#55669=CARTESIAN_POINT('Ctrl Pts',(-0.781014134674409,-0.145866910446324,
-1.76726520490626));
#55670=CARTESIAN_POINT('Ctrl Pts',(-0.761111981169042,-0.215996575470099,
-1.76433123194753));
#55671=CARTESIAN_POINT('Ctrl Pts',(-0.725274727382491,-0.342277111028477,
-1.75904810851587));
#55672=CARTESIAN_POINT('Ctrl Pts',(-0.657332438138893,-0.459446532998264,
-1.75376498508421));
#55673=CARTESIAN_POINT('Ctrl Pts',(-0.56553489713985,-0.553277731895016,
-1.74848186165255));
#55674=CARTESIAN_POINT('Ctrl Pts',(-0.473737356140807,-0.647108930791767,
-1.74319873822089));
#55675=CARTESIAN_POINT('Ctrl Pts',(-0.358084563386321,-0.717601906615482,
-1.73791561478923));
#55676=CARTESIAN_POINT('Ctrl Pts',(-0.232619474086362,-0.756197162629997,
-1.73263249135757));
#55677=CARTESIAN_POINT('Ctrl Pts',(-0.107154384786411,-0.79479241864451,
-1.72734936792591));
#55678=CARTESIAN_POINT('Ctrl Pts',(0.0281230010590105,-0.801489954849828,
-1.72206624449425));
#55679=CARTESIAN_POINT('Ctrl Pts',(0.156786843441164,-0.775476533634403,
-1.71678312106259));
#55680=CARTESIAN_POINT('Ctrl Pts',(0.285450685823325,-0.749463112418977,
-1.71149999763093));
#55681=CARTESIAN_POINT('Ctrl Pts',(0.407500984742214,-0.690738733782805,
-1.70621687419927));
#55682=CARTESIAN_POINT('Ctrl Pts',(0.50811797804371,-0.606433911389069,
-1.70093375076761));
#55683=CARTESIAN_POINT('Ctrl Pts',(0.608734971345201,-0.522129088995338,
-1.69565062733595));
#55684=CARTESIAN_POINT('Ctrl Pts',(0.687918659029299,-0.412243822844049,
-1.69036750390429));
#55685=CARTESIAN_POINT('Ctrl Pts',(0.736054288585285,-0.290120755460693,
-1.68508438047263));
#55686=CARTESIAN_POINT('Ctrl Pts',(0.784189918141273,-0.167997688077334,
-1.67980125704097));
#55687=CARTESIAN_POINT('Ctrl Pts',(0.801277489569146,-0.0336368194619003,
-1.67451813360931));
#55688=CARTESIAN_POINT('Ctrl Pts',(0.785242171864016,0.096647297014235,
-1.66923501017765));
#55689=CARTESIAN_POINT('Ctrl Pts',(0.769206854158885,0.226931413490374,
-1.66395188674599));
#55690=CARTESIAN_POINT('Ctrl Pts',(0.720048647320751,0.353138777827222,
-1.65866876331433));
#55691=CARTESIAN_POINT('Ctrl Pts',(0.643736507916843,0.459944862857389,
-1.65338563988267));
#55692=CARTESIAN_POINT('Ctrl Pts',(0.567424368512935,0.566750947887556,
-1.64810251645101));
#55693=CARTESIAN_POINT('Ctrl Pts',(0.463958296543255,0.65415575361104,-1.64281939301935));
#55694=CARTESIAN_POINT('Ctrl Pts',(0.345901494156378,0.711546291420495,
-1.63753626958769));
#55695=CARTESIAN_POINT('Ctrl Pts',(0.227844691769501,0.768936829229949,
-1.63225314615603));
#55696=CARTESIAN_POINT('Ctrl Pts',(0.095197158965428,0.796313099125374,
-1.62697002272437));
#55697=CARTESIAN_POINT('Ctrl Pts',(-0.0359345899424767,0.790350981361787,
-1.62168689929271));
#55698=CARTESIAN_POINT('Ctrl Pts',(-0.167066338850374,0.7843888635982,-1.61640377586105));
#55699=CARTESIAN_POINT('Ctrl Pts',(-0.296682303862101,0.745088358175606,
-1.61112065242939));
#55700=CARTESIAN_POINT('Ctrl Pts',(-0.4090440739302,0.67722146604819,-1.60583752899773));
#55701=CARTESIAN_POINT('Ctrl Pts',(-0.521405843998305,0.609354573920769,
-1.60055440556607));
#55702=CARTESIAN_POINT('Ctrl Pts',(-0.616513419122778,0.512921295088524,
-1.59527128213441));
#55703=CARTESIAN_POINT('Ctrl Pts',(-0.682818514253234,0.399630886052217,
-1.58998815870275));
#55704=CARTESIAN_POINT('Ctrl Pts',(-0.749123609383688,0.286340477015913,
-1.58470503527108));
#55705=CARTESIAN_POINT('Ctrl Pts',(-0.786626224520126,0.15619293777555,
-1.57942191183943));
#55706=CARTESIAN_POINT('Ctrl Pts',(-0.790772664658091,0.0249912249282936,
-1.57413878840777));
#55707=CARTESIAN_POINT('Ctrl Pts',(-0.79103575498693,0.0166665173167768,
-1.57380357587975));
#55708=CARTESIAN_POINT('Ctrl Pts',(-0.791164557932427,0.00833756574697465,
-1.57346836335172));
#55709=CARTESIAN_POINT('Ctrl Pts',(-0.791159979474253,8.47231515970201E-6,
-1.5731331508237));
#55710=CARTESIAN_POINT('Origin',(0.,0.,-1.94));
#55711=CARTESIAN_POINT('',(-0.791054873532962,-1.56092113809958E-5,-1.34466684917629));
#55712=CARTESIAN_POINT('',(-0.791066487406845,-1.81135318691069E-5,-1.3731331508237));
#55713=CARTESIAN_POINT('',(-0.7911,-9.68818082805471E-17,-1.94));
#55714=CARTESIAN_POINT('Ctrl Pts',(-0.791054873532962,-1.56092113809958E-5,
-1.34466684917629));
#55715=CARTESIAN_POINT('Ctrl Pts',(-0.790994308958492,0.0847635680099431,
-1.348077564082));
#55716=CARTESIAN_POINT('Ctrl Pts',(-0.777416502544745,0.169561683102478,
-1.35148827898771));
#55717=CARTESIAN_POINT('Ctrl Pts',(-0.750641953334654,0.249965256714577,
-1.35489899389341));
#55718=CARTESIAN_POINT('Ctrl Pts',(-0.709168757182336,0.37450864878428,
-1.36018211732507));
#55719=CARTESIAN_POINT('Ctrl Pts',(-0.636032169671575,0.488508068838821,
-1.36546524075673));
#55720=CARTESIAN_POINT('Ctrl Pts',(-0.540112683855437,0.578121319801412,
-1.37074836418839));
#55721=CARTESIAN_POINT('Ctrl Pts',(-0.444193198039299,0.667734570764002,
-1.37603148762005));
#55722=CARTESIAN_POINT('Ctrl Pts',(-0.325490813917783,0.732961652634642,
-1.38131461105171));
#55723=CARTESIAN_POINT('Ctrl Pts',(-0.198418778450467,0.765882471420174,
-1.38659773448337));
#55724=CARTESIAN_POINT('Ctrl Pts',(-0.0713467429831482,0.798803290205708,
-1.39188085791503));
#55725=CARTESIAN_POINT('Ctrl Pts',(0.0640949438299711,0.799417845906132,
-1.39716398134669));
#55726=CARTESIAN_POINT('Ctrl Pts',(0.191460491998178,0.767651517079374,
-1.40244710477835));
#55727=CARTESIAN_POINT('Ctrl Pts',(0.318826040166385,0.735885188252617,
-1.40773022821001));
#55728=CARTESIAN_POINT('Ctrl Pts',(0.43811544968968,0.671737974898678,-1.41301335164167));
#55729=CARTESIAN_POINT('Ctrl Pts',(0.53484419498885,0.58299884970485,-1.41829647507333));
#55730=CARTESIAN_POINT('Ctrl Pts',(0.631572940288017,0.494259724511026,
-1.42357959850499));
#55731=CARTESIAN_POINT('Ctrl Pts',(0.705741021363061,0.380928687477314,
-1.42886272193665));
#55732=CARTESIAN_POINT('Ctrl Pts',(0.748342697706208,0.256766778342223,
-1.43414584536831));
#55733=CARTESIAN_POINT('Ctrl Pts',(0.790944374049354,0.132604869207133,
-1.43942896879997));
#55734=CARTESIAN_POINT('Ctrl Pts',(0.801979645660603,-0.00238791202933467,
-1.44471209223163));
#55735=CARTESIAN_POINT('Ctrl Pts',(0.780108572351085,-0.131820283017454,
-1.44999521566329));
#55736=CARTESIAN_POINT('Ctrl Pts',(0.758237499041567,-0.261252654005574,
-1.45527833909495));
#55737=CARTESIAN_POINT('Ctrl Pts',(0.703460080811282,-0.385124614745345,
-1.46056146252661));
#55738=CARTESIAN_POINT('Ctrl Pts',(0.622427577974875,-0.488395210712369,
-1.46584458595827));
#55739=CARTESIAN_POINT('Ctrl Pts',(0.541395075138469,-0.591665806679393,
-1.47112770938993));
#55740=CARTESIAN_POINT('Ctrl Pts',(0.434107487695941,-0.674335037873671,
-1.47641083282159));
#55741=CARTESIAN_POINT('Ctrl Pts',(0.313592039194238,-0.726364925243813,
-1.48169395625325));
#55742=CARTESIAN_POINT('Ctrl Pts',(0.193076590692534,-0.778394812613955,
-1.48697707968491));
#55743=CARTESIAN_POINT('Ctrl Pts',(0.059333281131654,-0.799785356159962,
-1.49226020311657));
#55744=CARTESIAN_POINT('Ctrl Pts',(-0.0713983222365862,-0.787939243376194,
-1.49754332654823));
#55745=CARTESIAN_POINT('Ctrl Pts',(-0.202129925604834,-0.776093130592426,
-1.50282644997989));
#55746=CARTESIAN_POINT('Ctrl Pts',(-0.329849822780441,-0.731010361478878,
-1.50810957341156));
#55747=CARTESIAN_POINT('Ctrl Pts',(-0.439049829717504,-0.658165039101501,
-1.51339269684322));
#55748=CARTESIAN_POINT('Ctrl Pts',(-0.54824983665456,-0.585319716724129,
-1.51867582027488));
#55749=CARTESIAN_POINT('Ctrl Pts',(-0.638929953353074,-0.48471184108293,
-1.52395894370654));
#55750=CARTESIAN_POINT('Ctrl Pts',(-0.70007949181405,-0.368557562413024,
-1.5292420671382));
#55751=CARTESIAN_POINT('Ctrl Pts',(-0.759590897310686,-0.25551493687456,
-1.5343836611509));
#55752=CARTESIAN_POINT('Ctrl Pts',(-0.791132719355588,-0.127747695604292,
-1.5395252551636));
#55753=CARTESIAN_POINT('Ctrl Pts',(-0.791166035532024,3.68633254679493E-6,
-1.5446668491763));
#55754=CARTESIAN_POINT('Ctrl Pts',(-0.791159979474253,8.47231515970201E-6,
-1.5731331508237));
#55755=CARTESIAN_POINT('Ctrl Pts',(-0.791092399055183,-0.122933269904619,
-1.56818523992006));
#55756=CARTESIAN_POINT('Ctrl Pts',(-0.761964622417966,-0.245905920015694,
-1.56323732901642));
#55757=CARTESIAN_POINT('Ctrl Pts',(-0.706690205369702,-0.355717475151843,
-1.55828941811278));
#55758=CARTESIAN_POINT('Ctrl Pts',(-0.647671040803863,-0.472968575930565,
-1.55300629468112));
#55759=CARTESIAN_POINT('Ctrl Pts',(-0.558842446532696,-0.57521489103386,
-1.54772317124947));
#55760=CARTESIAN_POINT('Ctrl Pts',(-0.450990292408587,-0.650041325337929,
-1.5424400478178));
#55761=CARTESIAN_POINT('Ctrl Pts',(-0.343138138284478,-0.724867759641997,
-1.53715692438614));
#55762=CARTESIAN_POINT('Ctrl Pts',(-0.216262424307427,-0.772274313146837,
-1.53187380095448));
#55763=CARTESIAN_POINT('Ctrl Pts',(-0.0857688309299165,-0.786504720986968,
-1.52659067752282));
#55764=CARTESIAN_POINT('Ctrl Pts',(0.0447247624475942,-0.800735128827099,
-1.52130755409116));
#55765=CARTESIAN_POINT('Ctrl Pts',(0.178836235225564,-0.781789391002521,
-1.5160244306595));
#55766=CARTESIAN_POINT('Ctrl Pts',(0.300281316522941,-0.731967963398073,
-1.51074130722784));
#55767=CARTESIAN_POINT('Ctrl Pts',(0.421726397820321,-0.682146535793625,
-1.50545818379618));
#55768=CARTESIAN_POINT('Ctrl Pts',(0.530505087637106,-0.601449418409306,
-1.50017506036452));
#55769=CARTESIAN_POINT('Ctrl Pts',(0.613409107707684,-0.499675129534317,
-1.49489193693286));
#55770=CARTESIAN_POINT('Ctrl Pts',(0.696313127778262,-0.397900840659328,
-1.4896088135012));
#55771=CARTESIAN_POINT('Ctrl Pts',(0.753342478102633,-0.275049380293668,
-1.48432569006954));
#55772=CARTESIAN_POINT('Ctrl Pts',(0.777572461116777,-0.146037790337545,
-1.47904256663788));
#55773=CARTESIAN_POINT('Ctrl Pts',(0.80180244413092,-0.0170262003814258,
-1.47375944320622));
#55774=CARTESIAN_POINT('Ctrl Pts',(0.793233059834839,0.118145519165157,
-1.46847631977456));
#55775=CARTESIAN_POINT('Ctrl Pts',(0.752904831997833,0.243064358654635,
-1.4631931963429));
#55776=CARTESIAN_POINT('Ctrl Pts',(0.712576604160826,0.367983198144114,
-1.45791007291124));
#55777=CARTESIAN_POINT('Ctrl Pts',(0.640489532782895,0.482649157576488,
-1.45262694947958));
#55778=CARTESIAN_POINT('Ctrl Pts',(0.545396675100861,0.573139106398089,
-1.44734382604792));
#55779=CARTESIAN_POINT('Ctrl Pts',(0.450303817418827,0.663629055219689,
-1.44206070261626));
#55780=CARTESIAN_POINT('Ctrl Pts',(0.332205173432689,0.729942993430516,
-1.4367775791846));
#55781=CARTESIAN_POINT('Ctrl Pts',(0.205440681922623,0.76402885724627,-1.43149445575294));
#55782=CARTESIAN_POINT('Ctrl Pts',(0.0786761904125578,0.798114721062024,
-1.42621133232128));
#55783=CARTESIAN_POINT('Ctrl Pts',(-0.0567541486214352,0.799972510482705,
-1.42092820888962));
#55784=CARTESIAN_POINT('Ctrl Pts',(-0.184405923074557,0.769376646402069,
-1.41564508545796));
#55785=CARTESIAN_POINT('Ctrl Pts',(-0.312057697527683,0.738780782321432,
-1.4103619620263));
#55786=CARTESIAN_POINT('Ctrl Pts',(-0.431930907399938,0.675731264739476,
-1.40507883859464));
#55787=CARTESIAN_POINT('Ctrl Pts',(-0.529470140089352,0.587883780391699,
-1.39979571516298));
#55788=CARTESIAN_POINT('Ctrl Pts',(-0.627009372778766,0.500036296043922,
-1.39451259173132));
#55789=CARTESIAN_POINT('Ctrl Pts',(-0.702214628285339,0.387390844930324,
-1.38922946829966));
#55790=CARTESIAN_POINT('Ctrl Pts',(-0.745954228856374,0.263625220616629,
-1.383946344868));
#55791=CARTESIAN_POINT('Ctrl Pts',(-0.775795464160492,0.179186426720742,
-1.38034194685324));
#55792=CARTESIAN_POINT('Ctrl Pts',(-0.790990641636737,0.0895716178943466,
-1.37673754883847));
#55793=CARTESIAN_POINT('Ctrl Pts',(-0.791066487406845,-1.81135318691069E-5,
-1.3731331508237));
#55794=CARTESIAN_POINT('Origin',(0.,0.,-1.94));
#55795=CARTESIAN_POINT('',(-0.791086342131762,2.01490389672293E-5,-1.1446668491763));
#55796=CARTESIAN_POINT('',(-0.79107238223822,1.89686955811942E-5,-1.1731331508237));
#55797=CARTESIAN_POINT('',(-0.7911,-9.68818082805471E-17,-1.94));
#55798=CARTESIAN_POINT('Ctrl Pts',(-0.791086342131762,2.01490389672293E-5,
-1.1446668491763));
#55799=CARTESIAN_POINT('Ctrl Pts',(-0.791120376438806,0.0347354763001229,
-1.14606362613709));
#55800=CARTESIAN_POINT('Ctrl Pts',(-0.788877432756344,0.0694464381092138,
-1.14746040309788));
#55801=CARTESIAN_POINT('Ctrl Pts',(-0.784321936747084,0.103851197430517,
-1.14885718005867));
#55802=CARTESIAN_POINT('Ctrl Pts',(-0.767091377835423,0.233982632321972,
-1.15414030349033));
#55803=CARTESIAN_POINT('Ctrl Pts',(-0.716776746918577,0.35973344194638,
-1.15942342692199));
#55804=CARTESIAN_POINT('Ctrl Pts',(-0.6394874175062,0.465834535561396,-1.16470655035365));
#55805=CARTESIAN_POINT('Ctrl Pts',(-0.562198088093824,0.571935629176409,
-1.16998967378531));
#55806=CARTESIAN_POINT('Ctrl Pts',(-0.457934060185918,0.658387006782034,
-1.17527279721697));
#55807=CARTESIAN_POINT('Ctrl Pts',(-0.339355426453396,0.714691448253778,
-1.18055592064863));
#55808=CARTESIAN_POINT('Ctrl Pts',(-0.220776792720872,0.770995889725524,
-1.18583904408029));
#55809=CARTESIAN_POINT('Ctrl Pts',(-0.0878835531637302,0.797153395063388,
-1.19112216751195));
#55810=CARTESIAN_POINT('Ctrl Pts',(0.0431879433555249,0.78998783105765,
-1.19640529094361));
#55811=CARTESIAN_POINT('Ctrl Pts',(0.174259439874776,0.782822267051912,
-1.20168841437527));
#55812=CARTESIAN_POINT('Ctrl Pts',(0.303509193356143,0.742333633702575,
-1.20697153780693));
#55813=CARTESIAN_POINT('Ctrl Pts',(0.415243259400964,0.673438198495239,
-1.21225466123859));
#55814=CARTESIAN_POINT('Ctrl Pts',(0.52697732544578,0.604542763287905,-1.21753778467025));
#55815=CARTESIAN_POINT('Ctrl Pts',(0.621195704054054,0.507240526222574,
-1.22282090810191));
#55816=CARTESIAN_POINT('Ctrl Pts',(0.686458079438849,0.393346255662332,
-1.22810403153357));
#55817=CARTESIAN_POINT('Ctrl Pts',(0.751720454823647,0.279451985102084,
-1.23338715496523));
#55818=CARTESIAN_POINT('Ctrl Pts',(0.788026826984966,0.148965681046922,
-1.23867027839689));
#55819=CARTESIAN_POINT('Ctrl Pts',(0.790968752806516,0.017731434069321,
-1.24395340182855));
#55820=CARTESIAN_POINT('Ctrl Pts',(0.793910678628066,-0.113502812908284,
-1.24923652526021));
#55821=CARTESIAN_POINT('Ctrl Pts',(0.763488158109848,-0.245485002808319,
-1.25451964869187));
#55822=CARTESIAN_POINT('Ctrl Pts',(0.703395197101927,-0.362189409514402,
-1.25980277212353));
#55823=CARTESIAN_POINT('Ctrl Pts',(0.643302236094011,-0.478893816220475,
-1.26508589555519));
#55824=CARTESIAN_POINT('Ctrl Pts',(0.553538834596398,-0.58032043973259,
-1.27036901898685));
#55825=CARTESIAN_POINT('Ctrl Pts',(0.445004369932397,-0.654153714666148,
-1.27565214241851));
#55826=CARTESIAN_POINT('Ctrl Pts',(0.33646990526839,-0.727986989599709,
-1.28093526585017));
#55827=CARTESIAN_POINT('Ctrl Pts',(0.209164377437992,-0.774226915954711,
-1.28621838928183));
#55828=CARTESIAN_POINT('Ctrl Pts',(0.0785456563527366,-0.787258884699669,
-1.29150151271349));
#55829=CARTESIAN_POINT('Ctrl Pts',(-0.0520730647325192,-0.800290853444627,
-1.29678463614515));
#55830=CARTESIAN_POINT('Ctrl Pts',(-0.186004979072635,-0.780114864579541,
-1.30206775957681));
#55831=CARTESIAN_POINT('Ctrl Pts',(-0.306987618382414,-0.729180755252319,
-1.30735088300847));
#55832=CARTESIAN_POINT('Ctrl Pts',(-0.42797025769219,-0.678246645925099,
-1.31263400644013));
#55833=CARTESIAN_POINT('Ctrl Pts',(-0.536003621971631,-0.596554416135744,
-1.31791712987179));
#55834=CARTESIAN_POINT('Ctrl Pts',(-0.617969932915293,-0.494023414104147,
-1.32320025330345));
#55835=CARTESIAN_POINT('Ctrl Pts',(-0.699936243858955,-0.39149241207255,
-1.32848337673511));
#55836=CARTESIAN_POINT('Ctrl Pts',(-0.755835501466839,-0.268122637798709,
-1.33376650016677));
#55837=CARTESIAN_POINT('Ctrl Pts',(-0.778880227873844,-0.138894068619357,
-1.33904962359843));
#55838=CARTESIAN_POINT('Ctrl Pts',(-0.787047582424787,-0.0930937616876116,
-1.34092203212439));
#55839=CARTESIAN_POINT('Ctrl Pts',(-0.791088122171075,-0.0465575391707168,
-1.34279444065034));
#55840=CARTESIAN_POINT('Ctrl Pts',(-0.791054873532962,-1.56092113809958E-5,
-1.34466684917629));
#55841=CARTESIAN_POINT('Ctrl Pts',(-0.791066487406845,-1.81135318691069E-5,
-1.3731331508237));
#55842=CARTESIAN_POINT('Ctrl Pts',(-0.791101812091168,-0.0417439602951441,
-1.37145442540681));
#55843=CARTESIAN_POINT('Ctrl Pts',(-0.787857494745136,-0.0834643673407622,
-1.36977569998991));
#55844=CARTESIAN_POINT('Ctrl Pts',(-0.781285721563619,-0.124653879902264,
-1.36809697457302));
#55845=CARTESIAN_POINT('Ctrl Pts',(-0.760603668064331,-0.254281558593677,
-1.36281385114136));
#55846=CARTESIAN_POINT('Ctrl Pts',(-0.706965615430256,-0.378651118462714,
-1.3575307277097));
#55847=CARTESIAN_POINT('Ctrl Pts',(-0.626884478332546,-0.48266118480732,
-1.35224760427804));
#55848=CARTESIAN_POINT('Ctrl Pts',(-0.546803341234833,-0.586671251151929,
-1.34696448084638));
#55849=CARTESIAN_POINT('Ctrl Pts',(-0.440279119673483,-0.670321823972104,
-1.34168135741472));
#55850=CARTESIAN_POINT('Ctrl Pts',(-0.320246346715405,-0.723455766380578,
-1.33639823398306));
#55851=CARTESIAN_POINT('Ctrl Pts',(-0.200213573757331,-0.776589708789051,
-1.3311151105514));
#55852=CARTESIAN_POINT('Ctrl Pts',(-0.0666722494025287,-0.799207020785824,
-1.32583198711974));
#55853=CARTESIAN_POINT('Ctrl Pts',(0.0641625848274726,-0.788561431470073,
-1.32054886368808));
#55854=CARTESIAN_POINT('Ctrl Pts',(0.194997419057474,-0.777915842154323,
-1.31526574025642));
#55855=CARTESIAN_POINT('Ctrl Pts',(0.323125763162674,-0.734007351526049,
-1.30998261682476));
#55856=CARTESIAN_POINT('Ctrl Pts',(0.432989838082634,-0.662167477766046,
-1.3046994933931));
#55857=CARTESIAN_POINT('Ctrl Pts',(0.542853913002597,-0.590327604006042,
-1.29941636996144));
#55858=CARTESIAN_POINT('Ctrl Pts',(0.634453718737318,-0.490556347114309,
-1.29413324652978));
#55859=CARTESIAN_POINT('Ctrl Pts',(0.696666895518923,-0.374968272233665,
-1.28885012309812));
#55860=CARTESIAN_POINT('Ctrl Pts',(0.758880072300526,-0.259380197353024,
-1.28356699966646));
#55861=CARTESIAN_POINT('Ctrl Pts',(0.791706620129014,-0.127975304483475,
-1.2782838762348));
#55862=CARTESIAN_POINT('Ctrl Pts',(0.791160627986813,0.00329077762630802,
-1.27300075280314));
#55863=CARTESIAN_POINT('Ctrl Pts',(0.790614635844611,0.134556859736091,
-1.26771762937148));
#55864=CARTESIAN_POINT('Ctrl Pts',(0.75669610373172,0.265684131086106,-1.26243450593982));
#55865=CARTESIAN_POINT('Ctrl Pts',(0.693523535109274,0.38075067267624,-1.25715138250816));
#55866=CARTESIAN_POINT('Ctrl Pts',(0.630350966486827,0.495817214266377,
-1.2518682590765));
#55867=CARTESIAN_POINT('Ctrl Pts',(0.537924361354823,0.59482302609663,-1.24658513564484));
#55868=CARTESIAN_POINT('Ctrl Pts',(0.427466472274317,0.665746485965359,
-1.24130201221318));
#55869=CARTESIAN_POINT('Ctrl Pts',(0.317008583193811,0.736669945834088,
-1.23601888878152));
#55870=CARTESIAN_POINT('Ctrl Pts',(0.188519410164803,0.779511053741293,
-1.23073576534986));
#55871=CARTESIAN_POINT('Ctrl Pts',(0.0576005453221517,0.789067896744294,
-1.2254526419182));
#55872=CARTESIAN_POINT('Ctrl Pts',(-0.0733183195204963,0.798624739747296,
-1.22016951848654));
#55873=CARTESIAN_POINT('Ctrl Pts',(-0.206666876176788,0.774897317846096,
-1.21488639505488));
#55874=CARTESIAN_POINT('Ctrl Pts',(-0.326253489634383,0.720766695259472,
-1.20960327162322));
#55875=CARTESIAN_POINT('Ctrl Pts',(-0.445840103091977,0.666636072672849,
-1.20432014819156));
#55876=CARTESIAN_POINT('Ctrl Pts',(-0.551664773350874,0.582102249400802,
-1.1990370247599));
#55877=CARTESIAN_POINT('Ctrl Pts',(-0.630877909241144,0.47742960960271,
-1.19375390132824));
#55878=CARTESIAN_POINT('Ctrl Pts',(-0.710091045131417,0.372756969804615,
-1.18847077789658));
#55879=CARTESIAN_POINT('Ctrl Pts',(-0.762692646653061,0.247945513480473,
-1.18318765446492));
#55880=CARTESIAN_POINT('Ctrl Pts',(-0.782295648551982,0.118150271901965,
-1.17790453103326));
#55881=CARTESIAN_POINT('Ctrl Pts',(-0.788197042334037,0.0790760099322191,
-1.17631407096341));
#55882=CARTESIAN_POINT('Ctrl Pts',(-0.791107827808171,0.0395500757776835,
-1.17472361089355));
#55883=CARTESIAN_POINT('Ctrl Pts',(-0.79107238223822,1.89686955811942E-5,
-1.1731331508237));
#55884=CARTESIAN_POINT('Origin',(0.,0.,-1.94));
#55885=CARTESIAN_POINT('',(-0.791144809354952,-1.43559245109892E-5,-0.944666849176295));
#55886=CARTESIAN_POINT('',(-0.791155923841092,-1.04795641788954E-5,-0.973133150823705));
#55887=CARTESIAN_POINT('',(-0.7911,-9.68818082805471E-17,-1.94));
#55888=CARTESIAN_POINT('Ctrl Pts',(-0.791144809354952,-1.43559245109892E-5,
-0.944666849176295));
#55889=CARTESIAN_POINT('Ctrl Pts',(-0.791047376981328,0.115928204571859,
-0.949332811623831));
#55890=CARTESIAN_POINT('Ctrl Pts',(-0.76524696255707,0.231912697319003,
-0.953998774071366));
#55891=CARTESIAN_POINT('Ctrl Pts',(-0.715892089735664,0.336815212727028,
-0.958664736518902));
#55892=CARTESIAN_POINT('Ctrl Pts',(-0.660009109964346,0.455593051902503,
-0.963947859950562));
#55893=CARTESIAN_POINT('Ctrl Pts',(-0.573928548900091,0.5601634359142,-0.969230983382222));
#55894=CARTESIAN_POINT('Ctrl Pts',(-0.468102600862498,0.637829073291751,
-0.974514106813882));
#55895=CARTESIAN_POINT('Ctrl Pts',(-0.362276652824905,0.715494710669303,
-0.979797230245542));
#55896=CARTESIAN_POINT('Ctrl Pts',(-0.236705317813976,0.766255601412707,
-0.985080353677203));
#55897=CARTESIAN_POINT('Ctrl Pts',(-0.106635894154431,0.783948185627299,
-0.990363477108863));
#55898=CARTESIAN_POINT('Ctrl Pts',(0.0234335295051176,0.801640769841891,
-0.995646600540523));
#55899=CARTESIAN_POINT('Ctrl Pts',(0.158001041813281,0.786265047527667,
-1.00092972397218));
#55900=CARTESIAN_POINT('Ctrl Pts',(0.280726998019134,0.739687991151414,
-1.00621284740384));
#55901=CARTESIAN_POINT('Ctrl Pts',(0.403452954224987,0.693110934775161,
-1.0114959708355));
#55902=CARTESIAN_POINT('Ctrl Pts',(0.514337354328528,0.615332544336879,
-1.01677909426716));
#55903=CARTESIAN_POINT('Ctrl Pts',(0.599916237563637,0.515796936378977,
-1.02206221769882));
#55904=CARTESIAN_POINT('Ctrl Pts',(0.685495120798745,0.416261328421078,
-1.02734534113048));
#55905=CARTESIAN_POINT('Ctrl Pts',(0.74576848716542,0.294968502943563,-1.03262846456214));
#55906=CARTESIAN_POINT('Ctrl Pts',(0.773417739645104,0.166646247100582,
-1.0379115879938));
#55907=CARTESIAN_POINT('Ctrl Pts',(0.801066992124787,0.0383239912576011,
-1.04319471142546));
#55908=CARTESIAN_POINT('Ctrl Pts',(0.796092130717476,-0.0970276949508529,
-1.04847783485713));
#55909=CARTESIAN_POINT('Ctrl Pts',(0.759097220005225,-0.222973949713388,
-1.05376095828878));
#55910=CARTESIAN_POINT('Ctrl Pts',(0.722102309292974,-0.348920204475926,
-1.05904408172044));
#55911=CARTESIAN_POINT('Ctrl Pts',(0.653087349275782,-0.465461027792553,
-1.0643272051521));
#55912=CARTESIAN_POINT('Ctrl Pts',(0.560432370986682,-0.558445636763952,
-1.06961032858377));
#55913=CARTESIAN_POINT('Ctrl Pts',(0.467777392697587,-0.651430245735346,
-1.07489345201542));
#55914=CARTESIAN_POINT('Ctrl Pts',(0.351482396136587,-0.720858640361512,
-1.08017657544709));
#55915=CARTESIAN_POINT('Ctrl Pts',(0.225668315082744,-0.758300588973901,
-1.08545969887875));
#55916=CARTESIAN_POINT('Ctrl Pts',(0.0998542340288942,-0.795742537586291,
-1.09074282231041));
#55917=CARTESIAN_POINT('Ctrl Pts',(-0.0354789315177982,-0.801198040184898,
-1.09602594574207));
#55918=CARTESIAN_POINT('Ctrl Pts',(-0.163898568587665,-0.774004671100481,
-1.10130906917373));
#55919=CARTESIAN_POINT('Ctrl Pts',(-0.292318205657531,-0.746811302016064,
-1.10659219260539));
#55920=CARTESIAN_POINT('Ctrl Pts',(-0.41382431425057,-0.686969061248622,
-1.11187531603705));
#55921=CARTESIAN_POINT('Ctrl Pts',(-0.513663209651773,-0.601744197081025,
-1.11715843946871));
#55922=CARTESIAN_POINT('Ctrl Pts',(-0.613502105052971,-0.516519332913434,
-1.12244156290037));
#55923=CARTESIAN_POINT('Ctrl Pts',(-0.691673787262334,-0.405911845345692,
-1.12772468633203));
#55924=CARTESIAN_POINT('Ctrl Pts',(-0.738686384913777,-0.283352071482572,
-1.13300780976369));
#55925=CARTESIAN_POINT('Ctrl Pts',(-0.773269571419359,-0.193195225672542,
-1.13689415623456));
#55926=CARTESIAN_POINT('Ctrl Pts',(-0.790991646190477,-0.0965706405958467,
-1.14078050270543));
#55927=CARTESIAN_POINT('Ctrl Pts',(-0.791086342131762,2.01490389672293E-5,
-1.1446668491763));
#55928=CARTESIAN_POINT('Ctrl Pts',(-0.79107238223822,1.89686955811942E-5,
-1.1731331508237));
#55929=CARTESIAN_POINT('Ctrl Pts',(-0.790990086203271,-0.0917626946992069,
-1.1694404874619));
#55930=CARTESIAN_POINT('Ctrl Pts',(-0.775025954580806,-0.183572243071071,
-1.16574782410009));
#55931=CARTESIAN_POINT('Ctrl Pts',(-0.743735394388986,-0.269821481033168,
-1.16205516073828));
#55932=CARTESIAN_POINT('Ctrl Pts',(-0.698967736050869,-0.393218965556938,
-1.15677203730662));
#55933=CARTESIAN_POINT('Ctrl Pts',(-0.622828017098433,-0.505234907771603,
-1.15148891387496));
#55934=CARTESIAN_POINT('Ctrl Pts',(-0.524561381012293,-0.5922679512217,
-1.1462057904433));
#55935=CARTESIAN_POINT('Ctrl Pts',(-0.426294744926152,-0.679300994671797,
-1.14092266701163));
#55936=CARTESIAN_POINT('Ctrl Pts',(-0.305901191706306,-0.741351139357328,
-1.13563954357997));
#55937=CARTESIAN_POINT('Ctrl Pts',(-0.177999315812682,-0.770884045796831,
-1.13035642014831));
#55938=CARTESIAN_POINT('Ctrl Pts',(-0.0500974399190584,-0.800416952236334,
-1.12507329671665));
#55939=CARTESIAN_POINT('Ctrl Pts',(0.0853127586483453,-0.797432620429811,
-1.11979017328499));
#55940=CARTESIAN_POINT('Ctrl Pts',(0.21178931330864,-0.762293418089208,
-1.11450704985333));
#55941=CARTESIAN_POINT('Ctrl Pts',(0.338265867968928,-0.727154215748607,
-1.10922392642167));
#55942=CARTESIAN_POINT('Ctrl Pts',(0.455808778722111,-0.659860142873929,
-1.10394080299001));
#55943=CARTESIAN_POINT('Ctrl Pts',(0.55014558580614,-0.568582274531921,
-1.09865767955835));
#55944=CARTESIAN_POINT('Ctrl Pts',(0.644482392890175,-0.477304406189908,
-1.09337455612669));
#55945=CARTESIAN_POINT('Ctrl Pts',(0.715613096305057,-0.362042742380558,
-1.08809143269503));
#55946=CARTESIAN_POINT('Ctrl Pts',(0.754900764262811,-0.236792746107849,
-1.08280830926337));
#55947=CARTESIAN_POINT('Ctrl Pts',(0.794188432220566,-0.11154274983514,
-1.07752518583171));
#55948=CARTESIAN_POINT('Ctrl Pts',(0.801633064721195,0.0236955789009309,
-1.07224206240005));
#55949=CARTESIAN_POINT('Ctrl Pts',(0.776330709181529,0.152501142538597,
-1.06695893896839));
#55950=CARTESIAN_POINT('Ctrl Pts',(0.751028353641863,0.281306706176263,
-1.06167581553673));
#55951=CARTESIAN_POINT('Ctrl Pts',(0.692979010061908,0.403679504715515,
-1.05639269210507));
#55952=CARTESIAN_POINT('Ctrl Pts',(0.609231227053811,0.504760617002139,
-1.05110956867341));
#55953=CARTESIAN_POINT('Ctrl Pts',(0.525483444045717,0.605841729288761,
-1.04582644524175));
#55954=CARTESIAN_POINT('Ctrl Pts',(0.416037221609485,0.685631155322747,
-1.04054332181009));
#55955=CARTESIAN_POINT('Ctrl Pts',(0.294181892090384,0.734440591783975,
-1.03526019837843));
#55956=CARTESIAN_POINT('Ctrl Pts',(0.172326562571282,0.783250028245203,
-1.02997707494677));
#55957=CARTESIAN_POINT('Ctrl Pts',(0.0380621259693093,0.801079475133673,
-1.02469395151511));
#55958=CARTESIAN_POINT('Ctrl Pts',(-0.0923085734470331,0.785764020404375,
-1.01941082808345));
#55959=CARTESIAN_POINT('Ctrl Pts',(-0.222679272863376,0.770448565675077,
-1.01412770465179));
#55960=CARTESIAN_POINT('Ctrl Pts',(-0.349156235094089,0.72198820932801,
-1.00884458122013));
#55961=CARTESIAN_POINT('Ctrl Pts',(-0.456382197479121,0.646267172551726,
-1.00356145778847));
#55962=CARTESIAN_POINT('Ctrl Pts',(-0.563608159864155,0.570546135775441,
-0.998278334356811));
#55963=CARTESIAN_POINT('Ctrl Pts',(-0.651583122403507,0.467564418569935,
-0.992995210925151));
#55964=CARTESIAN_POINT('Ctrl Pts',(-0.709624866111236,0.349826411081959,
-0.987712087493491));
#55965=CARTESIAN_POINT('Ctrl Pts',(-0.763014173696973,0.241525896749369,
-0.982852441936896));
#55966=CARTESIAN_POINT('Ctrl Pts',(-0.791076636121826,0.12073991330517,
-0.9779927963803));
#55967=CARTESIAN_POINT('Ctrl Pts',(-0.791155923841092,-1.04795641788954E-5,
-0.973133150823705));
#55968=CARTESIAN_POINT('Origin',(0.,0.,-1.94));
#55969=CARTESIAN_POINT('',(-0.791032821705865,-2.40842565418786E-7,-0.744666849176295));
#55970=CARTESIAN_POINT('',(-0.791034434997536,-4.6591721334828E-6,-0.773133150823704));
#55971=CARTESIAN_POINT('',(-0.7911,-9.68818082805471E-17,-1.94));
#55972=CARTESIAN_POINT('Ctrl Pts',(-0.791032821705865,-2.40842565418786E-7,
-0.744666849176295));
#55973=CARTESIAN_POINT('Ctrl Pts',(-0.791032120695214,0.065925645056054,
-0.747318873678916));
#55974=CARTESIAN_POINT('Ctrl Pts',(-0.782881257592987,0.13185170122012,
-0.749970898181537));
#55975=CARTESIAN_POINT('Ctrl Pts',(-0.766582283740692,0.19569765947848,
-0.752622922684158));
#55976=CARTESIAN_POINT('Ctrl Pts',(-0.734112941701818,0.322885804896515,
-0.757906046115818));
#55977=CARTESIAN_POINT('Ctrl Pts',(-0.669307817269351,0.441819080529466,
-0.763189169547478));
#55978=CARTESIAN_POINT('Ctrl Pts',(-0.580035768930037,0.538056203785618,
-0.768472292979138));
#55979=CARTESIAN_POINT('Ctrl Pts',(-0.490763720590723,0.634293327041769,
-0.773755416410798));
#55980=CARTESIAN_POINT('Ctrl Pts',(-0.377024748344561,0.707834297921121,
-0.779038539842458));
#55981=CARTESIAN_POINT('Ctrl Pts',(-0.252629424810162,0.749749521767461,
-0.784321663274118));
#55982=CARTESIAN_POINT('Ctrl Pts',(-0.128234101275767,0.791664745613799,
-0.789604786705778));
#55983=CARTESIAN_POINT('Ctrl Pts',(0.00681757354686521,0.801954222427127,
-0.794887910137438));
#55984=CARTESIAN_POINT('Ctrl Pts',(0.136127166248591,0.77936856895796,-0.800171033569098));
#55985=CARTESIAN_POINT('Ctrl Pts',(0.265436758950324,0.756782915488791,
-0.805454157000758));
#55986=CARTESIAN_POINT('Ctrl Pts',(0.389004269531151,0.701322131737123,
-0.810737280432419));
#55987=CARTESIAN_POINT('Ctrl Pts',(0.491825710839823,0.619720454582025,
-0.816020403864079));
#55988=CARTESIAN_POINT('Ctrl Pts',(0.594647152148495,0.538118777426927,
-0.821303527295739));
#55989=CARTESIAN_POINT('Ctrl Pts',(0.676722524185013,0.4303762068684,-0.826586650727399));
#55990=CARTESIAN_POINT('Ctrl Pts',(0.728085956295501,0.30957521204986,-0.831869774159059));
#55991=CARTESIAN_POINT('Ctrl Pts',(0.779449388405989,0.18877421723132,-0.837152897590719));
#55992=CARTESIAN_POINT('Ctrl Pts',(0.800100880590446,0.0549147981527687,
-0.84243602102238));
#55993=CARTESIAN_POINT('Ctrl Pts',(0.787532858471651,-0.0757493795216767,
-0.84771914445404));
#55994=CARTESIAN_POINT('Ctrl Pts',(0.774964836352857,-0.206413557196118,
-0.8530022678857));
#55995=CARTESIAN_POINT('Ctrl Pts',(0.729177299930812,-0.333882493466454,
-0.85828539131736));
#55996=CARTESIAN_POINT('Ctrl Pts',(0.655729927513629,-0.442678476812936,
-0.86356851474902));
#55997=CARTESIAN_POINT('Ctrl Pts',(0.582282555096445,-0.551474460159418,
-0.86885163818068));
#55998=CARTESIAN_POINT('Ctrl Pts',(0.481175346684122,-0.641597490582047,
-0.87413476161234));
#55999=CARTESIAN_POINT('Ctrl Pts',(0.364685083194123,-0.702104523391029,
-0.879417885044));
#56000=CARTESIAN_POINT('Ctrl Pts',(0.248194819704125,-0.762611556200011,
-0.88470100847566));
#56001=CARTESIAN_POINT('Ctrl Pts',(0.11632150113645,-0.793502591395346,
-0.88998413190732));
#56002=CARTESIAN_POINT('Ctrl Pts',(-0.0149223659197404,-0.791026734482348,
-0.89526725533898));
#56003=CARTESIAN_POINT('Ctrl Pts',(-0.146166232975938,-0.78855087756935,
-0.90055037877064));
#56004=CARTESIAN_POINT('Ctrl Pts',(-0.276780648520651,-0.752708128548016,
-0.905833502202301));
#56005=CARTESIAN_POINT('Ctrl Pts',(-0.390905966248882,-0.687850635837082,
-0.911116625633962));
#56006=CARTESIAN_POINT('Ctrl Pts',(-0.505031283977106,-0.622993143126152,
-0.916399749065622));
#56007=CARTESIAN_POINT('Ctrl Pts',(-0.602667503888851,-0.529120906725625,
-0.921682872497282));
#56008=CARTESIAN_POINT('Ctrl Pts',(-0.671959304288581,-0.417632212659005,
-0.926965995928942));
#56009=CARTESIAN_POINT('Ctrl Pts',(-0.74125110468831,-0.306143518592384,
-0.932249119360602));
#56010=CARTESIAN_POINT('Ctrl Pts',(-0.782198485576025,-0.177038366859669,
-0.937532242792262));
#56011=CARTESIAN_POINT('Ctrl Pts',(-0.789829476780693,-0.0459931438236847,
-0.942815366223922));
#56012=CARTESIAN_POINT('Ctrl Pts',(-0.790720909680688,-0.0306847756093432,
-0.943432527208046));
#56013=CARTESIAN_POINT('Ctrl Pts',(-0.791157696612461,-0.0153499325697136,
-0.94404968819217));
#56014=CARTESIAN_POINT('Ctrl Pts',(-0.791144809354952,-1.43559245109892E-5,
-0.944666849176295));
#56015=CARTESIAN_POINT('Ctrl Pts',(-0.791155923841092,-1.04795641788954E-5,
-0.973133150823705));
#56016=CARTESIAN_POINT('Ctrl Pts',(-0.791162833109368,-0.0105328765558965,
-0.97270967294864));
#56017=CARTESIAN_POINT('Ctrl Pts',(-0.790957247118644,-0.0210550032841967,
-0.972286195073575));
#56018=CARTESIAN_POINT('Ctrl Pts',(-0.790537408105818,-0.031568574234663,
-0.971862717198511));
#56019=CARTESIAN_POINT('Ctrl Pts',(-0.785299681516566,-0.162731254292855,
-0.96657959376685));
#56020=CARTESIAN_POINT('Ctrl Pts',(-0.746715703461958,-0.292562316638795,
-0.96129647033519));
#56021=CARTESIAN_POINT('Ctrl Pts',(-0.679470471707622,-0.405297232375568,
-0.95601334690353));
#56022=CARTESIAN_POINT('Ctrl Pts',(-0.612225239953286,-0.518032148112341,
-0.95073022347187));
#56023=CARTESIAN_POINT('Ctrl Pts',(-0.516318754499222,-0.613670917239946,
-0.94544710004021));
#56024=CARTESIAN_POINT('Ctrl Pts',(-0.4033963068036,-0.680600755326564,
-0.94016397660855));
#56025=CARTESIAN_POINT('Ctrl Pts',(-0.290473859107974,-0.747530593413184,
-0.93488085317689));
#56026=CARTESIAN_POINT('Ctrl Pts',(-0.160535449170788,-0.785751500458815,
-0.92959772974523));
#56027=CARTESIAN_POINT('Ctrl Pts',(-0.0293586403983704,-0.790622564013849,
-0.924314606313569));
#56028=CARTESIAN_POINT('Ctrl Pts',(0.101818168374047,-0.795493627568883,
-0.919031482881909));
#56029=CARTESIAN_POINT('Ctrl Pts',(0.234233375981696,-0.767014847633319,
-0.913748359450248));
#56030=CARTESIAN_POINT('Ctrl Pts',(0.351808677826252,-0.70864421446874,
-0.908465236018588));
#56031=CARTESIAN_POINT('Ctrl Pts',(0.469383979670803,-0.650273581304164,
-0.903182112586928));
#56032=CARTESIAN_POINT('Ctrl Pts',(0.572119375752263,-0.562011094910577,
-0.897898989155269));
#56033=CARTESIAN_POINT('Ctrl Pts',(0.647540385072036,-0.454573886397616,
-0.892615865723609));
#56034=CARTESIAN_POINT('Ctrl Pts',(0.722961394391813,-0.34713667788465,
-0.887332742291949));
#56035=CARTESIAN_POINT('Ctrl Pts',(0.7710680169499,-0.220524747252309,-0.882049618860289));
#56036=CARTESIAN_POINT('Ctrl Pts',(0.786018983116774,-0.0901117454827402,
-0.876766495428628));
#56037=CARTESIAN_POINT('Ctrl Pts',(0.800969949283647,0.040301256286821,
-0.871483371996968));
#56038=CARTESIAN_POINT('Ctrl Pts',(0.782765259059311,0.17451532919361,-0.866200248565308));
#56039=CARTESIAN_POINT('Ctrl Pts',(0.733615387810102,0.296233744300185,
-0.860917125133648));
#56040=CARTESIAN_POINT('Ctrl Pts',(0.68446551656089,0.417952159406768,-0.855634001701988));
#56041=CARTESIAN_POINT('Ctrl Pts',(0.604370464286801,0.527174916713137,
-0.850350878270329));
#56042=CARTESIAN_POINT('Ctrl Pts',(0.50305564448488,0.61063981776967,-0.845067754838668));
#56043=CARTESIAN_POINT('Ctrl Pts',(0.401740824682959,0.694104718826203,
-0.839784631407008));
#56044=CARTESIAN_POINT('Ctrl Pts',(0.279206237353206,0.7518117636329,-0.834501507975347));
#56045=CARTESIAN_POINT('Ctrl Pts',(0.15033044859473,0.776753966658157,-0.829218384543687));
#56046=CARTESIAN_POINT('Ctrl Pts',(0.0214546598362535,0.801696169683414,
-0.823935261112027));
#56047=CARTESIAN_POINT('Ctrl Pts',(-0.113762330350946,0.79387353092723,
-0.818652137680367));
#56048=CARTESIAN_POINT('Ctrl Pts',(-0.238902015404239,0.7542359017772,-0.813369014248707));
#56049=CARTESIAN_POINT('Ctrl Pts',(-0.364041700457527,0.714598272627171,
-0.808085890817047));
#56050=CARTESIAN_POINT('Ctrl Pts',(-0.479104080376909,0.643145653083297,
-0.802802767385386));
#56051=CARTESIAN_POINT('Ctrl Pts',(-0.570117889885716,0.548554063084152,
-0.797519643953726));
#56052=CARTESIAN_POINT('Ctrl Pts',(-0.661131699394522,0.453962473085008,
-0.792236520522066));
#56053=CARTESIAN_POINT('Ctrl Pts',(-0.728096938492752,0.336231912630593,
-0.786953397090406));
#56054=CARTESIAN_POINT('Ctrl Pts',(-0.762882460228531,0.209657626547513,
-0.781670273658746));
#56055=CARTESIAN_POINT('Ctrl Pts',(-0.7816193732044,0.141479509187784,-0.778824566047066));
#56056=CARTESIAN_POINT('Ctrl Pts',(-0.791019847233727,0.0707355239100122,
-0.775978858435385));
#56057=CARTESIAN_POINT('Ctrl Pts',(-0.791034434997536,-4.65917213348279E-6,
-0.773133150823704));
#56058=CARTESIAN_POINT('Origin',(0.,0.,-1.94));
#56059=CARTESIAN_POINT('',(-0.791143457346284,1.47250900771681E-5,-0.544666849176294));
#56060=CARTESIAN_POINT('',(-0.791129915139071,1.76226913310852E-5,-0.573133150823703));
#56061=CARTESIAN_POINT('',(-0.7911,-9.68818082805471E-17,-1.94));
#56062=CARTESIAN_POINT('Ctrl Pts',(-0.791143457346284,1.47250900771681E-5,
-0.544666849176294));
#56063=CARTESIAN_POINT('Ctrl Pts',(-0.791157032798385,0.0158703510580344,
-0.545304935734));
#56064=CARTESIAN_POINT('Ctrl Pts',(-0.790690104471727,0.0317251781600011,
-0.545943022291706));
#56065=CARTESIAN_POINT('Ctrl Pts',(-0.789737233642478,0.0475507462532112,
-0.546581108849412));
#56066=CARTESIAN_POINT('Ctrl Pts',(-0.781847811518544,0.178580664691211,
-0.551864232281072));
#56067=CARTESIAN_POINT('Ctrl Pts',(-0.740645890688464,0.307604809429334,
-0.557147355712733));
#56068=CARTESIAN_POINT('Ctrl Pts',(-0.671134348428437,0.418956630249429,
-0.562430479144392));
#56069=CARTESIAN_POINT('Ctrl Pts',(-0.601622806168408,0.530308451069527,
-0.567713602576053));
#56070=CARTESIAN_POINT('Ctrl Pts',(-0.50380164247843,0.623987947971596,
-0.572996726007712));
#56071=CARTESIAN_POINT('Ctrl Pts',(-0.38954863555615,0.688620238017154,
-0.578279849439373));
#56072=CARTESIAN_POINT('Ctrl Pts',(-0.27529562863387,0.753252528062712,
-0.583562972871033));
#56073=CARTESIAN_POINT('Ctrl Pts',(-0.144610778479288,0.78883761125176,
-0.588846096302693));
#56074=CARTESIAN_POINT('Ctrl Pts',(-0.0133622838071854,0.791054625826753,
-0.594129219734354));
#56075=CARTESIAN_POINT('Ctrl Pts',(0.117886210864914,0.793271640401747,
-0.599412343166014));
#56076=CARTESIAN_POINT('Ctrl Pts',(0.249698350054534,0.762120586362689,
-0.604695466597674));
#56077=CARTESIAN_POINT('Ctrl Pts',(0.366069055780573,0.701383930576091,
-0.609978590029334));
#56078=CARTESIAN_POINT('Ctrl Pts',(0.482439761506612,0.640647274789494,
-0.615261713460994));
#56079=CARTESIAN_POINT('Ctrl Pts',(0.583369033769069,0.550325017255357,
-0.620544836892654));
#56080=CARTESIAN_POINT('Ctrl Pts',(0.656601697262608,0.441384393496546,
-0.625827960324314));
#56081=CARTESIAN_POINT('Ctrl Pts',(0.729834360756149,0.332443769737732,
-0.631111083755974));
#56082=CARTESIAN_POINT('Ctrl Pts',(0.775370415480771,0.204884779754242,
-0.636394207187635));
#56083=CARTESIAN_POINT('Ctrl Pts',(0.787680718890875,0.0741960696937758,
-0.641677330619295));
#56084=CARTESIAN_POINT('Ctrl Pts',(0.799991022300978,-0.0564926403666832,
-0.646960454050955));
#56085=CARTESIAN_POINT('Ctrl Pts',(0.779075574396567,-0.190311070504119,
-0.652243577482614));
#56086=CARTESIAN_POINT('Ctrl Pts',(0.727473999955588,-0.311010532070969,
-0.657526700914274));
#56087=CARTESIAN_POINT('Ctrl Pts',(0.675872425514605,-0.431709993637826,
-0.662809824345935));
#56088=CARTESIAN_POINT('Ctrl Pts',(0.59358472453705,-0.539290486634097,
-0.668092947777595));
#56089=CARTESIAN_POINT('Ctrl Pts',(0.490602549378544,-0.620689221924888,
-0.673376071209255));
#56090=CARTESIAN_POINT('Ctrl Pts',(0.387620374220037,-0.702087957215679,
-0.678659194640915));
#56091=CARTESIAN_POINT('Ctrl Pts',(0.263943724880579,-0.75730493480099,
-0.683942318072575));
#56092=CARTESIAN_POINT('Ctrl Pts',(0.134589840510463,-0.779635521575189,
-0.689225441504236));
#56093=CARTESIAN_POINT('Ctrl Pts',(0.00523595614035394,-0.801966108349387,
-0.694508564935896));
#56094=CARTESIAN_POINT('Ctrl Pts',(-0.129795163260413,-0.791410304312477,
-0.699791688367556));
#56095=CARTESIAN_POINT('Ctrl Pts',(-0.254107580191888,-0.7492498310707,
-0.705074811799216));
#56096=CARTESIAN_POINT('Ctrl Pts',(-0.378419997123371,-0.70708935782892,
-0.710357935230876));
#56097=CARTESIAN_POINT('Ctrl Pts',(-0.49201371158556,-0.63332421538227,
-0.715641058662536));
#56098=CARTESIAN_POINT('Ctrl Pts',(-0.581095788653718,-0.536911218060642,
-0.720924182094196));
#56099=CARTESIAN_POINT('Ctrl Pts',(-0.670177865721877,-0.440498220739014,
-0.726207305525856));
#56100=CARTESIAN_POINT('Ctrl Pts',(-0.734748305396003,-0.321437368542408,
-0.731490428957517));
#56101=CARTESIAN_POINT('Ctrl Pts',(-0.766966745410426,-0.194185434842544,
-0.736773552389177));
#56102=CARTESIAN_POINT('Ctrl Pts',(-0.783012159475383,-0.130811479869343,
-0.739404651318217));
#56103=CARTESIAN_POINT('Ctrl Pts',(-0.791033517185251,-0.0654059441505127,
-0.742035750247256));
#56104=CARTESIAN_POINT('Ctrl Pts',(-0.791032821705865,-2.40842565418786E-7,
-0.744666849176295));
#56105=CARTESIAN_POINT('Ctrl Pts',(-0.791034434997536,-4.65917213348279E-6,
-0.773133150823704));
#56106=CARTESIAN_POINT('Ctrl Pts',(-0.791046929761981,-0.0605952977342058,
-0.770695735003725));
#56107=CARTESIAN_POINT('Ctrl Pts',(-0.784173631136982,-0.12118314688111,
-0.768258319183745));
#56108=CARTESIAN_POINT('Ctrl Pts',(-0.770383467724153,-0.180153493308298,
-0.765820903363765));
#56109=CARTESIAN_POINT('Ctrl Pts',(-0.740493149110667,-0.307972315369276,
-0.760537779932105));
#56110=CARTESIAN_POINT('Ctrl Pts',(-0.678106707510369,-0.428191947779487,
-0.755254656500445));
#56111=CARTESIAN_POINT('Ctrl Pts',(-0.590799316719212,-0.526214914134886,
-0.749971533068785));
#56112=CARTESIAN_POINT('Ctrl Pts',(-0.503491925928054,-0.624237880490285,
-0.744688409637125));
#56113=CARTESIAN_POINT('Ctrl Pts',(-0.391263585946037,-0.700064180790871,
-0.739405286205465));
#56114=CARTESIAN_POINT('Ctrl Pts',(-0.26774144328749,-0.744486727914074,
-0.734122162773805));
#56115=CARTESIAN_POINT('Ctrl Pts',(-0.144219300628944,-0.788909275037278,
-0.728839039342145));
#56116=CARTESIAN_POINT('Ctrl Pts',(-0.00940335529385652,-0.8019280689831,
-0.723555915910484));
#56117=CARTESIAN_POINT('Ctrl Pts',(0.120336582384249,-0.781962323538643,
-0.718272792478824));
#56118=CARTESIAN_POINT('Ctrl Pts',(0.250076520062358,-0.761996578094185,
-0.712989669047164));
#56119=CARTESIAN_POINT('Ctrl Pts',(0.374740450083486,-0.709046293259455,
-0.707706545615504));
#56120=CARTESIAN_POINT('Ctrl Pts',(0.479191254321141,-0.629540872601617,
-0.702423422183844));
#56121=CARTESIAN_POINT('Ctrl Pts',(0.583642058558793,-0.550035451943781,
-0.697140298752184));
#56122=CARTESIAN_POINT('Ctrl Pts',(0.667879737012961,-0.443974895462845,
-0.691857175320524));
#56123=CARTESIAN_POINT('Ctrl Pts',(0.721675864434676,-0.324237436435612,
-0.686574051888864));
#56124=CARTESIAN_POINT('Ctrl Pts',(0.775471991856391,-0.204499977408379,
-0.681290928457204));
#56125=CARTESIAN_POINT('Ctrl Pts',(0.798826568245652,-0.0710856158348409,
-0.676007805025542));
#56126=CARTESIAN_POINT('Ctrl Pts',(0.788903801553075,0.0598060230159138,
-0.670724681593883));
#56127=CARTESIAN_POINT('Ctrl Pts',(0.778981034860496,0.190697661866672,
-0.665441558162223));
#56128=CARTESIAN_POINT('Ctrl Pts',(0.73578092508608,0.319066577994655,-0.660158434730563));
#56129=CARTESIAN_POINT('Ctrl Pts',(0.664548976399496,0.429325781266692,
-0.654875311298903));
#56130=CARTESIAN_POINT('Ctrl Pts',(0.593317027712914,0.539584984538727,
-0.649592187867243));
#56131=CARTESIAN_POINT('Ctrl Pts',(0.494053240114169,0.631734474954815,
-0.644309064435582));
#56132=CARTESIAN_POINT('Ctrl Pts',(0.378810560099591,0.694585148164649,
-0.639025941003921));
#56133=CARTESIAN_POINT('Ctrl Pts',(0.263567880085013,0.757435821374483,
-0.633742817572261));
#56134=CARTESIAN_POINT('Ctrl Pts',(0.132346307654605,0.79098767737806,-0.628459694140602));
#56135=CARTESIAN_POINT('Ctrl Pts',(0.00107921216619798,0.791166735773803,
-0.623176570708942));
#56136=CARTESIAN_POINT('Ctrl Pts',(-0.130187883322209,0.791345794169545,
-0.617893447277282));
#56137=CARTESIAN_POINT('Ctrl Pts',(-0.261500501868612,0.758152054957453,
-0.612610323845622));
#56138=CARTESIAN_POINT('Ctrl Pts',(-0.376914218986303,0.695616014781013,
-0.607327200413961));
#56139=CARTESIAN_POINT('Ctrl Pts',(-0.492327936103994,0.633079974604573,
-0.602044076982301));
#56140=CARTESIAN_POINT('Ctrl Pts',(-0.591842751792971,0.541201633463786,
-0.596760953550642));
#56141=CARTESIAN_POINT('Ctrl Pts',(-0.663375238872918,0.431137171842295,
-0.591477830118981));
#56142=CARTESIAN_POINT('Ctrl Pts',(-0.73490772595287,0.321072710220798,
-0.586194706687321));
#56143=CARTESIAN_POINT('Ctrl Pts',(-0.778457884423789,0.192822128118595,
-0.580911583255661));
#56144=CARTESIAN_POINT('Ctrl Pts',(-0.78873770601343,0.0619580471492215,
-0.575628459824));
#56145=CARTESIAN_POINT('Ctrl Pts',(-0.790356150838471,0.0413549371845394,
-0.574796690157235));
#56146=CARTESIAN_POINT('Ctrl Pts',(-0.791149922541304,0.0206870463227368,
-0.573964920490469));
#56147=CARTESIAN_POINT('Ctrl Pts',(-0.791129915139071,1.76226913310852E-5,
-0.573133150823703));
#56148=CARTESIAN_POINT('Origin',(0.,0.,-1.94));
#56149=CARTESIAN_POINT('',(-0.791087916566115,-2.02165423325296E-5,-0.344666849176295));
#56150=CARTESIAN_POINT('',(-0.791102868091814,-2.02590743034978E-5,-0.373133150823704));
#56151=CARTESIAN_POINT('',(-0.7911,-9.68818082805471E-17,-1.94));
#56152=CARTESIAN_POINT('Ctrl Pts',(-0.791087916566115,-2.02165423325296E-5,
-0.344666849176295));
#56153=CARTESIAN_POINT('Ctrl Pts',(-0.790992060355861,0.097090099215087,
-0.348574121220746));
#56154=CARTESIAN_POINT('Ctrl Pts',(-0.773074216505353,0.194234811893738,
-0.352481393265196));
#56155=CARTESIAN_POINT('Ctrl Pts',(-0.738126125034402,0.284808348566891,
-0.356388665309647));
#56156=CARTESIAN_POINT('Ctrl Pts',(-0.690871908066276,0.407275166449671,
-0.361671788741307));
#56157=CARTESIAN_POINT('Ctrl Pts',(-0.612482238925616,0.517728269629272,
-0.366954912172967));
#56158=CARTESIAN_POINT('Ctrl Pts',(-0.512475458209948,0.602756067010894,
-0.372238035604627));
#56159=CARTESIAN_POINT('Ctrl Pts',(-0.412468677494272,0.687783864392524,
-0.377521159036288));
#56160=CARTESIAN_POINT('Ctrl Pts',(-0.290844785203582,0.747386355976171,
-0.382804282467948));
#56161=CARTESIAN_POINT('Ctrl Pts',(-0.162371767485705,0.774326404571983,
-0.388087405899608));
#56162=CARTESIAN_POINT('Ctrl Pts',(-0.0338987497678321,0.801266453167794,
-0.393370529331269));
#56163=CARTESIAN_POINT('Ctrl Pts',(0.101423393377231,0.795544058775773,
-0.398653652762929));
#56164=CARTESIAN_POINT('Ctrl Pts',(0.227163387222433,0.757854054008525,
-0.403936776194589));
#56165=CARTESIAN_POINT('Ctrl Pts',(0.352903381067629,0.72016404924128,-0.409219899626249));
#56166=CARTESIAN_POINT('Ctrl Pts',(0.469061225612968,0.65050643409881,-0.414503023057909));
#56167=CARTESIAN_POINT('Ctrl Pts',(0.561532640612168,0.557339272966225,
-0.419786146489568));
#56168=CARTESIAN_POINT('Ctrl Pts',(0.654004055611374,0.464172111833635,
-0.425069269921229));
#56169=CARTESIAN_POINT('Ctrl Pts',(0.72278904106444,0.347495404710924,-0.430352393352889));
#56170=CARTESIAN_POINT('Ctrl Pts',(0.75953549019646,0.221476433980054,-0.435635516784549));
#56171=CARTESIAN_POINT('Ctrl Pts',(0.796281939328478,0.0954574632491873,
-0.44091864021621));
#56172=CARTESIAN_POINT('Ctrl Pts',(0.800989852139453,-0.0399037710898398,
-0.44620176364787));
#56173=CARTESIAN_POINT('Ctrl Pts',(0.773087577871225,-0.168171247863792,
-0.45148488707953));
#56174=CARTESIAN_POINT('Ctrl Pts',(0.745185303602996,-0.296438724637747,
-0.45676801051119));
#56175=CARTESIAN_POINT('Ctrl Pts',(0.684672842255569,-0.417612443846618,
-0.46205113394285));
#56176=CARTESIAN_POINT('Ctrl Pts',(0.5988978225636,-0.516979080621905,-0.46733425737451));
#56177=CARTESIAN_POINT('Ctrl Pts',(0.513122802871631,-0.616345717397192,
-0.47261738080617));
#56178=CARTESIAN_POINT('Ctrl Pts',(0.402085224835124,-0.693905271738887,
-0.47790050423783));
#56179=CARTESIAN_POINT('Ctrl Pts',(0.279267648610165,-0.74024019892847,
-0.483183627669491));
#56180=CARTESIAN_POINT('Ctrl Pts',(0.156450072385206,-0.786575126118053,
-0.488466751101151));
#56181=CARTESIAN_POINT('Ctrl Pts',(0.0218524979717924,-0.801685426155526,
-0.493749874532811));
#56182=CARTESIAN_POINT('Ctrl Pts',(-0.108181779638531,-0.783736355048523,
-0.499032997964471));
#56183=CARTESIAN_POINT('Ctrl Pts',(-0.238216057248851,-0.765787283941521,
-0.504316121396131));
#56184=CARTESIAN_POINT('Ctrl Pts',(-0.363687038056083,-0.714778841690045,
-0.509599244827791));
#56185=CARTESIAN_POINT('Ctrl Pts',(-0.469359609082811,-0.636904646734636,
-0.514882368259451));
#56186=CARTESIAN_POINT('Ctrl Pts',(-0.57503218010954,-0.559030451779227,
-0.520165491691111));
#56187=CARTESIAN_POINT('Ctrl Pts',(-0.660906341355765,-0.454290504119883,
-0.525448615122772));
#56188=CARTESIAN_POINT('Ctrl Pts',(-0.716554960269984,-0.335402684221274,
-0.530731738554432));
#56189=CARTESIAN_POINT('Ctrl Pts',(-0.765482434743157,-0.230873930646506,
-0.535376775428386));
#56190=CARTESIAN_POINT('Ctrl Pts',(-0.791044633017785,-0.115408435594574,
-0.54002181230234));
#56191=CARTESIAN_POINT('Ctrl Pts',(-0.791143457346284,1.47250900771681E-5,
-0.544666849176294));
#56192=CARTESIAN_POINT('Ctrl Pts',(-0.791129915139071,1.76226913310852E-5,
-0.573133150823703));
#56193=CARTESIAN_POINT('Ctrl Pts',(-0.791022842197109,-0.110598236934363,
-0.568681797058809));
#56194=CARTESIAN_POINT('Ctrl Pts',(-0.767608864627571,-0.221257995592029,
-0.564230443293914));
#56195=CARTESIAN_POINT('Ctrl Pts',(-0.722557746651952,-0.322267390914949,
-0.55977908952902));
#56196=CARTESIAN_POINT('Ctrl Pts',(-0.669088480992473,-0.442151168173203,
-0.55449596609736));
#56197=CARTESIAN_POINT('Ctrl Pts',(-0.585140464965152,-0.548441142853183,
-0.5492128426657));
#56198=CARTESIAN_POINT('Ctrl Pts',(-0.480906952022514,-0.628231224940537,
-0.54392971923404));
#56199=CARTESIAN_POINT('Ctrl Pts',(-0.37667343907987,-0.708021307027895,
-0.538646595802379));
#56200=CARTESIAN_POINT('Ctrl Pts',(-0.252154429221904,-0.761311496522626,
-0.533363472370719));
#56201=CARTESIAN_POINT('Ctrl Pts',(-0.122469443876305,-0.781631117478379,
-0.528080348939059));
#56202=CARTESIAN_POINT('Ctrl Pts',(0.00721554146929006,-0.801950738434132,
-0.522797225507399));
#56203=CARTESIAN_POINT('Ctrl Pts',(0.142066502302521,-0.789299790850911,
-0.517514102075739));
#56204=CARTESIAN_POINT('Ctrl Pts',(0.265709376589039,-0.745214395785903,
-0.512230978644079));
#56205=CARTESIAN_POINT('Ctrl Pts',(0.389352250875561,-0.701129000720895,
-0.506947855212419));
#56206=CARTESIAN_POINT('Ctrl Pts',(0.501787038615372,-0.625609158174098,
-0.501664731780758));
#56207=CARTESIAN_POINT('Ctrl Pts',(0.589361525705732,-0.527824744125977,
-0.496381608349098));
#56208=CARTESIAN_POINT('Ctrl Pts',(0.676936012796088,-0.430040330077863,
-0.491098484917439));
#56209=CARTESIAN_POINT('Ctrl Pts',(0.739650199236998,-0.309991344528425,
-0.485815361485779));
#56210=CARTESIAN_POINT('Ctrl Pts',(0.769889115339775,-0.182254543359766,
-0.480532238054119));
#56211=CARTESIAN_POINT('Ctrl Pts',(0.800128031442554,-0.0545177421910954,
-0.475249114622459));
#56212=CARTESIAN_POINT('Ctrl Pts',(0.797891677207195,0.0809068745967896,
-0.469965991190798));
#56213=CARTESIAN_POINT('Ctrl Pts',(0.763451598366819,0.207575589713544,
-0.464682867759138));
#56214=CARTESIAN_POINT('Ctrl Pts',(0.729011519526445,0.334244304830287,
-0.459399744327478));
#56215=CARTESIAN_POINT('Ctrl Pts',(0.662367716081058,0.452157118275893,
-0.454116620895818));
#56216=CARTESIAN_POINT('Ctrl Pts',(0.571612305172384,0.546996655446337,
-0.448833497464158));
#56217=CARTESIAN_POINT('Ctrl Pts',(0.480856894263705,0.641836192616787,
-0.443550374032498));
#56218=CARTESIAN_POINT('Ctrl Pts',(0.365989875891734,0.713602453512075,
-0.438267250600838));
#56219=CARTESIAN_POINT('Ctrl Pts',(0.240958793871168,0.753581334794116,
-0.432984127169178));
#56220=CARTESIAN_POINT('Ctrl Pts',(0.115927711850602,0.793560216076158,
-0.427701003737517));
#56221=CARTESIAN_POINT('Ctrl Pts',(-0.0192674338185621,0.801751717744953,
-0.422417880305857));
#56222=CARTESIAN_POINT('Ctrl Pts',(-0.148210789011595,0.777161199825293,
-0.417134756874197));
#56223=CARTESIAN_POINT('Ctrl Pts',(-0.277154144204628,0.752570681905633,
-0.411851633442537));
#56224=CARTESIAN_POINT('Ctrl Pts',(-0.399845708921533,0.695198144397515,
-0.406568510010877));
#56225=CARTESIAN_POINT('Ctrl Pts',(-0.501387856330821,0.612009955817321,
-0.401285386579216));
#56226=CARTESIAN_POINT('Ctrl Pts',(-0.602930003740106,0.528821767237129,
-0.396002263147556));
#56227=CARTESIAN_POINT('Ctrl Pts',(-0.683322733841777,0.419817927584861,
-0.390719139715896));
#56228=CARTESIAN_POINT('Ctrl Pts',(-0.732804488093843,0.298234053588397,
-0.385436016284236));
#56229=CARTESIAN_POINT('Ctrl Pts',(-0.771214049734729,0.203856168782306,
-0.381335061130725));
#56230=CARTESIAN_POINT('Ctrl Pts',(-0.790998398675608,0.101898263967332,
-0.377234105977215));
#56231=CARTESIAN_POINT('Ctrl Pts',(-0.791102868091814,-2.02590743034978E-5,
-0.373133150823704));
#56232=CARTESIAN_POINT('Origin',(0.,0.,-1.94));
#56233=CARTESIAN_POINT('',(-0.791054317571617,1.54395522024842E-5,-0.144666849176294));
#56234=CARTESIAN_POINT('',(-0.791044518748003,1.1964098827608E-5,-0.173133150823703));
#56235=CARTESIAN_POINT('',(-0.7911,-9.68818082805471E-17,-1.94));
#56236=CARTESIAN_POINT('Ctrl Pts',(-0.791054317571617,1.54395522024842E-5,
-0.144666849176294));
#56237=CARTESIAN_POINT('Ctrl Pts',(-0.79108665330085,0.0470775663249256,
-0.14656018327583));
#56238=CARTESIAN_POINT('Ctrl Pts',(-0.786954227878093,0.0941339831305366,
-0.148453517375366));
#56239=CARTESIAN_POINT('Ctrl Pts',(-0.778604014212082,0.140429697846895,
-0.150346851474902));
#56240=CARTESIAN_POINT('Ctrl Pts',(-0.755303736945075,0.269612378950766,
-0.155629974906562));
#56241=CARTESIAN_POINT('Ctrl Pts',(-0.699162807492777,0.392872061722574,
-0.160913098338222));
#56242=CARTESIAN_POINT('Ctrl Pts',(-0.616994819475088,0.495241307414285,
-0.166196221769883));
#56243=CARTESIAN_POINT('Ctrl Pts',(-0.5348268314574,0.597610553105996,-0.171479345201543));
#56244=CARTESIAN_POINT('Ctrl Pts',(-0.426631784874323,0.679089361717608,
-0.176762468633203));
#56245=CARTESIAN_POINT('Ctrl Pts',(-0.305548738351313,0.729784722528592,
-0.182045592064863));
#56246=CARTESIAN_POINT('Ctrl Pts',(-0.184465691828305,0.780480083339574,
-0.187328715496523));
#56247=CARTESIAN_POINT('Ctrl Pts',(-0.0504946453653669,0.800391996349929,
-0.192611838928183));
#56248=CARTESIAN_POINT('Ctrl Pts',(0.0800980227545852,0.787102473350495,
-0.197894962359843));
#56249=CARTESIAN_POINT('Ctrl Pts',(0.210690690874534,0.77381295035106,-0.203178085791503));
#56250=CARTESIAN_POINT('Ctrl Pts',(0.337904980651504,0.727321991341834,
-0.208461209223164));
#56251=CARTESIAN_POINT('Ctrl Pts',(0.446293670933016,0.653274796900439,
-0.213744332654824));
#56252=CARTESIAN_POINT('Ctrl Pts',(0.554682361214537,0.579227602459038,
-0.219027456086484));
#56253=CARTESIAN_POINT('Ctrl Pts',(0.644245452000599,0.477624172585471,
-0.224310579518144));
#56254=CARTESIAN_POINT('Ctrl Pts',(0.704108107756478,0.360801484773388,
-0.229593702949804));
#56255=CARTESIAN_POINT('Ctrl Pts',(0.763970763512355,0.243978796961309,
-0.234876826381464));
#56256=CARTESIAN_POINT('Ctrl Pts',(0.794132984238041,0.111936851210725,
-0.240159949813125));
#56257=CARTESIAN_POINT('Ctrl Pts',(0.790932258558706,-0.0192913418477741,
-0.245443073244785));
#56258=CARTESIAN_POINT('Ctrl Pts',(0.787731532879371,-0.150519534906269,
-0.250726196676446));
#56259=CARTESIAN_POINT('Ctrl Pts',(0.751167860795012,-0.280933975272688,
-0.256009320108106));
#56260=CARTESIAN_POINT('Ctrl Pts',(0.685680984842779,-0.394699312989822,
-0.261292443539766));
#56261=CARTESIAN_POINT('Ctrl Pts',(0.620194108890548,-0.508464650706953,
-0.266575566971426));
#56262=CARTESIAN_POINT('Ctrl Pts',(0.525784029070445,-0.60558088577481,
-0.271858690403086));
#56263=CARTESIAN_POINT('Ctrl Pts',(0.413914308982594,-0.674255827328862,
-0.277141813834746));
#56264=CARTESIAN_POINT('Ctrl Pts',(0.30204458889474,-0.742930768882917,
-0.282424937266406));
#56265=CARTESIAN_POINT('Ctrl Pts',(0.172715228539141,-0.783164416923164,
-0.287708060698066));
#56266=CARTESIAN_POINT('Ctrl Pts',(0.0416298533602581,-0.790071468974327,
-0.292991184129726));
#56267=CARTESIAN_POINT('Ctrl Pts',(-0.0894555218186243,-0.79697852102549,
-0.298274307561386));
#56268=CARTESIAN_POINT('Ctrl Pts',(-0.222296911820787,-0.770558977087567,
-0.303557430993046));
#56269=CARTESIAN_POINT('Ctrl Pts',(-0.34076427114486,-0.71402078603363,
-0.308840554424706));
#56270=CARTESIAN_POINT('Ctrl Pts',(-0.459231630468936,-0.65748259497969,
-0.314123677856367));
#56271=CARTESIAN_POINT('Ctrl Pts',(-0.563324959114919,-0.570825756809734,
-0.319406801288026));
#56272=CARTESIAN_POINT('Ctrl Pts',(-0.640404887410046,-0.464572440366096,
-0.324689924719687));
#56273=CARTESIAN_POINT('Ctrl Pts',(-0.717484815705173,-0.358319123922458,
-0.329973048151347));
#56274=CARTESIAN_POINT('Ctrl Pts',(-0.767551343649444,-0.232469329205139,
-0.335256171583008));
#56275=CARTESIAN_POINT('Ctrl Pts',(-0.784525225223783,-0.102304165553495,
-0.340539295014668));
#56276=CARTESIAN_POINT('Ctrl Pts',(-0.788945628951326,-0.068406051437288,
-0.341915146401877));
#56277=CARTESIAN_POINT('Ctrl Pts',(-0.791121670013111,-0.0342152664715848,
-0.343290997789086));
#56278=CARTESIAN_POINT('Ctrl Pts',(-0.791087916566115,-2.02165423325296E-5,
-0.344666849176295));
#56279=CARTESIAN_POINT('Ctrl Pts',(-0.791102868091814,-2.02590743034978E-5,
-0.373133150823704));
#56280=CARTESIAN_POINT('Ctrl Pts',(-0.791132983132153,-0.0293999621887177,
-0.371950982545555));
#56281=CARTESIAN_POINT('Ctrl Pts',(-0.789527747106607,-0.0587763927716652,
-0.370768814267405));
#56282=CARTESIAN_POINT('Ctrl Pts',(-0.786261896246886,-0.087967033655985,
-0.369586645989256));
#56283=CARTESIAN_POINT('Ctrl Pts',(-0.771666771745399,-0.218420338563246,
-0.364303522557596));
#56284=CARTESIAN_POINT('Ctrl Pts',(-0.723905744339962,-0.345163040037108,
-0.359020399125935));
#56285=CARTESIAN_POINT('Ctrl Pts',(-0.648778120355349,-0.452805608440245,
-0.353737275694275));
#56286=CARTESIAN_POINT('Ctrl Pts',(-0.573650496370737,-0.560448176843381,
-0.348454152262615));
#56287=CARTESIAN_POINT('Ctrl Pts',(-0.471156275806947,-0.648990612175792,
-0.343171028830956));
#56288=CARTESIAN_POINT('Ctrl Pts',(-0.35374065524607,-0.707681791005683,
-0.337887905399295));
#56289=CARTESIAN_POINT('Ctrl Pts',(-0.23632503468519,-0.766372969835576,
-0.332604781967635));
#56290=CARTESIAN_POINT('Ctrl Pts',(-0.103988014127221,-0.795212892162948,
-0.327321658535975));
#56291=CARTESIAN_POINT('Ctrl Pts',(0.0272015954388539,-0.790699716531558,
-0.322038535104315));
#56292=CARTESIAN_POINT('Ctrl Pts',(0.158391205004929,-0.786186540900168,
-0.316755411672654));
#56293=CARTESIAN_POINT('Ctrl Pts',(0.288433403579109,-0.748320267310017,
-0.311472288240994));
#56294=CARTESIAN_POINT('Ctrl Pts',(0.401538025636569,-0.68169874752446,
-0.306189164809334));
#56295=CARTESIAN_POINT('Ctrl Pts',(0.514642647694025,-0.615077227738905,
-0.300906041377674));
#56296=CARTESIAN_POINT('Ctrl Pts',(0.610809693234762,-0.519700461757946,
-0.295622917946014));
#56297=CARTESIAN_POINT('Ctrl Pts',(0.678362232218607,-0.407149420478866,
-0.290339794514354));
#56298=CARTESIAN_POINT('Ctrl Pts',(0.745914771202452,-0.294598379199785,
-0.285056671082694));
#56299=CARTESIAN_POINT('Ctrl Pts',(0.784852803629405,-0.164873062622582,
-0.279773547651034));
#56300=CARTESIAN_POINT('Ctrl Pts',(0.790448342209017,-0.0337251600679334,
-0.274490424219374));
#56301=CARTESIAN_POINT('Ctrl Pts',(0.796043880788629,0.0974227424867189,
-0.269207300787713));
#56302=CARTESIAN_POINT('Ctrl Pts',(0.768296925520898,0.229993231018817,
-0.263924177356053));
#56303=CARTESIAN_POINT('Ctrl Pts',(0.710576604148165,0.34788914704293,-0.258641053924393));
#56304=CARTESIAN_POINT('Ctrl Pts',(0.652856282775432,0.465785063067044,
-0.253357930492733));
#56305=CARTESIAN_POINT('Ctrl Pts',(0.565162595297698,0.569006406583174,
-0.248074807061072));
#56306=CARTESIAN_POINT('Ctrl Pts',(0.458143611008586,0.645019689538202,
-0.242791683629412));
#56307=CARTESIAN_POINT('Ctrl Pts',(0.351124626719476,0.721032972493228,
-0.237508560197752));
#56308=CARTESIAN_POINT('Ctrl Pts',(0.22478034561899,0.769838194887155,-0.232225436766092));
#56309=CARTESIAN_POINT('Ctrl Pts',(0.0944519125651878,0.785509263983989,
-0.226942313334432));
#56310=CARTESIAN_POINT('Ctrl Pts',(-0.0358765204886145,0.801180333080823,
-0.221659189902772));
#56311=CARTESIAN_POINT('Ctrl Pts',(-0.170189105495733,0.783717248880564,
-0.216376066471112));
#56312=CARTESIAN_POINT('Ctrl Pts',(-0.292177137732413,0.735240432042466,
-0.211092943039452));
#56313=CARTESIAN_POINT('Ctrl Pts',(-0.414165169969093,0.686763615204368,
-0.205809819607792));
#56314=CARTESIAN_POINT('Ctrl Pts',(-0.523828649435335,0.60727306572843,
-0.200526696176131));
#56315=CARTESIAN_POINT('Ctrl Pts',(-0.607851891327949,0.506420808823632,
-0.195243572744471));
#56316=CARTESIAN_POINT('Ctrl Pts',(-0.69187513322056,0.405568551918837,
-0.189960449312812));
#56317=CARTESIAN_POINT('Ctrl Pts',(-0.750258137539544,0.283354587585183,
-0.184677325881152));
#56318=CARTESIAN_POINT('Ctrl Pts',(-0.775911787358977,0.15461852632206,
-0.179394202449492));
#56319=CARTESIAN_POINT('Ctrl Pts',(-0.786045869844276,0.103763311845536,
-0.177307185240896));
#56320=CARTESIAN_POINT('Ctrl Pts',(-0.791072456914615,0.0518903082719592,
-0.1752201680323));
#56321=CARTESIAN_POINT('Ctrl Pts',(-0.791044518748003,1.1964098827608E-5,
-0.173133150823703));
#56322=CARTESIAN_POINT('Origin',(0.,0.,-4.178617978381));
#56323=CARTESIAN_POINT('',(-0.676660923651515,1.32068574775878E-5,-0.0786179783809996));
#56324=CARTESIAN_POINT('',(-0.6767,-8.45931892044317E-14,-0.0711000000000004));
#56325=CARTESIAN_POINT('',(-0.6767,-8.45931892044317E-14,-4.178617978381));
#56326=CARTESIAN_POINT('',(-0.657933019064465,-0.158364055658306,-0.0711000000000004));
#56327=CARTESIAN_POINT('Ctrl Pts',(-0.676660923651515,1.32068574776288E-5,
-0.0786179783809996));
#56328=CARTESIAN_POINT('Ctrl Pts',(-0.676624313627597,-0.0532698217775889,
-0.0761119855873332));
#56329=CARTESIAN_POINT('Ctrl Pts',(-0.670346619805526,-0.106561407057785,
-0.0736059927936668));
#56330=CARTESIAN_POINT('Ctrl Pts',(-0.657933019064465,-0.158364055658306,
-0.0711000000000003));
#56331=CARTESIAN_POINT('Origin',(0.,0.,-0.0711000000000004));
#56332=CARTESIAN_POINT('Origin',(0.,0.,-4.178617978381));
#56333=CARTESIAN_POINT('',(-0.676689663936658,-1.72930529912188E-5,-0.278617978381001));
#56334=CARTESIAN_POINT('',(-0.676652541823756,1.02339851014988E-5,-0.239182021618994));
#56335=CARTESIAN_POINT('',(-0.6767,-8.45931892044317E-14,-4.178617978381));
#56336=CARTESIAN_POINT('Ctrl Pts',(-0.676689663936658,-1.72930529912067E-5,
-0.278617978381001));
#56337=CARTESIAN_POINT('Ctrl Pts',(-0.676718536339111,-0.029267438783139,
-0.277242126993792));
#56338=CARTESIAN_POINT('Ctrl Pts',(-0.667709720174263,-0.170817385471675,
-0.270583152174923));
#56339=CARTESIAN_POINT('Ctrl Pts',(-0.570903748360253,-0.414153845586582,
-0.258641053924393));
#56340=CARTESIAN_POINT('Ctrl Pts',(-0.303782187894811,-0.636530343082252,
-0.242791683629414));
#56341=CARTESIAN_POINT('Ctrl Pts',(0.0371118910375575,-0.704327481431854,
-0.226942313334432));
#56342=CARTESIAN_POINT('Ctrl Pts',(0.36899349191975,-0.601080952691479,
-0.211092943039453));
#56343=CARTESIAN_POINT('Ctrl Pts',(0.611266154089886,-0.351863826144559,
-0.195243572744473));
#56344=CARTESIAN_POINT('Ctrl Pts',(0.705094887117879,-0.0171977214955263,
-0.179394202449492));
#56345=CARTESIAN_POINT('Ctrl Pts',(0.627693390094468,0.321644844638033,
-0.163544832154511));
#56346=CARTESIAN_POINT('Ctrl Pts',(0.39785894362146,0.58237689240233,-0.147695461859531));
#56347=CARTESIAN_POINT('Ctrl Pts',(0.071404981194182,0.701680767872716,
-0.13184609156455));
#56348=CARTESIAN_POINT('Ctrl Pts',(-0.272387992417769,0.650583340742987,
-0.11599672126957));
#56349=CARTESIAN_POINT('Ctrl Pts',(-0.550035273505243,0.441494566425662,
-0.100147350974589));
#56350=CARTESIAN_POINT('Ctrl Pts',(-0.663290191377602,0.192838810536258,
-0.0876877700117325));
#56351=CARTESIAN_POINT('Ctrl Pts',(-0.676688583350635,0.0402697372418875,
-0.0805113124805359));
#56352=CARTESIAN_POINT('Ctrl Pts',(-0.676660923651515,1.32068574776288E-5,
-0.0786179783809996));
#56353=CARTESIAN_POINT('',(-0.364065050236237,0.570420484551954,-0.0711000000000004));
#56354=CARTESIAN_POINT('Origin',(0.,0.,-0.0711000000000004));
#56355=CARTESIAN_POINT('Ctrl Pts',(-0.676652541823757,1.02339851015057E-5,
-0.239182021618994));
#56356=CARTESIAN_POINT('Ctrl Pts',(-0.676615943780199,-0.067948624078856,
-0.235985915395931));
#56357=CARTESIAN_POINT('Ctrl Pts',(-0.64961770844105,-0.248271044387699,
-0.227506685741207));
#56358=CARTESIAN_POINT('Ctrl Pts',(-0.491821179438923,-0.505535863107229,
-0.213744332654824));
#56359=CARTESIAN_POINT('Ctrl Pts',(-0.190657404081973,-0.679046628726581,
-0.197894962359843));
#56360=CARTESIAN_POINT('Ctrl Pts',(0.156805532386105,-0.687652471031271,
-0.182045592064863));
#56361=CARTESIAN_POINT('Ctrl Pts',(0.466191447257558,-0.529265333633324,
-0.166196221769883));
#56362=CARTESIAN_POINT('Ctrl Pts',(0.662358975760562,-0.242345413653074,
-0.150346851474902));
#56363=CARTESIAN_POINT('Ctrl Pts',(0.697685099148249,0.103422631371823,
-0.134497481179922));
#56364=CARTESIAN_POINT('Ctrl Pts',(0.563560339571208,0.424084008064863,
-0.118648110884941));
#56365=CARTESIAN_POINT('Ctrl Pts',(0.292616745553076,0.64173975329643,-0.102798740589961));
#56366=CARTESIAN_POINT('Ctrl Pts',(-0.0494690429576347,0.703588850062655,
-0.0869493702949807));
#56367=CARTESIAN_POINT('Ctrl Pts',(-0.269389956604521,0.630845896423734,
-0.0763831234316606));
#56368=CARTESIAN_POINT('Ctrl Pts',(-0.364065050236245,0.570420484551949,
-0.0711000000000004));
#56369=CARTESIAN_POINT('Origin',(0.,0.,-4.178617978381));
#56370=CARTESIAN_POINT('',(-0.676737173032778,1.25957128338008E-5,-0.478617978381));
#56371=CARTESIAN_POINT('',(-0.676702453340578,-1.73294345428565E-5,-0.439182021618994));
#56372=CARTESIAN_POINT('',(-0.6767,-8.45931892044317E-14,-4.178617978381));
#56373=CARTESIAN_POINT('Ctrl Pts',(-0.676737173032778,1.25957128337788E-5,
-0.478617978381));
#56374=CARTESIAN_POINT('Ctrl Pts',(-0.676652639569119,-0.0987193633761514,
-0.473972941507046));
#56375=CARTESIAN_POINT('Ctrl Pts',(-0.629917600928146,-0.30982344429185,
-0.464044781201433));
#56376=CARTESIAN_POINT('Ctrl Pts',(-0.41842147815042,-0.567783376690792,
-0.448833497464158));
#56377=CARTESIAN_POINT('Ctrl Pts',(-0.0964411493212378,-0.698679898767291,
-0.432984127169178));
#56378=CARTESIAN_POINT('Ctrl Pts',(0.248959603828383,-0.659904244480755,
-0.417134756874197));
#56379=CARTESIAN_POINT('Ctrl Pts',(0.533901314322515,-0.4608729573248,-0.401285386579217));
#56380=CARTESIAN_POINT('Ctrl Pts',(0.689186800078316,-0.149920148114908,
-0.385436016284236));
#56381=CARTESIAN_POINT('Ctrl Pts',(0.677105478124627,0.197440289037993,
-0.369586645989256));
#56382=CARTESIAN_POINT('Ctrl Pts',(0.50059125872345,0.496852984183748,-0.353737275694276));
#56383=CARTESIAN_POINT('Ctrl Pts',(0.202510055068408,0.675606522928187,
-0.337887905399296));
#56384=CARTESIAN_POINT('Ctrl Pts',(-0.144750067291325,0.690291180816235,
-0.322038535104314));
#56385=CARTESIAN_POINT('Ctrl Pts',(-0.456858098816181,0.537340835519866,
-0.306189164809335));
#56386=CARTESIAN_POINT('Ctrl Pts',(-0.640557186228658,0.278503995431137,
-0.291715645901563));
#56387=CARTESIAN_POINT('Ctrl Pts',(-0.676607669375318,0.0830500191364299,
-0.282525250425452));
#56388=CARTESIAN_POINT('Ctrl Pts',(-0.676689663936658,-1.72930529912067E-5,
-0.278617978381001));
#56389=CARTESIAN_POINT('Ctrl Pts',(-0.676702453340578,-1.73294345428357E-5,
-0.439182021618993));
#56390=CARTESIAN_POINT('Ctrl Pts',(-0.676728213481893,-0.0251484697423405,
-0.437999853340846));
#56391=CARTESIAN_POINT('Ctrl Pts',(-0.669218687692859,-0.162575651503364,
-0.431534561631038));
#56392=CARTESIAN_POINT('Ctrl Pts',(-0.57836825932194,-0.40366403145049,
-0.419786146489569));
#56393=CARTESIAN_POINT('Ctrl Pts',(-0.315350287932037,-0.63087929875971,
-0.403936776194589));
#56394=CARTESIAN_POINT('Ctrl Pts',(0.0242494914065197,-0.704887548433319,
-0.388087405899608));
#56395=CARTESIAN_POINT('Ctrl Pts',(0.357960358964906,-0.607716113702729,
-0.372238035604628));
#56396=CARTESIAN_POINT('Ctrl Pts',(0.604741700327879,-0.362962766947641,
-0.356388665309647));
#56397=CARTESIAN_POINT('Ctrl Pts',(0.704663454379142,-0.030065073630256,
-0.340539295014667));
#56398=CARTESIAN_POINT('Ctrl Pts',(0.633459948009497,0.310133825079147,
-0.324689924719686));
#56399=CARTESIAN_POINT('Ctrl Pts',(0.408422715107778,0.575017720253068,
-0.308840554424706));
#56400=CARTESIAN_POINT('Ctrl Pts',(0.0842013460493761,0.700260397514991,
-0.292991184129726));
#56401=CARTESIAN_POINT('Ctrl Pts',(-0.260468074786106,0.655447090429983,
-0.277141813834745));
#56402=CARTESIAN_POINT('Ctrl Pts',(-0.541883609692458,0.451460534380044,
-0.261292443539765));
#56403=CARTESIAN_POINT('Ctrl Pts',(-0.661492385626837,0.201081800936145,
-0.248639179467848));
#56404=CARTESIAN_POINT('Ctrl Pts',(-0.676676439886391,0.0443865144831086,
-0.241269038827591));
#56405=CARTESIAN_POINT('Ctrl Pts',(-0.676652541823757,1.02339851015057E-5,
-0.239182021618994));
#56406=CARTESIAN_POINT('Origin',(0.,0.,-4.178617978381));
#56407=CARTESIAN_POINT('',(-0.676642536276524,-2.06014658737574E-7,-0.678617978381));
#56408=CARTESIAN_POINT('',(-0.676725589147528,1.50742954787217E-5,-0.639182021618993));
#56409=CARTESIAN_POINT('',(-0.6767,-8.45931892044317E-14,-4.178617978381));
#56410=CARTESIAN_POINT('Ctrl Pts',(-0.676642536276524,-2.06014658693521E-7,
-0.678617978381));
#56411=CARTESIAN_POINT('Ctrl Pts',(-0.676643131183487,-0.0559476708465134,
-0.675986879451961));
#56412=CARTESIAN_POINT('Ctrl Pts',(-0.656004364269065,-0.224234593763904,
-0.668072657091263));
#56413=CARTESIAN_POINT('Ctrl Pts',(-0.518031279492488,-0.478641922203943,
-0.654875311298903));
#56414=CARTESIAN_POINT('Ctrl Pts',(-0.226530078974616,-0.667936089415343,
-0.639025941003923));
#56415=CARTESIAN_POINT('Ctrl Pts',(0.119983225911628,-0.695024115929475,
-0.623176570708943));
#56416=CARTESIAN_POINT('Ctrl Pts',(0.437358988551026,-0.553327761238609,
-0.607327200413961));
#56417=CARTESIAN_POINT('Ctrl Pts',(0.648523521169567,-0.277257531391908,
-0.591477830118983));
#56418=CARTESIAN_POINT('Ctrl Pts',(0.702196193133595,0.0661438022220719,
-0.575628459824));
#56419=CARTESIAN_POINT('Ctrl Pts',(0.585342767907381,0.393482325247575,
-0.559779089529022));
#56420=CARTESIAN_POINT('Ctrl Pts',(0.326340725662382,0.625264925449887,
-0.54392971923404));
#56421=CARTESIAN_POINT('Ctrl Pts',(-0.011912116922439,0.705203940498158,
-0.528080348939061));
#56422=CARTESIAN_POINT('Ctrl Pts',(-0.347272140053286,0.613886436539002,
-0.51223097864408));
#56423=CARTESIAN_POINT('Ctrl Pts',(-0.59829823587811,0.373488577025802,
-0.496381608349099));
#56424=CARTESIAN_POINT('Ctrl Pts',(-0.67304244002644,0.139426503702999,
-0.485177274928072));
#56425=CARTESIAN_POINT('Ctrl Pts',(-0.676748785355414,0.013575359070847,
-0.479256064938706));
#56426=CARTESIAN_POINT('Ctrl Pts',(-0.676737173032778,1.25957128337788E-5,
-0.478617978381));
#56427=CARTESIAN_POINT('Ctrl Pts',(-0.676725589147528,1.50742954787165E-5,
-0.639182021618993));
#56428=CARTESIAN_POINT('Ctrl Pts',(-0.676633999892269,-0.0946047616401611,
-0.6347306678541));
#56429=CARTESIAN_POINT('Ctrl Pts',(-0.632835371378299,-0.30160699551933,
-0.624996190657547));
#56430=CARTESIAN_POINT('Ctrl Pts',(-0.42871562406298,-0.560051254246869,
-0.609978590029332));
#56431=CARTESIAN_POINT('Ctrl Pts',(-0.109178218030051,-0.69680313604847,
-0.594129219734354));
#56432=CARTESIAN_POINT('Ctrl Pts',(0.236872768681544,-0.664338607305327,
-0.578279849439372));
#56433=CARTESIAN_POINT('Ctrl Pts',(0.525399961944826,-0.470541574876744,
-0.562430479144392));
#56434=CARTESIAN_POINT('Ctrl Pts',(0.686335456690993,-0.162475027583201,
-0.546581108849412));
#56435=CARTESIAN_POINT('Ctrl Pts',(0.680596583308102,0.185048059941882,
-0.530731738554432));
#56436=CARTESIAN_POINT('Ctrl Pts',(0.509577008823849,0.487632818601885,
-0.514882368259451));
#56437=CARTESIAN_POINT('Ctrl Pts',(0.214808289323237,0.67179750858231,-0.499032997964472));
#56438=CARTESIAN_POINT('Ctrl Pts',(-0.132125935456141,0.692818324582584,
-0.48318362766949));
#56439=CARTESIAN_POINT('Ctrl Pts',(-0.446973799862388,0.545590428747379,
-0.46733425737451));
#56440=CARTESIAN_POINT('Ctrl Pts',(-0.637887935546393,0.286731526864918,
-0.452667055357677));
#56441=CARTESIAN_POINT('Ctrl Pts',(-0.676613091118437,0.0871628810853665,
-0.443282976772505));
#56442=CARTESIAN_POINT('Ctrl Pts',(-0.676702453340578,-1.73294345428357E-5,
-0.439182021618993));
#56443=CARTESIAN_POINT('Origin',(0.,0.,-4.178617978381));
#56444=CARTESIAN_POINT('',(-0.676738329529131,-1.22799319098172E-5,-0.878617978381001));
#56445=CARTESIAN_POINT('',(-0.676643916272068,-3.98541505916561E-6,-0.839182021618994));
#56446=CARTESIAN_POINT('',(-0.6767,-8.45931892044317E-14,-4.178617978381));
#56447=CARTESIAN_POINT('Ctrl Pts',(-0.676738329529131,-1.22799319097634E-5,
-0.878617978381001));
#56448=CARTESIAN_POINT('Ctrl Pts',(-0.676749353176149,-0.013130197661408,
-0.878000817396877));
#56449=CARTESIAN_POINT('Ctrl Pts',(-0.673177374051864,-0.138536282933656,
-0.872100532981092));
#56450=CARTESIAN_POINT('Ctrl Pts',(-0.599033661857993,-0.372307894335739,
-0.860917125133648));
#56451=CARTESIAN_POINT('Ctrl Pts',(-0.348482163889545,-0.613200356877398,
-0.845067754838668));
#56452=CARTESIAN_POINT('Ctrl Pts',(-0.0133028882008698,-0.705179076114163,
-0.829218384543688));
#56453=CARTESIAN_POINT('Ctrl Pts',(0.325106951293811,-0.625907314579525,
-0.813369014248707));
#56454=CARTESIAN_POINT('Ctrl Pts',(0.584565608603702,-0.394635965747537,
-0.797519643953726));
#56455=CARTESIAN_POINT('Ctrl Pts',(0.702064379543393,-0.067528536190703,
-0.781670273658747));
#56456=CARTESIAN_POINT('Ctrl Pts',(0.64906906380117,0.275977982165213,-0.765820903363766));
#56457=CARTESIAN_POINT('Ctrl Pts',(0.438449404123081,0.552464131186653,
-0.749971533068786));
#56458=CARTESIAN_POINT('Ctrl Pts',(0.121353710493789,0.694786134845175,
-0.734122162773805));
#56459=CARTESIAN_POINT('Ctrl Pts',(-0.225212343175068,0.66838155024305,
-0.718272792478825));
#56460=CARTESIAN_POINT('Ctrl Pts',(-0.517086300395306,0.479662646207939,
-0.702423422183845));
#56461=CARTESIAN_POINT('Ctrl Pts',(-0.655780419625378,0.225124967968464,
-0.689205150817903));
#56462=CARTESIAN_POINT('Ctrl Pts',(-0.676641936638166,0.056392218441925,
-0.681270002883622));
#56463=CARTESIAN_POINT('Ctrl Pts',(-0.676642536276524,-2.06014658693521E-7,
-0.678617978381));
#56464=CARTESIAN_POINT('Ctrl Pts',(-0.676643916272068,-3.98541505918296E-6,
-0.839182021618994));
#56465=CARTESIAN_POINT('Ctrl Pts',(-0.676654604183955,-0.0518326861038898,
-0.836744605799016));
#56466=CARTESIAN_POINT('Ctrl Pts',(-0.658031674012512,-0.215993061705228,
-0.829024066547377));
#56467=CARTESIAN_POINT('Ctrl Pts',(-0.526681713994867,-0.469106454701526,
-0.816020403864078));
#56468=CARTESIAN_POINT('Ctrl Pts',(-0.23868430153437,-0.66368991095259,
-0.800171033569099));
#56469=CARTESIAN_POINT('Ctrl Pts',(0.107276829327393,-0.697098397350523,
-0.784321663274117));
#56470=CARTESIAN_POINT('Ctrl Pts',(0.427186125669077,-0.561218769941854,
-0.768472292979137));
#56471=CARTESIAN_POINT('Ctrl Pts',(0.643354639169021,-0.289048961179428,
-0.752622922684157));
#56472=CARTESIAN_POINT('Ctrl Pts',(0.703286538458407,0.0533154623200356,
-0.736773552389177));
#56473=CARTESIAN_POINT('Ctrl Pts',(0.592427553686509,0.38273239650208,-0.720924182094196));
#56474=CARTESIAN_POINT('Ctrl Pts',(0.337699434353656,0.619203993637335,
-0.705074811799215));
#56475=CARTESIAN_POINT('Ctrl Pts',(0.00096208864391743,0.705303883503167,
-0.689225441504236));
#56476=CARTESIAN_POINT('Ctrl Pts',(-0.336008897212553,0.620122983522791,
-0.673376071209255));
#56477=CARTESIAN_POINT('Ctrl Pts',(-0.591381198224044,0.384347202521759,
-0.657526700914275));
#56478=CARTESIAN_POINT('Ctrl Pts',(-0.671751029522471,0.14766660228095,
-0.646128684384187));
#56479=CARTESIAN_POINT('Ctrl Pts',(-0.676742703303884,0.0176955179453271,
-0.64001379128576));
#56480=CARTESIAN_POINT('Ctrl Pts',(-0.676725589147528,1.50742954787165E-5,
-0.639182021618993));
#56481=CARTESIAN_POINT('Origin',(0.,0.,-4.178617978381));
#56482=CARTESIAN_POINT('',(-0.676688317179324,1.72353111514132E-5,-1.078617978381));
#56483=CARTESIAN_POINT('',(-0.676747836763073,-8.96412734507912E-6,-1.03918202161899));
#56484=CARTESIAN_POINT('',(-0.6767,-8.45931892044317E-14,-4.178617978381));
#56485=CARTESIAN_POINT('Ctrl Pts',(-0.676688317179324,1.72353111514319E-5,
-1.078617978381));
#56486=CARTESIAN_POINT('Ctrl Pts',(-0.676607315101875,-0.0826056787905753,
-1.07473163191013));
#56487=CARTESIAN_POINT('Ctrl Pts',(-0.640840351711829,-0.277614899869378,
-1.0655621620076));
#56488=CARTESIAN_POINT('Ctrl Pts',(-0.45791694746335,-0.536438780709928,
-1.05110956867341));
#56489=CARTESIAN_POINT('Ctrl Pts',(-0.146111169363581,-0.69000436405208,
-1.03526019837843));
#56490=CARTESIAN_POINT('Ctrl Pts',(0.201177238393133,-0.676004596860274,
-1.01941082808345));
#56491=CARTESIAN_POINT('Ctrl Pts',(0.49961039794122,-0.497839277772177,
-1.00356145778847));
#56492=CARTESIAN_POINT('Ctrl Pts',(0.676714772016422,-0.198775284073422,
-0.987712087493491));
#56493=CARTESIAN_POINT('Ctrl Pts',(0.689481130432523,0.148560650918064,
-0.971862717198511));
#56494=CARTESIAN_POINT('Ctrl Pts',(0.53480920392387,0.459819107499921,-0.956013346903531));
#56495=CARTESIAN_POINT('Ctrl Pts',(0.250260574610009,0.659411966087648,
-0.94016397660855));
#56496=CARTESIAN_POINT('Ctrl Pts',(-0.0950630339562937,0.698868740035448,
-0.92431460631357));
#56497=CARTESIAN_POINT('Ctrl Pts',(-0.417300889101903,0.568607478123943,
-0.908465236018589));
#56498=CARTESIAN_POINT('Ctrl Pts',(-0.629596992258038,0.31071086642954,
-0.893233026707733));
#56499=CARTESIAN_POINT('Ctrl Pts',(-0.676654986731472,0.0991639691995475,
-0.883283940828537));
#56500=CARTESIAN_POINT('Ctrl Pts',(-0.676738329529131,-1.22799319097634E-5,
-0.878617978381001));
#56501=CARTESIAN_POINT('Ctrl Pts',(-0.676747836763073,-8.96412734503922E-6,
-1.03918202161899));
#56502=CARTESIAN_POINT('Ctrl Pts',(-0.676753746890542,-0.0090097302053093,
-1.03875854374393));
#56503=CARTESIAN_POINT('Ctrl Pts',(-0.674383982793645,-0.130296973834658,
-1.03305194243721));
#56504=CARTESIAN_POINT('Ctrl Pts',(-0.605729665760521,-0.361311590897459,
-1.02206221769882));
#56505=CARTESIAN_POINT('Ctrl Pts',(-0.359616966834596,-0.606737283232118,
-1.00621284740384));
#56506=CARTESIAN_POINT('Ctrl Pts',(-0.0261724389449761,-0.704818769002982,
-0.990363477108863));
#56507=CARTESIAN_POINT('Ctrl Pts',(0.313627981942751,-0.631737273430753,
-0.974514106813883));
#56508=CARTESIAN_POINT('Ctrl Pts',(0.5772648515989,-0.405240403720689,-0.958664736518902));
#56509=CARTESIAN_POINT('Ctrl Pts',(0.700714800347687,-0.0803321994775939,
-0.942815366223922));
#56510=CARTESIAN_POINT('Ctrl Pts',(0.653998403401114,0.264084422198656,
-0.926965995928941));
#56511=CARTESIAN_POINT('Ctrl Pts',(0.44846058817974,0.544368987497165,-0.911116625633962));
#56512=CARTESIAN_POINT('Ctrl Pts',(0.134015555013097,0.692455287158485,
-0.89526725533898));
#56513=CARTESIAN_POINT('Ctrl Pts',(-0.212974726593566,0.672381037456889,
-0.879417885044001));
#56514=CARTESIAN_POINT('Ctrl Pts',(-0.508244777755666,0.489021205658097,
-0.86356851474902));
#56515=CARTESIAN_POINT('Ctrl Pts',(-0.653661894356427,0.233365601831161,
-0.850156560274017));
#56516=CARTESIAN_POINT('Ctrl Pts',(-0.676631438026886,0.0605065466184489,
-0.842027729230676));
#56517=CARTESIAN_POINT('Ctrl Pts',(-0.676643916272068,-3.98541505918296E-6,
-0.839182021618994));
#56518=CARTESIAN_POINT('Origin',(0.,0.,-4.178617978381));
#56519=CARTESIAN_POINT('',(-0.676661399215972,-1.33519825231872E-5,-1.278617978381));
#56520=CARTESIAN_POINT('',(-0.676676376008853,1.62256556966722E-5,-1.23918202161899));
#56521=CARTESIAN_POINT('',(-0.6767,-8.45931892044317E-14,-4.178617978381));
#56522=CARTESIAN_POINT('Ctrl Pts',(-0.676661399215972,-1.3351982523134E-5,
-1.278617978381));
#56523=CARTESIAN_POINT('Ctrl Pts',(-0.676689839809335,-0.0398249105762218,
-1.27674556985505));
#56524=CARTESIAN_POINT('Ctrl Pts',(-0.663481583410436,-0.191948734974615,
-1.26959003789743));
#56525=CARTESIAN_POINT('Ctrl Pts',(-0.550903588163435,-0.440408597523208,
-1.25715138250816));
#56526=CARTESIAN_POINT('Ctrl Pts',(-0.273671211948421,-0.650045047650077,
-1.24130201221318));
#56527=CARTESIAN_POINT('Ctrl Pts',(0.0700213418398019,-0.70182013928831,
-1.2254526419182));
#56528=CARTESIAN_POINT('Ctrl Pts',(0.396709436958603,-0.583160457208559,
-1.20960327162322));
#56529=CARTESIAN_POINT('Ctrl Pts',(0.627057915507849,-0.322882125275867,
-1.19375390132824));
#56530=CARTESIAN_POINT('Ctrl Pts',(0.705127387008331,0.0158070969666729,
-1.17790453103325));
#56531=CARTESIAN_POINT('Ctrl Pts',(0.611958930271261,0.35065761632248,-1.16205516073828));
#56532=CARTESIAN_POINT('Ctrl Pts',(0.37017820670576,0.600352056300146,-1.14620579044329));
#56533=CARTESIAN_POINT('Ctrl Pts',(0.0385008908891459,0.704252921630042,
-1.13035642014832));
#56534=CARTESIAN_POINT('Ctrl Pts',(-0.302526243006624,0.637128219839621,
-1.11450704985333));
#56535=CARTESIAN_POINT('Ctrl Pts',(-0.570085847425583,0.41527896983686,
-1.09865767955835));
#56536=CARTESIAN_POINT('Ctrl Pts',(-0.667542007044258,0.171707850430491,
-1.08669465573424));
#56537=CARTESIAN_POINT('Ctrl Pts',(-0.676717429827001,0.0297124217068367,
-1.08001475534179));
#56538=CARTESIAN_POINT('Ctrl Pts',(-0.676688317179324,1.72353111514319E-5,
-1.078617978381));
#56539=CARTESIAN_POINT('Ctrl Pts',(-0.676676376008853,1.62256556967139E-5,
-1.23918202161899));
#56540=CARTESIAN_POINT('Ctrl Pts',(-0.676605980702497,-0.0784930040488071,
-1.23548935825719));
#56541=CARTESIAN_POINT('Ctrl Pts',(-0.643413256117644,-0.269384004288173,
-1.22651357146372));
#56542=CARTESIAN_POINT('Ctrl Pts',(-0.467632374358977,-0.527990962186469,
-1.21225466123859));
#56543=CARTESIAN_POINT('Ctrl Pts',(-0.158681606577905,-0.687222410456076,
-1.19640529094361));
#56544=CARTESIAN_POINT('Ctrl Pts',(0.188804481289216,-0.679564096715178,
-1.18055592064863));
#56545=CARTESIAN_POINT('Ctrl Pts',(0.490440005394944,-0.506875817935137,
-1.16470655035365));
#56546=CARTESIAN_POINT('Ctrl Pts',(0.67297374449562,-0.211094369699316,
-1.14885718005867));
#56547=CARTESIAN_POINT('Ctrl Pts',(0.692077964492487,0.135950670329878,
-1.13300780976369));
#56548=CARTESIAN_POINT('Ctrl Pts',(0.543113266727756,0.449980525360276,
-1.1171584394687));
#56549=CARTESIAN_POINT('Ctrl Pts',(0.262255251094087,0.654734050567698,
-1.10130906917373));
#56550=CARTESIAN_POINT('Ctrl Pts',(-0.0822906125712717,0.700487507941325,
-1.08545969887874));
#56551=CARTESIAN_POINT('Ctrl Pts',(-0.406852464454183,0.576129816852735,
-1.06961032858376));
#56552=CARTESIAN_POINT('Ctrl Pts',(-0.626579463050419,0.318921822910923,
-1.05418443616385));
#56553=CARTESIAN_POINT('Ctrl Pts',(-0.676680014743584,0.103279862638811,
-1.04404166717559));
#56554=CARTESIAN_POINT('Ctrl Pts',(-0.676747836763073,-8.96412734503922E-6,
-1.03918202161899));
#56555=CARTESIAN_POINT('Origin',(0.,0.,-4.178617978381));
#56556=CARTESIAN_POINT('',(-0.67675648621479,3.15325649049231E-6,-1.478617978381));
#56557=CARTESIAN_POINT('',(-0.676671333621808,-1.54941563473843E-5,-1.43918202161899));
#56558=CARTESIAN_POINT('',(-0.6767,-8.45931892044317E-14,-4.178617978381));
#56559=CARTESIAN_POINT('Ctrl Pts',(-0.67675648621479,3.15325649049647E-6,
-1.478617978381));
#56560=CARTESIAN_POINT('Ctrl Pts',(-0.676727987849731,-0.109274258141125,
-1.4734763843683));
#56561=CARTESIAN_POINT('Ctrl Pts',(-0.622024114183857,-0.330864596680709,
-1.46305166692394));
#56562=CARTESIAN_POINT('Ctrl Pts',(-0.391401124376496,-0.58673644514426,
-1.44734382604792));
#56563=CARTESIAN_POINT('Ctrl Pts',(-0.0636496855493053,-0.702426660764798,
-1.43149445575294));
#56564=CARTESIAN_POINT('Ctrl Pts',(0.279558875618117,-0.647534810868762,
-1.41564508545796));
#56565=CARTESIAN_POINT('Ctrl Pts',(0.554877458941432,-0.435391205449084,
-1.39979571516298));
#56566=CARTESIAN_POINT('Ctrl Pts',(0.695445827983648,-0.117514239834355,
-1.383946344868));
#56567=CARTESIAN_POINT('Ctrl Pts',(0.667127404398765,0.228900682663626,
-1.36809697457302));
#56568=CARTESIAN_POINT('Ctrl Pts',(0.476799226683618,0.51972780727763,-1.35224760427804));
#56569=CARTESIAN_POINT('Ctrl Pts',(0.170681883398015,0.684340697973908,
-1.33639823398306));
#56570=CARTESIAN_POINT('Ctrl Pts',(-0.176885008776566,0.682763641309219,
-1.32054886368808));
#56571=CARTESIAN_POINT('Ctrl Pts',(-0.481495942925332,0.515379620445116,
-1.3046994933931));
#56572=CARTESIAN_POINT('Ctrl Pts',(-0.647004900930806,0.257397591632518,
-1.29072253162407));
#56573=CARTESIAN_POINT('Ctrl Pts',(-0.676609592810283,0.0725060124792107,
-1.28202869328671));
#56574=CARTESIAN_POINT('Ctrl Pts',(-0.676661399215972,-1.3351982523134E-5,
-1.278617978381));
#56575=CARTESIAN_POINT('Ctrl Pts',(-0.676671333621808,-1.54941563473114E-5,
-1.43918202161899));
#56576=CARTESIAN_POINT('Ctrl Pts',(-0.676701550046883,-0.0357074174336674,
-1.4375032962021));
#56577=CARTESIAN_POINT('Ctrl Pts',(-0.665192670506278,-0.183706237481266,
-1.43054144735355));
#56578=CARTESIAN_POINT('Ctrl Pts',(-0.558850665837655,-0.430279475448245,
-1.41829647507333));
#56579=CARTESIAN_POINT('Ctrl Pts',(-0.285491011948519,-0.64494137392155,
-1.40244710477835));
#56580=CARTESIAN_POINT('Ctrl Pts',(0.0571992200988665,-0.7029813247301,
-1.38659773448337));
#56581=CARTESIAN_POINT('Ctrl Pts',(0.385998804687375,-0.590304511654048,
-1.37074836418839));
#56582=CARTESIAN_POINT('Ctrl Pts',(0.62105981545978,-0.334274137977006,
-1.35489899389341));
#56583=CARTESIAN_POINT('Ctrl Pts',(0.705298438575201,0.00293363981907094,
-1.33904962359843));
#56584=CARTESIAN_POINT('Ctrl Pts',(0.618257594127741,0.339428992578101,
-1.32320025330345));
#56585=CARTESIAN_POINT('Ctrl Pts',(0.381074872501545,0.593495101283185,
-1.30735088300847));
#56586=CARTESIAN_POINT('Ctrl Pts',(0.0513493382249849,0.703432824911564,
-1.29150151271349));
#56587=CARTESIAN_POINT('Ctrl Pts',(-0.290846218427701,0.642544139281894,
-1.27565214241851));
#56588=CARTESIAN_POINT('Ctrl Pts',(-0.562410702175123,0.425615666744179,
-1.25980277212353));
#56589=CARTESIAN_POINT('Ctrl Pts',(-0.66594612195667,0.179950018736301,
-1.24764606519036));
#56590=CARTESIAN_POINT('Ctrl Pts',(-0.676706695838444,0.0338307878633588,
-1.24077248168885));
#56591=CARTESIAN_POINT('Ctrl Pts',(-0.676676376008853,1.62256556967139E-5,
-1.23918202161899));
#56592=CARTESIAN_POINT('Origin',(0.,0.,-4.178617978381));
#56593=CARTESIAN_POINT('',(-0.676650274159548,9.11169281612442E-6,-1.678617978381));
#56594=CARTESIAN_POINT('',(-0.6767513059161,7.24714397432741E-6,-1.63918202161899));
#56595=CARTESIAN_POINT('',(-0.6767,-8.45931892044317E-14,-4.178617978381));
#56596=CARTESIAN_POINT('Ctrl Pts',(-0.676650274159548,9.11169281613E-6,
-1.678617978381));
#56597=CARTESIAN_POINT('Ctrl Pts',(-0.676618550586515,-0.0664949256843561,
-1.67549032231322));
#56598=CARTESIAN_POINT('Ctrl Pts',(-0.650429330989842,-0.245359622697372,
-1.66707954281377));
#56599=CARTESIAN_POINT('Ctrl Pts',(-0.495072108323442,-0.502352569202039,
-1.65338563988267));
#56600=CARTESIAN_POINT('Ctrl Pts',(-0.195034448742293,-0.677802375348079,
-1.63753626958769));
#56601=CARTESIAN_POINT('Ctrl Pts',(0.152366702248935,-0.688650044848245,
-1.62168689929271));
#56602=CARTESIAN_POINT('Ctrl Pts',(0.462766087451164,-0.532261255896812,
-1.60583752899773));
#56603=CARTESIAN_POINT('Ctrl Pts',(0.660784210013829,-0.246614525160438,
-1.58998815870274));
#56604=CARTESIAN_POINT('Ctrl Pts',(0.698333002892782,0.0989217533935704,
-1.57413878840777));
#56605=CARTESIAN_POINT('Ctrl Pts',(0.566293861962189,0.420435200866502,
-1.55828941811278));
#56606=CARTESIAN_POINT('Ctrl Pts',(0.296732069830279,0.639847305970687,
-1.54244004781781));
#56607=CARTESIAN_POINT('Ctrl Pts',(-0.0448901553745235,0.703874541501651,
-1.52659067752282));
#56608=CARTESIAN_POINT('Ctrl Pts',(-0.37561095007723,0.596968098314967,
-1.51074130722784));
#56609=CARTESIAN_POINT('Ctrl Pts',(-0.615115828195774,0.345089863842356,
-1.49489193693286));
#56610=CARTESIAN_POINT('Ctrl Pts',(-0.67600460121947,0.118304202037452,
-1.48418416065058));
#56611=CARTESIAN_POINT('Ctrl Pts',(-0.67675727067133,0.00301116371053214,
-1.47875950779996));
#56612=CARTESIAN_POINT('Ctrl Pts',(-0.67675648621479,3.15325649049647E-6,
-1.478617978381));
#56613=CARTESIAN_POINT('Ctrl Pts',(-0.6767513059161,7.24714397433088E-6,
-1.63918202161899));
#56614=CARTESIAN_POINT('Ctrl Pts',(-0.676693498218469,-0.105156040632668,
-1.63423411071536));
#56615=CARTESIAN_POINT('Ctrl Pts',(-0.625174216556339,-0.322661917470327,
-1.62400307638006));
#56616=CARTESIAN_POINT('Ctrl Pts',(-0.402045725983278,-0.579494372636858,
-1.6084889186131));
#56617=CARTESIAN_POINT('Ctrl Pts',(-0.0764606078631723,-0.701147822605475,
-1.59263954831812));
#56618=CARTESIAN_POINT('Ctrl Pts',(0.267692724062702,-0.652529768809897,
-1.57679017802314));
#56619=CARTESIAN_POINT('Ctrl Pts',(0.54683773505632,-0.445446949947669,
-1.56094080772816));
#56620=CARTESIAN_POINT('Ctrl Pts',(0.693184952972512,-0.130188765535679,
-1.54509143743318));
#56621=CARTESIAN_POINT('Ctrl Pts',(0.671194424519117,0.216685343744462,
-1.5292420671382));
#56622=CARTESIAN_POINT('Ctrl Pts',(0.486206479121138,0.510938111085708,
-1.51339269684322));
#56623=CARTESIAN_POINT('Ctrl Pts',(0.183144847018672,0.681111194086335,
-1.49754332654823));
#56624=CARTESIAN_POINT('Ctrl Pts',(-0.16439292478377,0.685878604404777,
-1.48169395625326));
#56625=CARTESIAN_POINT('Ctrl Pts',(-0.472008401160537,0.524082591709629,
-1.46584458595827));
#56626=CARTESIAN_POINT('Ctrl Pts',(-0.644557160212723,0.265632132741012,
-1.45167394108019));
#56627=CARTESIAN_POINT('Ctrl Pts',(-0.676606455815432,0.0766187761712225,
-1.44278641963376));
#56628=CARTESIAN_POINT('Ctrl Pts',(-0.676671333621808,-1.54941563473114E-5,
-1.43918202161899));
#56629=CARTESIAN_POINT('Origin',(0.,0.,-4.178617978381));
#56630=CARTESIAN_POINT('',(-0.676707048125263,-1.71239118336567E-5,-1.878617978381));
#56631=CARTESIAN_POINT('',(-0.676645363994687,5.65701016097542E-6,-1.839182021619));
#56632=CARTESIAN_POINT('',(-0.6767,-8.45931892044317E-14,-4.178617978381));
#56633=CARTESIAN_POINT('Ctrl Pts',(-0.676707048125263,-1.71239118336441E-5,
-1.878617978381));
#56634=CARTESIAN_POINT('Ctrl Pts',(-0.676731370348907,-0.0236926529716641,
-1.87750426025813));
#56635=CARTESIAN_POINT('Ctrl Pts',(-0.669733324470885,-0.15966303113128,
-1.8711074187036));
#56636=CARTESIAN_POINT('Ctrl Pts',(-0.580960354995419,-0.399924445548537,
-1.85942745371742));
#56637=CARTESIAN_POINT('Ctrl Pts',(-0.319413674149484,-0.628831774793575,
-1.84357808342243));
#56638=CARTESIAN_POINT('Ctrl Pts',(0.0197015947556392,-0.705029320941897,
-1.82772871312745));
#56639=CARTESIAN_POINT('Ctrl Pts',(0.354032394455494,-0.610012753882915,
-1.81187934283247));
#56640=CARTESIAN_POINT('Ctrl Pts',(0.602387560713073,-0.366856542700088,
-1.79602997253749));
#56641=CARTESIAN_POINT('Ctrl Pts',(0.704454836593539,-0.0346103947345185,
-1.78018060224251));
#56642=CARTESIAN_POINT('Ctrl Pts',(0.635447510951297,0.306040776775757,
-1.76433123194753));
#56643=CARTESIAN_POINT('Ctrl Pts',(0.412123791868901,0.572370925536324,
-1.74848186165255));
#56644=CARTESIAN_POINT('Ctrl Pts',(0.0887171294811145,0.699702627664309,
-1.73263249135757));
#56645=CARTESIAN_POINT('Ctrl Pts',(-0.256234203744069,0.657113786992292,
-1.71678312106259));
#56646=CARTESIAN_POINT('Ctrl Pts',(-0.53895988100815,0.454946967115278,
-1.70093375076761));
#56647=CARTESIAN_POINT('Ctrl Pts',(-0.660837136749363,0.203994775542709,
-1.68821203654041));
#56648=CARTESIAN_POINT('Ctrl Pts',(-0.676672136897923,0.045841287298366,
-1.68077344574488));
#56649=CARTESIAN_POINT('Ctrl Pts',(-0.676650274159548,9.11169281613E-6,
-1.678617978381));
#56650=CARTESIAN_POINT('Ctrl Pts',(-0.676645363994687,5.65701016099623E-6,
-1.839182021619));
#56651=CARTESIAN_POINT('Ctrl Pts',(-0.676627054762735,-0.0623813489974528,
-1.83624804866027));
#56652=CARTESIAN_POINT('Ctrl Pts',(-0.65266894145479,-0.237120680884818,
-1.82803095226989));
#56653=CARTESIAN_POINT('Ctrl Pts',(-0.504159162883881,-0.493232229461368,
-1.81453073244784));
#56654=CARTESIAN_POINT('Ctrl Pts',(-0.207374009842694,-0.67412944880117,
-1.79868136215287));
#56655=CARTESIAN_POINT('Ctrl Pts',(0.139771257512638,-0.691316489946928,
-1.78283199185788));
#56656=CARTESIAN_POINT('Ctrl Pts',(0.45297352250471,-0.540619534986371,
-1.7669826215629));
#56657=CARTESIAN_POINT('Ctrl Pts',(0.656172617900346,-0.258634856925766,
-1.75113325126792));
#56658=CARTESIAN_POINT('Ctrl Pts',(0.700022293991506,0.0861584680346388,
-1.73528388097294));
#56659=CARTESIAN_POINT('Ctrl Pts',(0.573873797338617,0.410028484897529,
-1.71943451067796));
#56660=CARTESIAN_POINT('Ctrl Pts',(0.308361886447897,0.634324397044211,
-1.70358514038298));
#56661=CARTESIAN_POINT('Ctrl Pts',(-0.0320347212446137,0.704576660367049,
-1.687735770088));
#56662=CARTESIAN_POINT('Ctrl Pts',(-0.364651799452575,0.603724737653847,
-1.67188639979302));
#56663=CARTESIAN_POINT('Ctrl Pts',(-0.608714355716241,0.356260195424872,
-1.65603702949804));
#56664=CARTESIAN_POINT('Ctrl Pts',(-0.6749086000968,0.126542401434684,-1.6451355701067));
#56665=CARTESIAN_POINT('Ctrl Pts',(-0.676755222289058,0.00713188059781006,
-1.63951723414702));
#56666=CARTESIAN_POINT('Ctrl Pts',(-0.6767513059161,7.24714397433088E-6,
-1.63918202161899));
#56667=CARTESIAN_POINT('Origin',(0.,0.,-4.178617978381));
#56668=CARTESIAN_POINT('',(-0.676721208628825,1.57472380184304E-5,-2.078617978381));
#56669=CARTESIAN_POINT('',(-0.676719918585588,-1.59214003083719E-5,-2.039182021619));
#56670=CARTESIAN_POINT('',(-0.6767,-8.45931892044317E-14,-4.178617978381));
#56671=CARTESIAN_POINT('Ctrl Pts',(-0.676721208628825,1.57472380184313E-5,
-2.078617978381));
#56672=CARTESIAN_POINT('Ctrl Pts',(-0.676628683042819,-0.0931508258832454,
-2.07423507477139));
#56673=CARTESIAN_POINT('Ctrl Pts',(-0.633845182230617,-0.298702118546585,
-2.06456904773011));
#56674=CARTESIAN_POINT('Ctrl Pts',(-0.432319723520416,-0.557273858061672,
-2.04961989725718));
#56675=CARTESIAN_POINT('Ctrl Pts',(-0.113671183958779,-0.69608430391808,
-2.0337705269622));
#56676=CARTESIAN_POINT('Ctrl Pts',(0.232582038671535,-0.665852905311,-2.01792115666722));
#56677=CARTESIAN_POINT('Ctrl Pts',(0.522353457898419,-0.473921260596391,
-2.00207178637224));
#56678=CARTESIAN_POINT('Ctrl Pts',(0.685273012361204,-0.166899355160858,
-1.98622241607726));
#56679=CARTESIAN_POINT('Ctrl Pts',(0.681776209899179,0.180653524292269,
-1.97037304578227));
#56680=CARTESIAN_POINT('Ctrl Pts',(0.512712237794087,0.484335273792739,
-1.9545236754873));
#56681=CARTESIAN_POINT('Ctrl Pts',(0.219137740357689,0.670397752811446,
-1.93867430519231));
#56682=CARTESIAN_POINT('Ctrl Pts',(-0.12765365568297,0.693656284058958,
-1.92282493489733));
#56683=CARTESIAN_POINT('Ctrl Pts',(-0.443444770166212,0.548462607691666,
-1.90697556460235));
#56684=CARTESIAN_POINT('Ctrl Pts',(-0.636923641371969,0.289638431046473,
-1.89223991243024));
#56685=CARTESIAN_POINT('Ctrl Pts',(-0.676615993480196,0.0886165029668635,
-1.88278738368979));
#56686=CARTESIAN_POINT('Ctrl Pts',(-0.676707048125263,-1.71239118336441E-5,
-1.878617978381));
#56687=CARTESIAN_POINT('Ctrl Pts',(-0.676719918585588,-1.59214003083753E-5,
-2.039182021619));
#56688=CARTESIAN_POINT('Ctrl Pts',(-0.676739457480622,-0.0195730432971318,
-2.03826198660519));
#56689=CARTESIAN_POINT('Ctrl Pts',(-0.671136992488532,-0.151422004354565,
-2.03205882815972));
#56690=CARTESIAN_POINT('Ctrl Pts',(-0.588163460150873,-0.38925343651991,
-2.02057254628259));
#56691=CARTESIAN_POINT('Ctrl Pts',(-0.330838643304082,-0.622896689504703,
-2.00472317598761));
#56692=CARTESIAN_POINT('Ctrl Pts',(0.00682927878028947,-0.705271475852064,
-1.98887380569263));
#56693=CARTESIAN_POINT('Ctrl Pts',(0.342838732379053,-0.616373342447522,
-1.97302443539765));
#56694=CARTESIAN_POINT('Ctrl Pts',(0.59559089753061,-0.377790916351739,
-1.95717506510267));
#56695=CARTESIAN_POINT('Ctrl Pts',(0.703705720197163,-0.0474631758419071,
-1.94132569480769));
#56696=CARTESIAN_POINT('Ctrl Pts',(0.640927861859323,0.294390844952153,
-1.92547632451271));
#56697=CARTESIAN_POINT('Ctrl Pts',(0.422502724410463,0.56475299163877,-1.90962695421772));
#56698=CARTESIAN_POINT('Ctrl Pts',(0.101474153120063,0.697966682548511,
-1.89377758392275));
#56699=CARTESIAN_POINT('Ctrl Pts',(-0.244197091352646,0.661681399371415,
-1.87792821362777));
#56700=CARTESIAN_POINT('Ctrl Pts',(-0.53056585406773,0.464708906947766,
-1.86207884333278));
#56701=CARTESIAN_POINT('Ctrl Pts',(-0.658928445463778,0.212237031353743,
-1.84916344599653));
#56702=CARTESIAN_POINT('Ctrl Pts',(-0.676660023687023,0.049957196008536,
-1.84153117209193));
#56703=CARTESIAN_POINT('Ctrl Pts',(-0.676645363994687,5.65701016099623E-6,
-1.839182021619));
#56704=CARTESIAN_POINT('Origin',(0.,0.,-4.178617978381));
#56705=CARTESIAN_POINT('',(-0.676644996800385,-5.2859233725154E-6,-2.278617978381));
#56706=CARTESIAN_POINT('',(-0.676708376272384,1.70429511678338E-5,-2.23918202161899));
#56707=CARTESIAN_POINT('',(-0.6767,-8.45931892044317E-14,-4.178617978381));
#56708=CARTESIAN_POINT('Ctrl Pts',(-0.676644996800385,-5.28592337248335E-6,
-2.278617978381));
#56709=CARTESIAN_POINT('Ctrl Pts',(-0.676658801146923,-0.0503782471512948,
-2.2762490127163));
#56710=CARTESIAN_POINT('Ctrl Pts',(-0.658728598412653,-0.213080253371554,
-2.26859692361994));
#56711=CARTESIAN_POINT('Ctrl Pts',(-0.529697069227978,-0.465698948973474,
-2.25566171109192));
#56712=CARTESIAN_POINT('Ctrl Pts',(-0.24296095180248,-0.662136294219658,
-2.23981234079694));
#56713=CARTESIAN_POINT('Ctrl Pts',(0.102777454848793,-0.69777596046189,
-2.22396297050196));
#56714=CARTESIAN_POINT('Ctrl Pts',(0.423556685665886,-0.563962968865366,
-2.20811360020698));
#56715=CARTESIAN_POINT('Ctrl Pts',(0.641476531525165,-0.293193375992965,
-2.192264229912));
#56716=CARTESIAN_POINT('Ctrl Pts',(0.70361585560182,0.048777289484231,-2.17641485961702));
#56717=CARTESIAN_POINT('Ctrl Pts',(0.59488432200333,0.378902546386728,-2.16056548932204));
#56718=CARTESIAN_POINT('Ctrl Pts',(0.341687035524299,0.617012533080427,
-2.14471611902706));
#56719=CARTESIAN_POINT('Ctrl Pts',(0.00551214649170594,0.70528300168426,
-2.12886674873208));
#56720=CARTESIAN_POINT('Ctrl Pts',(-0.332001349667448,0.622277751524753,
-2.1130173784371));
#56721=CARTESIAN_POINT('Ctrl Pts',(-0.588889381071465,0.388154341834502,
-2.09716800814212));
#56722=CARTESIAN_POINT('Ctrl Pts',(-0.671276237328251,0.150578921577801,
-2.08570154145675));
#56723=CARTESIAN_POINT('Ctrl Pts',(-0.676740212780864,0.0191515538507402,
-2.07951819820305));
#56724=CARTESIAN_POINT('Ctrl Pts',(-0.676721208628825,1.57472380184313E-5,
-2.078617978381));
#56725=CARTESIAN_POINT('Ctrl Pts',(-0.676708376272384,1.704295116782E-5,
-2.23918202161899));
#56726=CARTESIAN_POINT('Ctrl Pts',(-0.676616933198787,-0.0890373128188941,
-2.23499280111844));
#56727=CARTESIAN_POINT('Ctrl Pts',(-0.6366424413202,-0.290479846329372,
-2.22552045718623));
#56728=CARTESIAN_POINT('Ctrl Pts',(-0.442419721672428,-0.549289799263099,
-2.21076498982235));
#56729=CARTESIAN_POINT('Ctrl Pts',(-0.126358004157817,-0.693893470559033,
-2.19491561952737));
#56730=CARTESIAN_POINT('Ctrl Pts',(0.220389350089783,-0.669987334258051,
-2.17906624923239));
#56731=CARTESIAN_POINT('Ctrl Pts',(0.513615856317125,-0.483376919017481,
-2.16321687893741));
#56732=CARTESIAN_POINT('Ctrl Pts',(0.682112396348077,-0.179379966683827,
-2.14736750864243));
#56733=CARTESIAN_POINT('Ctrl Pts',(0.684960124933254,0.168178836214988,
-2.13151813834745));
#56734=CARTESIAN_POINT('Ctrl Pts',(0.521467480303687,0.474895947218893,
-2.11566876805247));
#56735=CARTESIAN_POINT('Ctrl Pts',(0.231338127732153,0.666286097976378,
-2.09981939775749));
#56736=CARTESIAN_POINT('Ctrl Pts',(-0.114970948453971,0.695870803174554,
-2.08397002746251));
#56737=CARTESIAN_POINT('Ctrl Pts',(-0.433359697925381,0.556465511881219,
-2.06812065716753));
#56738=CARTESIAN_POINT('Ctrl Pts',(-0.634135429768427,0.297861104444726,
-2.05319132188636));
#56739=CARTESIAN_POINT('Ctrl Pts',(-0.676627259148345,0.0927299532173215,
-2.04354511003685));
#56740=CARTESIAN_POINT('Ctrl Pts',(-0.676719918585588,-1.59214003083753E-5,
-2.039182021619));
#56741=CARTESIAN_POINT('Origin',(0.,0.,-4.178617978381));
#56742=CARTESIAN_POINT('',(-0.676750583136638,-7.642249214652E-6,-2.478617978381));
#56743=CARTESIAN_POINT('',(-0.67664966423598,-8.77515312422417E-6,-2.43918202161899));
#56744=CARTESIAN_POINT('',(-0.6767,-8.45931892044317E-14,-4.178617978381));
#56745=CARTESIAN_POINT('Ctrl Pts',(-0.676750583136638,-7.6422492146077E-6,
-2.478617978381));
#56746=CARTESIAN_POINT('Ctrl Pts',(-0.676754922059666,-0.00755345283786624,
-2.47826295066122));
#56747=CARTESIAN_POINT('Ctrl Pts',(-0.674792200770675,-0.127385273327122,
-2.47262479950977));
#56748=CARTESIAN_POINT('Ctrl Pts',(-0.608047966749425,-0.357396371491931,
-2.46170352492667));
#56749=CARTESIAN_POINT('Ctrl Pts',(-0.363523686348719,-0.604404687016196,
-2.44585415463169));
#56750=CARTESIAN_POINT('Ctrl Pts',(-0.0307188426589624,-0.704635259499128,
-2.43000478433671));
#56751=CARTESIAN_POINT('Ctrl Pts',(0.309545973614037,-0.633747415334411,
-2.41415541404173));
#56752=CARTESIAN_POINT('Ctrl Pts',(0.574638541308189,-0.408956040506685,
-2.39830604374675));
#56753=CARTESIAN_POINT('Ctrl Pts',(0.700181979140083,-0.0848510006492837,
-2.38245667345177));
#56754=CARTESIAN_POINT('Ctrl Pts',(0.655688465200883,0.259859833037388,
-2.36660730315679));
#56755=CARTESIAN_POINT('Ctrl Pts',(0.451963106890093,0.54146453829772,-2.35075793286181));
#56756=CARTESIAN_POINT('Ctrl Pts',(0.138479955179697,0.691576314109395,
-2.33490856256682));
#56757=CARTESIAN_POINT('Ctrl Pts',(-0.20863261025693,0.673740996348811,
-2.31905919227184));
#56758=CARTESIAN_POINT('Ctrl Pts',(-0.505079414298638,0.492289834828481,
-2.30320982197686));
#56759=CARTESIAN_POINT('Ctrl Pts',(-0.652893361036711,0.236277703536981,
-2.28972941734659));
#56760=CARTESIAN_POINT('Ctrl Pts',(-0.676628015531182,0.0619604733928406,
-2.28153213614796));
#56761=CARTESIAN_POINT('Ctrl Pts',(-0.676644996800385,-5.28592337248335E-6,
-2.278617978381));
#56762=CARTESIAN_POINT('Ctrl Pts',(-0.67664966423598,-8.77515312422764E-6,
-2.43918202161899));
#56763=CARTESIAN_POINT('Ctrl Pts',(-0.676670888840999,-0.0462624044265438,
-2.43700673906336));
#56764=CARTESIAN_POINT('Ctrl Pts',(-0.660645579160593,-0.204838031955816,
-2.42954833307605));
#56765=CARTESIAN_POINT('Ctrl Pts',(-0.538109309602317,-0.455952699979421,
-2.4168068036571));
#56766=CARTESIAN_POINT('Ctrl Pts',(-0.255006572123388,-0.657591166206698,
-2.40095743336211));
#56767=CARTESIAN_POINT('Ctrl Pts',(0.0900236949082282,-0.699535723215246,
-2.38510806306714));
#56768=CARTESIAN_POINT('Ctrl Pts',(0.413191995871872,-0.571600269634842,
-2.36925869277215));
#56769=CARTESIAN_POINT('Ctrl Pts',(0.63601794360821,-0.304853520740027,
-2.35340932247718));
#56770=CARTESIAN_POINT('Ctrl Pts',(0.704388970160089,0.0359259295776118,
-2.33755995218219));
#56771=CARTESIAN_POINT('Ctrl Pts',(0.601701390641733,0.367980882926015,
-2.32171058188722));
#56772=CARTESIAN_POINT('Ctrl Pts',(0.352892554951089,0.610672857067759,
-2.30586121159223));
#56773=CARTESIAN_POINT('Ctrl Pts',(0.0183848921922413,0.705064883140754,
-2.29001184129726));
#56774=CARTESIAN_POINT('Ctrl Pts',(-0.320587482770208,0.628234159840316,
-2.27416247100227));
#56775=CARTESIAN_POINT('Ctrl Pts',(-0.581706214008261,0.398838782321105,
-2.2583131007073));
#56776=CARTESIAN_POINT('Ctrl Pts',(-0.669880488577138,0.158819887446242,
-2.24665295091287));
#56777=CARTESIAN_POINT('Ctrl Pts',(-0.67673225418624,0.0232712070114671,
-2.2402759245501));
#56778=CARTESIAN_POINT('Ctrl Pts',(-0.676708376272384,1.704295116782E-5,
-2.23918202161899));
#56779=CARTESIAN_POINT('Origin',(0.,0.,-4.178617978381));
#56780=CARTESIAN_POINT('',(-0.676672441952873,1.56724317931045E-5,-2.678617978381));
#56781=CARTESIAN_POINT('',(-0.676756127719321,-3.58750326429069E-6,-2.639182021619));
#56782=CARTESIAN_POINT('',(-0.6767,-8.45931892044317E-14,-4.178617978381));
#56783=CARTESIAN_POINT('Ctrl Pts',(-0.676672441952873,1.56724317930956E-5,
-2.678617978381));
#56784=CARTESIAN_POINT('Ctrl Pts',(-0.676606295786303,-0.0770395337766664,
-2.67499376517447));
#56785=CARTESIAN_POINT('Ctrl Pts',(-0.644301914118974,-0.266474457412185,
-2.66608642853628));
#56786=CARTESIAN_POINT('Ctrl Pts',(-0.471028835749505,-0.52496317215227,
-2.65189596846643));
#56787=CARTESIAN_POINT('Ctrl Pts',(-0.163111735027927,-0.686184419904654,
-2.63604659817145));
#56788=CARTESIAN_POINT('Ctrl Pts',(0.184416528289274,-0.680767978328477,
-2.62019722787647));
#56789=CARTESIAN_POINT('Ctrl Pts',(0.487159828181642,-0.510029212917986,
-2.60434785758149));
#56790=CARTESIAN_POINT('Ctrl Pts',(0.671597923602639,-0.21543148617677,
-2.58849848728651));
#56791=CARTESIAN_POINT('Ctrl Pts',(0.692940613618548,0.131483087207663,
-2.57264911699153));
#56792=CARTESIAN_POINT('Ctrl Pts',(0.546004894294652,0.446467413850098,
-2.55679974669655));
#56793=CARTESIAN_POINT('Ctrl Pts',(0.266473634605688,0.653028558551418,
-2.54095037640157));
#56794=CARTESIAN_POINT('Ctrl Pts',(-0.0777698940442144,0.701003808694404,
-2.52510100610659));
#56795=CARTESIAN_POINT('Ctrl Pts',(-0.403127252931393,0.578742528390386,
-2.50925163581161));
#56796=CARTESIAN_POINT('Ctrl Pts',(-0.625491336998928,0.321822386292196,
-2.49375729323641));
#56797=CARTESIAN_POINT('Ctrl Pts',(-0.676690355084629,0.104734817936979,
-2.48354607409288));
#56798=CARTESIAN_POINT('Ctrl Pts',(-0.676750583136638,-7.6422492146077E-6,
-2.478617978381));
#56799=CARTESIAN_POINT('Ctrl Pts',(-0.67675612771932,-3.5875032643011E-6,
-2.639182021619));
#56800=CARTESIAN_POINT('Ctrl Pts',(-0.676757135496254,-0.00343274748612147,
-2.63902067700827));
#56801=CARTESIAN_POINT('Ctrl Pts',(-0.675895944019102,-0.119146993585894,
-2.63357620896589));
#56802=CARTESIAN_POINT('Ctrl Pts',(-0.614470285968358,-0.346238012588408,
-2.62284861749184));
#56803=CARTESIAN_POINT('Ctrl Pts',(-0.374495434261829,-0.597668523026142,
-2.60699924719686));
#56804=CARTESIAN_POINT('Ctrl Pts',(-0.0435755654152151,-0.703957146279481,
-2.59114987690188));
#56805=CARTESIAN_POINT('Ctrl Pts',(0.29792648997097,-0.639292030509363,
-2.5753005066069));
#56806=CARTESIAN_POINT('Ctrl Pts',(0.567078051177426,-0.419376892033906,
-2.55945113631192));
#56807=CARTESIAN_POINT('Ctrl Pts',(0.698516523342481,-0.097617418101175,
-2.54360176601694));
#56808=CARTESIAN_POINT('Ctrl Pts',(0.660322494344382,0.247848133263131,
-2.52775239572196));
#56809=CARTESIAN_POINT('Ctrl Pts',(0.461771261834565,0.533124559031865,
-2.51190302542698));
#56810=CARTESIAN_POINT('Ctrl Pts',(0.151080356900915,0.688933392613464,
-2.496053655132));
#56811=CARTESIAN_POINT('Ctrl Pts',(-0.196299928972631,0.67743695764591,
-2.48020428483702));
#56812=CARTESIAN_POINT('Ctrl Pts',(-0.496009405614011,0.501427126551448,
-2.46435491454204));
#56813=CARTESIAN_POINT('Ctrl Pts',(-0.650662304876479,0.244516783651035,
-2.4506808268027));
#56814=CARTESIAN_POINT('Ctrl Pts',(-0.67661934049947,0.066074097321367,
-2.44228986249502));
#56815=CARTESIAN_POINT('Ctrl Pts',(-0.67664966423598,-8.77515312422764E-6,
-2.43918202161899));
#56816=CARTESIAN_POINT('Origin',(0.,0.,-4.178617978381));
#56817=CARTESIAN_POINT('',(-0.67667522099595,-1.60756434531244E-5,-2.878617978381));
#56818=CARTESIAN_POINT('',(-0.676662334990091,1.3602642141286E-5,-2.839182021619));
#56819=CARTESIAN_POINT('',(-0.6767,-8.45931892044317E-14,-4.178617978381));
#56820=CARTESIAN_POINT('Ctrl Pts',(-0.67667522099595,-1.6075643453118E-5,
-2.878617978381));
#56821=CARTESIAN_POINT('Ctrl Pts',(-0.676705554749602,-0.0342520940821256,
-2.87700770311939));
#56822=CARTESIAN_POINT('Ctrl Pts',(-0.66577840727492,-0.180793269959295,
-2.87011430442611));
#56823=CARTESIAN_POINT('Ctrl Pts',(-0.56161486994617,-0.426665248267367,
-2.85793778230118));
#56824=CARTESIAN_POINT('Ctrl Pts',(-0.289645737183324,-0.643086186413016,
-2.84208841200619));
#56825=CARTESIAN_POINT('Ctrl Pts',(0.0526629354583269,-0.703335703240367,
-2.82623904171122));
#56826=CARTESIAN_POINT('Ctrl Pts',(0.382182582841647,-0.592782396496553,
-2.81038967141623));
#56827=CARTESIAN_POINT('Ctrl Pts',(0.618890413665208,-0.33827378275151,
-2.79454030112126));
#56828=CARTESIAN_POINT('Ctrl Pts',(0.705302689111543,-0.0016164639601243,
-2.77869093082627));
#56829=CARTESIAN_POINT('Ctrl Pts',(0.620434464765853,0.335433407928336,
-2.7628415605313));
#56830=CARTESIAN_POINT('Ctrl Pts',(0.384895717176935,0.591024350701866,
-2.74699219023631));
#56831=CARTESIAN_POINT('Ctrl Pts',(0.0558862770419258,0.703086922266445,
-2.73114281994134));
#56832=CARTESIAN_POINT('Ctrl Pts',(-0.286694966534403,0.644407085922823,
-2.71529344964635));
#56833=CARTESIAN_POINT('Ctrl Pts',(-0.559653255436154,0.429235052044242,
-2.69944407935137));
#56834=CARTESIAN_POINT('Ctrl Pts',(-0.665363249906537,0.182862978936254,
-2.68721892226292));
#56835=CARTESIAN_POINT('Ctrl Pts',(-0.676702719021528,0.0352861331343808,
-2.68027688860613));
#56836=CARTESIAN_POINT('Ctrl Pts',(-0.676672441952873,1.56724317930956E-5,
-2.678617978381));
#56837=CARTESIAN_POINT('Ctrl Pts',(-0.67666233499009,1.36026421412444E-5,
-2.839182021619));
#56838=CARTESIAN_POINT('Ctrl Pts',(-0.676609147890392,-0.0729267869494966,
-2.83575149152153));
#56839=CARTESIAN_POINT('Ctrl Pts',(-0.646758396857733,-0.258240144278789,
-2.8270378379924));
#56840=CARTESIAN_POINT('Ctrl Pts',(-0.48053261167355,-0.516277931755177,
-2.81304106103161));
#56841=CARTESIAN_POINT('Ctrl Pts',(-0.175609613684971,-0.683092788192513,
-2.79719169073663));
#56842=CARTESIAN_POINT('Ctrl Pts',(0.171959616715022,-0.684020748163701,
-2.78134232044165));
#56843=CARTESIAN_POINT('Ctrl Pts',(0.477769004781086,-0.518836459560908,
-2.76549295014667));
#56844=CARTESIAN_POINT('Ctrl Pts',(0.667553719770789,-0.227654397979453,
-2.74964357985169));
#56845=CARTESIAN_POINT('Ctrl Pts',(0.695225151307124,0.118812805240822,
-2.7337942095567));
#56846=CARTESIAN_POINT('Ctrl Pts',(0.55406338084068,0.436426699126669,-2.71794483926173));
#56847=CARTESIAN_POINT('Ctrl Pts',(0.278349092353365,0.648055766493336,
-2.70209546896675));
#56848=CARTESIAN_POINT('Ctrl Pts',(-0.0649613819857274,0.702306565930941,
-2.68624609867177));
#56849=CARTESIAN_POINT('Ctrl Pts',(-0.392496192704833,0.586004464497855,
-2.67039672837678));
#56850=CARTESIAN_POINT('Ctrl Pts',(-0.622350605748701,0.330025687005806,
-2.65470870269253));
#56851=CARTESIAN_POINT('Ctrl Pts',(-0.676724136501708,0.108852846529397,
-2.64430380043993));
#56852=CARTESIAN_POINT('Ctrl Pts',(-0.67675612771932,-3.5875032643011E-6,
-2.639182021619));
#56853=CARTESIAN_POINT('Origin',(0.,0.,-4.178617978381));
#56854=CARTESIAN_POINT('',(-0.676748670238398,8.58863998659695E-6,-3.078617978381));
#56855=CARTESIAN_POINT('',(-0.676687048566771,-1.71712397221968E-5,-3.039182021619));
#56856=CARTESIAN_POINT('',(-0.6767,-8.45931892044317E-14,-4.178617978381));
#56857=CARTESIAN_POINT('Ctrl Pts',(-0.676748670238398,8.58863998661613E-6,
-3.078617978381));
#56858=CARTESIAN_POINT('Ctrl Pts',(-0.676682926446315,-0.103701028300201,
-3.07373851763264));
#56859=CARTESIAN_POINT('Ctrl Pts',(-0.626265638634916,-0.319761561202685,
-3.06357593345262));
#56860=CARTESIAN_POINT('Ctrl Pts',(-0.405775812394436,-0.576888625558993,
-3.04813022584094));
#56861=CARTESIAN_POINT('Ctrl Pts',(-0.0809822831169064,-0.700639968917618,
-3.03228085554596));
#56862=CARTESIAN_POINT('Ctrl Pts',(0.263477534324128,-0.654243139154081,
-3.01643148525098));
#56863=CARTESIAN_POINT('Ctrl Pts',(0.543952676164601,-0.448965457821732,
-3.000582114956));
#56864=CARTESIAN_POINT('Ctrl Pts',(0.692330652242036,-0.134657952568069,
-2.98473274466102));
#56865=CARTESIAN_POINT('Ctrl Pts',(0.672578346146962,0.212350805314992,
-2.96888337436604));
#56866=CARTESIAN_POINT('Ctrl Pts',(0.489492542171056,0.507790850038306,
-2.95303400407106));
#56867=CARTESIAN_POINT('Ctrl Pts',(0.1875350416004,0.679915512689367,-2.93718463377608));
#56868=CARTESIAN_POINT('Ctrl Pts',(-0.159964743367749,0.686924870057126,
-2.9213352634811));
#56869=CARTESIAN_POINT('Ctrl Pts',(-0.468617602588818,0.527116722147587,
-2.90548589318612));
#56870=CARTESIAN_POINT('Ctrl Pts',(-0.643671614274052,0.26854177142875,
-2.89124679815276));
#56871=CARTESIAN_POINT('Ctrl Pts',(-0.676606033277398,0.0780722491725114,
-2.88229082655105));
#56872=CARTESIAN_POINT('Ctrl Pts',(-0.67667522099595,-1.6075643453118E-5,
-2.878617978381));
#56873=CARTESIAN_POINT('Ctrl Pts',(-0.676687048566771,-1.71712397222107E-5,
-3.039182021619));
#56874=CARTESIAN_POINT('Ctrl Pts',(-0.676716369911433,-0.0301337864271384,
-3.03776542946644));
#56875=CARTESIAN_POINT('Ctrl Pts',(-0.667382347146982,-0.172551068097945,
-3.03106571388223));
#56876=CARTESIAN_POINT('Ctrl Pts',(-0.569309303103972,-0.416342900862349,
-3.01908287486635));
#56877=CARTESIAN_POINT('Ctrl Pts',(-0.301335854323042,-0.63769208604044,
-3.00323350457137));
#56878=CARTESIAN_POINT('Ctrl Pts',(0.0398160418543145,-0.704179789904724,
-2.98738413427639));
#56879=CARTESIAN_POINT('Ctrl Pts',(0.371298739751515,-0.599659686454028,
-2.97153476398141));
#56880=CARTESIAN_POINT('Ctrl Pts',(0.612612727535191,-0.349514148155837,
-2.95568539368643));
#56881=CARTESIAN_POINT('Ctrl Pts',(0.705155675918236,-0.0144902180625897,
-2.93983602339145));
#56882=CARTESIAN_POINT('Ctrl Pts',(0.62645382619254,0.324052615091952,-2.92398665309647));
#56883=CARTESIAN_POINT('Ctrl Pts',(0.39561967057411,0.583900308232526,-2.90813728280149));
#56884=CARTESIAN_POINT('Ctrl Pts',(0.0687105446633539,0.70194968106786,
-2.89228791250651));
#56885=CARTESIAN_POINT('Ctrl Pts',(-0.274884717019473,0.649532821378821,
-2.87643854221153));
#56886=CARTESIAN_POINT('Ctrl Pts',(-0.551725105308022,0.439378995711058,
-2.86058917191655));
#56887=CARTESIAN_POINT('Ctrl Pts',(-0.663660295032008,0.191105462586324,
-2.84817033171904));
#56888=CARTESIAN_POINT('Ctrl Pts',(-0.676691057684125,0.0394036898040259,
-2.84103461495319));
#56889=CARTESIAN_POINT('Ctrl Pts',(-0.67666233499009,1.36026421412444E-5,
-2.839182021619));
#56890=CARTESIAN_POINT('Origin',(0.,0.,-4.178617978381));
#56891=CARTESIAN_POINT('',(-0.676644198931752,4.36460036937442E-6,-3.278617978381));
#56892=CARTESIAN_POINT('',(-0.676739402418013,1.19727938200573E-5,-3.23918202161899));
#56893=CARTESIAN_POINT('',(-0.6767,-8.45931892044317E-14,-4.178617978381));
#56894=CARTESIAN_POINT('Ctrl Pts',(-0.676644198931752,4.36460036935815E-6,
-3.278617978381));
#56895=CARTESIAN_POINT('Ctrl Pts',(-0.676630431341335,-0.060927441302453,
-3.27575245557756));
#56896=CARTESIAN_POINT('Ctrl Pts',(-0.653440485571609,-0.234208622315155,
-3.26760380934245));
#56897=CARTESIAN_POINT('Ctrl Pts',(-0.507330627672634,-0.489969519918335,
-3.25417203967569));
#56898=CARTESIAN_POINT('Ctrl Pts',(-0.211718659443945,-0.672777604760268,
-3.23832266938071));
#56899=CARTESIAN_POINT('Ctrl Pts',(0.135308507343731,-0.692203802405131,
-3.22247329908573));
#56900=CARTESIAN_POINT('Ctrl Pts',(0.449476436357704,-0.543530522954218,
-3.20662392879074));
#56901=CARTESIAN_POINT('Ctrl Pts',(0.65449045194897,-0.262862596295751,
-3.19077455849577));
#56902=CARTESIAN_POINT('Ctrl Pts',(0.700563556851036,0.0816406702320175,
-3.17492518820078));
#56903=CARTESIAN_POINT('Ctrl Pts',(0.576507045056651,0.406317761393417,
-3.1590758179058));
#56904=CARTESIAN_POINT('Ctrl Pts',(0.312447643247322,0.632321885160478,
-3.14322644761082));
#56905=CARTESIAN_POINT('Ctrl Pts',(-0.0274886683206437,0.704768663702968,
-3.12737707731584));
#56906=CARTESIAN_POINT('Ctrl Pts',(-0.360749444800962,0.606064628814044,
-3.11152770702087));
#56907=CARTESIAN_POINT('Ctrl Pts',(-0.606403373669456,0.360179739333031,
-3.09567833672588));
#56908=CARTESIAN_POINT('Ctrl Pts',(-0.674503132757475,0.129454074981309,
-3.08470842717926));
#56909=CARTESIAN_POINT('Ctrl Pts',(-0.676754109018807,0.00858816421545373,
-3.0790216410643));
#56910=CARTESIAN_POINT('Ctrl Pts',(-0.676748670238398,8.58863998661613E-6,
-3.078617978381));
#56911=CARTESIAN_POINT('Ctrl Pts',(-0.676739402418013,1.19727938200608E-5,
-3.23918202161899));
#56912=CARTESIAN_POINT('Ctrl Pts',(-0.676657269998734,-0.0995849951729056,
-3.23449624397969));
#56913=CARTESIAN_POINT('Ctrl Pts',(-0.629292425415603,-0.311551144554621,
-3.22452734290874));
#56914=CARTESIAN_POINT('Ctrl Pts',(-0.41623826497985,-0.56938580985635,
-3.20927531840611));
#56915=CARTESIAN_POINT('Ctrl Pts',(-0.0937577048939214,-0.699045053249238,
-3.19342594811114));
#56916=CARTESIAN_POINT('Ctrl Pts',(0.251491613629344,-0.658943443683383,
-3.17757657781615));
#56917=CARTESIAN_POINT('Ctrl Pts',(0.535666999015903,-0.458819528643346,
-3.16172720752118));
#56918=CARTESIAN_POINT('Ctrl Pts',(0.689757368805666,-0.147272760134018,
-3.1458778372262));
#56919=CARTESIAN_POINT('Ctrl Pts',(0.676342370066224,0.20003872663164,-3.13002846693121));
#56920=CARTESIAN_POINT('Ctrl Pts',(0.498679792288921,0.498771449124632,
-3.11417909663624));
#56921=CARTESIAN_POINT('Ctrl Pts',(0.199914423641749,0.676379122178673,
-3.09832972634125));
#56922=CARTESIAN_POINT('Ctrl Pts',(-0.147399522694991,0.689730291062018,
-3.08248035604627));
#56923=CARTESIAN_POINT('Ctrl Pts',(-0.458917966893342,0.535582667159503,
-3.0666309857513));
#56924=CARTESIAN_POINT('Ctrl Pts',(-0.641107555059538,0.276772949731498,
-3.05219820760887));
#56925=CARTESIAN_POINT('Ctrl Pts',(-0.67660701713636,0.0821849180722907,
-3.0430485528981));
#56926=CARTESIAN_POINT('Ctrl Pts',(-0.676687048566771,-1.71712397222107E-5,
-3.039182021619));
#56927=CARTESIAN_POINT('Origin',(0.,0.,-4.178617978381));
#56928=CARTESIAN_POINT('',(-0.676724334253827,-1.52803889846311E-5,-3.478617978381));
#56929=CARTESIAN_POINT('',(-0.676642561475797,5.96081397241655E-7,-3.439182021619));
#56930=CARTESIAN_POINT('',(-0.6767,-8.45931892044317E-14,-4.178617978381));
#56931=CARTESIAN_POINT('Ctrl Pts',(-0.676724334253826,-1.5280388984627E-5,
-3.478617978381));
#56932=CARTESIAN_POINT('Ctrl Pts',(-0.676742001449043,-0.0181170211682754,
-3.47776639352247));
#56933=CARTESIAN_POINT('Ctrl Pts',(-0.671614576287041,-0.148509662737602,
-3.47163168523228));
#56934=CARTESIAN_POINT('Ctrl Pts',(-0.590662385922995,-0.385450959342922,
-3.46021385351043));
#56935=CARTESIAN_POINT('Ctrl Pts',(-0.334850209657572,-0.620749412673154,
-3.44436448321545));
#56936=CARTESIAN_POINT('Ctrl Pts',(0.00227926788749094,-0.70530085860637,
-3.42851511292047));
#56937=CARTESIAN_POINT('Ctrl Pts',(0.338855232525197,-0.618572249312001,
-3.41266574262549));
#56938=CARTESIAN_POINT('Ctrl Pts',(0.593141288900064,-0.381625349818476,
-3.39681637233051));
#56939=CARTESIAN_POINT('Ctrl Pts',(0.703384882402956,-0.0520019560290773,
-3.38096700203553));
#56940=CARTESIAN_POINT('Ctrl Pts',(0.642813709332344,0.290249946284879,
-3.36511763174055));
#56941=CARTESIAN_POINT('Ctrl Pts',(0.426137285130135,0.562015578472108,
-3.34926826144557));
#56942=CARTESIAN_POINT('Ctrl Pts',(0.105974785652812,0.697297526906368,
-3.33341889115059));
#56943=CARTESIAN_POINT('Ctrl Pts',(-0.239923351207117,0.663243003558396,
-3.31756952085561));
#56944=CARTESIAN_POINT('Ctrl Pts',(-0.527556870419987,0.468122040387345,
-3.30172015056063));
#56945=CARTESIAN_POINT('Ctrl Pts',(-0.658234470612573,0.215149858671953,
-3.28873630306909));
#56946=CARTESIAN_POINT('Ctrl Pts',(-0.676655814450987,0.0514116582543703,
-3.28103557900922));
#56947=CARTESIAN_POINT('Ctrl Pts',(-0.676644198931752,4.36460036935815E-6,
-3.278617978381));
#56948=CARTESIAN_POINT('Ctrl Pts',(-0.676642561475797,5.96081397224307E-7,
-3.439182021619));
#56949=CARTESIAN_POINT('Ctrl Pts',(-0.67664081343884,-0.056813170325692,
-3.43651018192461));
#56950=CARTESIAN_POINT('Ctrl Pts',(-0.655567470475998,-0.225968086496106,
-3.42855521879857));
#56951=CARTESIAN_POINT('Ctrl Pts',(-0.51618960975049,-0.480627486193364,
-3.41531713224086));
#56952=CARTESIAN_POINT('Ctrl Pts',(-0.223963722768737,-0.6688009753155,
-3.39946776194589));
#56953=CARTESIAN_POINT('Ctrl Pts',(0.122651037193902,-0.694558288968156,
-3.3836183916509));
#56954=CARTESIAN_POINT('Ctrl Pts',(0.43948038548163,-0.551644346002168,
-3.36776902135592));
#56955=CARTESIAN_POINT('Ctrl Pts',(0.649583329296276,-0.274765339880352,
-3.35191965106094));
#56956=CARTESIAN_POINT('Ctrl Pts',(0.701937041446152,0.0688395492796521,
-3.33607028076596));
#56957=CARTESIAN_POINT('Ctrl Pts',(0.583827590563321,0.39572697430961,-3.32022091047098));
#56958=CARTESIAN_POINT('Ctrl Pts',(0.323937478628386,0.626513370678621,
-3.304371540176));
#56959=CARTESIAN_POINT('Ctrl Pts',(-0.0146198127989899,0.705153000967117,
-3.28852216988102));
#56960=CARTESIAN_POINT('Ctrl Pts',(-0.349626729498273,0.612548482750179,
-3.27267279958604));
#56961=CARTESIAN_POINT('Ctrl Pts',(-0.599727914383955,0.371188526772956,
-3.25682342929106));
#56962=CARTESIAN_POINT('Ctrl Pts',(-0.673304323117296,0.137693307660308,
-3.24565983663537));
#56963=CARTESIAN_POINT('Ctrl Pts',(-0.676749872708934,0.0127086550366688,
-3.23977936741135));
#56964=CARTESIAN_POINT('Ctrl Pts',(-0.676739402418013,1.19727938200608E-5,
-3.23918202161899));
#56965=CARTESIAN_POINT('Origin',(0.,0.,-4.178617978381));
#56966=CARTESIAN_POINT('',(-0.676703788167417,1.73951649274827E-5,-3.678617978381));
#56967=CARTESIAN_POINT('',(-0.67673605652177,-1.28860430050337E-5,-3.639182021619));
#56968=CARTESIAN_POINT('',(-0.6767,-8.45931892044317E-14,-4.178617978381));
#56969=CARTESIAN_POINT('Ctrl Pts',(-0.676703788167417,1.73951649275021E-5,
-3.678617978381));
#56970=CARTESIAN_POINT('Ctrl Pts',(-0.676613881463619,-0.0875835708292743,
-3.67449720803573));
#56971=CARTESIAN_POINT('Ctrl Pts',(-0.637609911674448,-0.287573235928348,
-3.66509331425879));
#56972=CARTESIAN_POINT('Ctrl Pts',(-0.445954115113484,-0.546424125806921,
-3.6504062970502));
#56973=CARTESIAN_POINT('Ctrl Pts',(-0.130831839792564,-0.693063915639031,
-3.63455692675522));
#56974=CARTESIAN_POINT('Ctrl Pts',(0.21606252083174,-0.671395152184437,
-3.61870755646024));
#56975=CARTESIAN_POINT('Ctrl Pts',(0.510486794197391,-0.48668032805703,
-3.60285818616526));
#56976=CARTESIAN_POINT('Ctrl Pts',(0.680940981975007,-0.183776692274722,
-3.58700881587028));
#56977=CARTESIAN_POINT('Ctrl Pts',(0.686030833613329,0.163756498125624,
-3.5711594455753));
#56978=CARTESIAN_POINT('Ctrl Pts',(0.524520293312469,0.471521960898263,
-3.55531007528032));
#56979=CARTESIAN_POINT('Ctrl Pts',(0.235631679485712,0.664779818244593,
-3.53946070498533));
#56980=CARTESIAN_POINT('Ctrl Pts',(-0.110479333395072,0.696598028792635,
-3.52361133469035));
#56981=CARTESIAN_POINT('Ctrl Pts',(-0.429760793823647,0.55924963662321,
-3.50776196439537));
#56982=CARTESIAN_POINT('Ctrl Pts',(-0.633128840107847,0.30076613753894,
-3.49276417895892));
#56983=CARTESIAN_POINT('Ctrl Pts',(-0.676632396431899,0.0941838610127268,
-3.48304951695413));
#56984=CARTESIAN_POINT('Ctrl Pts',(-0.676724334253826,-1.5280388984627E-5,
-3.478617978381));
#56985=CARTESIAN_POINT('Ctrl Pts',(-0.67673605652177,-1.28860430050285E-5,
-3.639182021619));
#56986=CARTESIAN_POINT('Ctrl Pts',(-0.676748229532135,-0.0139968950353071,
-3.63852411986953));
#56987=CARTESIAN_POINT('Ctrl Pts',(-0.672913840421779,-0.140269491848012,
-3.6325830946884));
#56988=CARTESIAN_POINT('Ctrl Pts',(-0.597599687597092,-0.374605270350371,
-3.62135894607561));
#56989=CARTESIAN_POINT('Ctrl Pts',(-0.346125077999637,-0.614533907095192,
-3.60550957578063));
#56990=CARTESIAN_POINT('Ctrl Pts',(-0.0105951019105329,-0.705224955685239,
-3.58966020548565));
#56991=CARTESIAN_POINT('Ctrl Pts',(0.32750786099247,-0.624654379983339,
-3.57381083519067));
#56992=CARTESIAN_POINT('Ctrl Pts',(0.586076588355783,-0.392388489065435,
-3.55796146489568));
#56993=CARTESIAN_POINT('Ctrl Pts',(0.702318492816257,-0.0648323094657422,
-3.54211209460071));
#56994=CARTESIAN_POINT('Ctrl Pts',(0.648004599968331,0.278468188664054,
-3.52626272430573));
#56995=CARTESIAN_POINT('Ctrl Pts',(0.436324864834359,0.55414357890779,-3.51041335401075));
#56996=CARTESIAN_POINT('Ctrl Pts',(0.118685033304739,0.695246975223788,
-3.49456398371577));
#56997=CARTESIAN_POINT('Ctrl Pts',(-0.227777078549499,0.667511869700924,
-3.47871461342078));
#56998=CARTESIAN_POINT('Ctrl Pts',(-0.518924256183446,0.477673643863711,
-3.46286524312581));
#56999=CARTESIAN_POINT('Ctrl Pts',(-0.65621553862413,0.223391456722108,
-3.44968771252521));
#57000=CARTESIAN_POINT('Ctrl Pts',(-0.67664426989434,0.0555267058940655,
-3.44179330535627));
#57001=CARTESIAN_POINT('Ctrl Pts',(-0.676642561475797,5.96081397224307E-7,
-3.439182021619));
#57002=CARTESIAN_POINT('Origin',(1.87869726832665E-16,-4.25270154953079E-17,
-0.0711000000000002));
#57003=CARTESIAN_POINT('',(0.533647856309012,-0.584002718706682,-0.0711000000000004));
#57004=CARTESIAN_POINT('Ctrl Pts',(-0.657933019064465,-0.158364055658306,
-0.0711000000000003));
#57005=CARTESIAN_POINT('Ctrl Pts',(-0.65503062620215,-0.177074058470794,
-0.0711000000000003));
#57006=CARTESIAN_POINT('Ctrl Pts',(-0.651342440307925,-0.195634100037483,
-0.0710999999999999));
#57007=CARTESIAN_POINT('Ctrl Pts',(-0.646874620641261,-0.213993464998097,
-0.0710999999999998));
#57008=CARTESIAN_POINT('Ctrl Pts',(-0.640039981846469,-0.242078669274306,
-0.0710999999999997));
#57009=CARTESIAN_POINT('Ctrl Pts',(-0.631382480356379,-0.269694614707558,
-0.0711));
#57010=CARTESIAN_POINT('Ctrl Pts',(-0.62100840580272,-0.296696933525342,
-0.0710999999999998));
#57011=CARTESIAN_POINT('Ctrl Pts',(-0.616895281241109,-0.307402842777815,
-0.0710999999999997));
#57012=CARTESIAN_POINT('Ctrl Pts',(-0.612511970360756,-0.318012260843023,
-0.0710999999999991));
#57013=CARTESIAN_POINT('Ctrl Pts',(-0.607863785080036,-0.328515943120043,
-0.0710999999999991));
#57014=CARTESIAN_POINT('Ctrl Pts',(-0.604119622512866,-0.336976770652498,
-0.0710999999999991));
#57015=CARTESIAN_POINT('Ctrl Pts',(-0.600206902465123,-0.34536129242641,
-0.0710999999999998));
#57016=CARTESIAN_POINT('Ctrl Pts',(-0.596131845457498,-0.353659680525224,
-0.0710999999999997));
#57017=CARTESIAN_POINT('Ctrl Pts',(-0.581559334527423,-0.38333493440406,
-0.0710999999999993));
#57018=CARTESIAN_POINT('Ctrl Pts',(-0.56490503752703,-0.411931064563356,
-0.0710999999999997));
#57019=CARTESIAN_POINT('Ctrl Pts',(-0.546315461068867,-0.439236112401077,
-0.071099999999999));
#57020=CARTESIAN_POINT('Ctrl Pts',(-0.53873175404231,-0.450375337848918,
-0.0710999999999987));
#57021=CARTESIAN_POINT('Ctrl Pts',(-0.530825419406411,-0.461299557966116,
-0.0710999999999999));
#57022=CARTESIAN_POINT('Ctrl Pts',(-0.522604263717814,-0.471993563819338,
-0.0710999999999997));
#57023=CARTESIAN_POINT('Ctrl Pts',(-0.51522815102627,-0.481588345293528,
-0.0710999999999996));
#57024=CARTESIAN_POINT('Ctrl Pts',(-0.507593820692343,-0.491002935074771,
-0.0710999999999987));
#57025=CARTESIAN_POINT('Ctrl Pts',(-0.499731411497607,-0.500197640924792,
-0.0710999999999989));
#57026=CARTESIAN_POINT('Ctrl Pts',(-0.494876261095983,-0.505875503612279,
-0.071099999999999));
#57027=CARTESIAN_POINT('Ctrl Pts',(-0.489932967483916,-0.511471246370217,
-0.0710999999999986));
#57028=CARTESIAN_POINT('Ctrl Pts',(-0.484903330545617,-0.516982602993148,
-0.0710999999999987));
#57029=CARTESIAN_POINT('Ctrl Pts',(-0.461971240369799,-0.542111042405098,
-0.0710999999999992));
#57030=CARTESIAN_POINT('Ctrl Pts',(-0.437248134919206,-0.56548729539326,
-0.0710999999999999));
#57031=CARTESIAN_POINT('Ctrl Pts',(-0.410992239190816,-0.587010422199328,
-0.0711));
#57032=CARTESIAN_POINT('Ctrl Pts',(-0.39326243857021,-0.601544329210201,
-0.0711000000000001));
#57033=CARTESIAN_POINT('Ctrl Pts',(-0.374832581857655,-0.615232798615158,
-0.0711));
#57034=CARTESIAN_POINT('Ctrl Pts',(-0.35577134099474,-0.628036837492105,
-0.0711000000000001));
#57035=CARTESIAN_POINT('Ctrl Pts',(-0.341140666782019,-0.637864724499193,
-0.0711000000000001));
#57036=CARTESIAN_POINT('Ctrl Pts',(-0.326137824756979,-0.647171429838753,
-0.0711000000000004));
#57037=CARTESIAN_POINT('Ctrl Pts',(-0.310791231743006,-0.655936080266888,
-0.0711000000000005));
#57038=CARTESIAN_POINT('Ctrl Pts',(-0.302074038217026,-0.66091458943176,
-0.0711000000000006));
#57039=CARTESIAN_POINT('Ctrl Pts',(-0.293241255994626,-0.665720310855507,
-0.0711000000000007));
#57040=CARTESIAN_POINT('Ctrl Pts',(-0.284325627455792,-0.670335295097501,
-0.0711000000000006));
#57041=CARTESIAN_POINT('Ctrl Pts',(-0.252583677741976,-0.686765835816121,
-0.0711000000000003));
#57042=CARTESIAN_POINT('Ctrl Pts',(-0.219739495999929,-0.700816273313726,
-0.0710999999999988));
#57043=CARTESIAN_POINT('Ctrl Pts',(-0.186058445098527,-0.712362050184812,
-0.0710999999999991));
#57044=CARTESIAN_POINT('Ctrl Pts',(-0.156596236519901,-0.722461618852489,
-0.0710999999999993));
#57045=CARTESIAN_POINT('Ctrl Pts',(-0.126492499041445,-0.730644623003689,
-0.0711000000000014));
#57046=CARTESIAN_POINT('Ctrl Pts',(-0.0959372766721807,-0.736918016760253,
-0.0711000000000021));
#57047=CARTESIAN_POINT('Ctrl Pts',(-0.0782625200973073,-0.74054687948642,
-0.0711000000000024));
#57048=CARTESIAN_POINT('Ctrl Pts',(-0.060436391626456,-0.743536212012475,
-0.0711000000000009));
#57049=CARTESIAN_POINT('Ctrl Pts',(-0.0424941216358214,-0.745882575461859,
-0.0711000000000012));
#57050=CARTESIAN_POINT('Ctrl Pts',(-0.0318388515518829,-0.747275996488369,
-0.0711000000000013));
#57051=CARTESIAN_POINT('Ctrl Pts',(-0.0211364537413023,-0.748442901172957,
-0.0711000000000007));
#57052=CARTESIAN_POINT('Ctrl Pts',(-0.0104285730074772,-0.749379640043616,
-0.0711000000000007));
#57053=CARTESIAN_POINT('Ctrl Pts',(0.025356570627025,-0.752510169404919,
-0.0711000000000008));
#57054=CARTESIAN_POINT('Ctrl Pts',(0.0612586008151781,-0.753084251111668,
-0.0711000000000002));
#57055=CARTESIAN_POINT('Ctrl Pts',(0.0969927642975169,-0.751127525158457,
-0.0711000000000003));
#57056=CARTESIAN_POINT('Ctrl Pts',(0.125940091500207,-0.749542431766203,
-0.0711000000000004));
#57057=CARTESIAN_POINT('Ctrl Pts',(0.154778109260746,-0.746295712572856,
-0.0711000000000011));
#57058=CARTESIAN_POINT('Ctrl Pts',(0.183361235835868,-0.741376633595651,
-0.0711000000000012));
#57059=CARTESIAN_POINT('Ctrl Pts',(0.199996157954703,-0.738513808373675,
-0.0711000000000013));
#57060=CARTESIAN_POINT('Ctrl Pts',(0.216544799385339,-0.735084126475059,
-0.0711000000000006));
#57061=CARTESIAN_POINT('Ctrl Pts',(0.232983116072828,-0.731099822944309,
-0.0711000000000004));
#57062=CARTESIAN_POINT('Ctrl Pts',(0.241901902693802,-0.728938095943941,
-0.0711000000000003));
#57063=CARTESIAN_POINT('Ctrl Pts',(0.250788206317074,-0.726613058778705,
-0.0711000000000002));
#57064=CARTESIAN_POINT('Ctrl Pts',(0.259638114598271,-0.724126353932503,
-0.0711000000000001));
#57065=CARTESIAN_POINT('Ctrl Pts',(0.26675216273337,-0.722127402371474,
-0.0711));
#57066=CARTESIAN_POINT('Ctrl Pts',(0.273841886282841,-0.72002407427316,
-0.0711000000000008));
#57067=CARTESIAN_POINT('Ctrl Pts',(0.280892730142186,-0.717821495687171,
-0.0711000000000007));
#57068=CARTESIAN_POINT('Ctrl Pts',(0.315569759821888,-0.70698890819525,
-0.0711000000000003));
#57069=CARTESIAN_POINT('Ctrl Pts',(0.349386649818376,-0.693738011373514,
-0.0711000000000011));
#57070=CARTESIAN_POINT('Ctrl Pts',(0.382115560216981,-0.678233698777178,
-0.0711000000000009));
#57071=CARTESIAN_POINT('Ctrl Pts',(0.415111724192097,-0.662602783035725,
-0.0711000000000007));
#57072=CARTESIAN_POINT('Ctrl Pts',(0.447003233551593,-0.644681145485417,
-0.0711000000000005));
#57073=CARTESIAN_POINT('Ctrl Pts',(0.477547339957608,-0.624586406195176,
-0.0711000000000002));
#57074=CARTESIAN_POINT('Ctrl Pts',(0.496805372995163,-0.611916690211726,
-0.0711));
#57075=CARTESIAN_POINT('Ctrl Pts',(0.515527533576182,-0.598382096416591,
-0.0711000000000005));
#57076=CARTESIAN_POINT('Ctrl Pts',(0.533647856309012,-0.584002718706682,
-0.0711000000000004));
#57077=CARTESIAN_POINT('',(-0.7911,-9.68818082805471E-17,-0.0711000000000002));
#57078=CARTESIAN_POINT('Origin',(0.,0.,-0.0711000000000002));
#57079=CARTESIAN_POINT('',(0.789513386643969,0.0505148782186592,-0.0710999999999996));
#57080=CARTESIAN_POINT('Origin',(0.,0.,-0.0711000000000002));
#57081=CARTESIAN_POINT('Ctrl Pts',(0.78951338664397,0.0505148782186367,
-0.0711000000000005));
#57082=CARTESIAN_POINT('Ctrl Pts',(0.78661052546768,0.0722981214340736,
-0.0711000000000005));
#57083=CARTESIAN_POINT('Ctrl Pts',(0.782799122054415,0.093925916286846,
-0.0711000000000009));
#57084=CARTESIAN_POINT('Ctrl Pts',(0.778073401536598,0.115341501127996,
-0.0711000000000008));
#57085=CARTESIAN_POINT('Ctrl Pts',(0.771149681304201,0.146717778564259,
-0.0711000000000006));
#57086=CARTESIAN_POINT('Ctrl Pts',(0.762264400925658,0.177639384255821,
-0.0711000000000003));
#57087=CARTESIAN_POINT('Ctrl Pts',(0.751493831504571,0.20793557337634,-0.0711000000000002));
#57088=CARTESIAN_POINT('Ctrl Pts',(0.747066427308488,0.220389276573766,
-0.0711000000000002));
#57089=CARTESIAN_POINT('Ctrl Pts',(0.742320147977868,0.23273712772702,-0.0711000000000011));
#57090=CARTESIAN_POINT('Ctrl Pts',(0.737259077679951,0.244966403627896,
-0.0711000000000011));
#57091=CARTESIAN_POINT('Ctrl Pts',(0.733765772645089,0.253407422733052,
-0.0711000000000011));
#57092=CARTESIAN_POINT('Ctrl Pts',(0.730123916425295,0.261788183558137,
-0.0711000000000004));
#57093=CARTESIAN_POINT('Ctrl Pts',(0.726339264530682,0.270096071681808,
-0.0711000000000004));
#57094=CARTESIAN_POINT('Ctrl Pts',(0.710964767292107,0.303845437957103,
-0.0711000000000003));
#57095=CARTESIAN_POINT('Ctrl Pts',(0.693219611127889,0.336438260657923,
-0.0711000000000011));
#57096=CARTESIAN_POINT('Ctrl Pts',(0.673216664367045,0.36760422296276,-0.0711000000000007));
#57097=CARTESIAN_POINT('Ctrl Pts',(0.660742576029565,0.387039707722144,
-0.0711000000000005));
#57098=CARTESIAN_POINT('Ctrl Pts',(0.647389499046721,0.405919707003685,
-0.0711000000000008));
#57099=CARTESIAN_POINT('Ctrl Pts',(0.633176849541804,0.424170344891628,
-0.0711000000000008));
#57100=CARTESIAN_POINT('Ctrl Pts',(0.628311904428941,0.430417480696169,
-0.0711000000000008));
#57101=CARTESIAN_POINT('Ctrl Pts',(0.623352327566985,0.436582931045207,
-0.0711000000000015));
#57102=CARTESIAN_POINT('Ctrl Pts',(0.618299802221877,0.442663774988552,
-0.0711000000000014));
#57103=CARTESIAN_POINT('Ctrl Pts',(0.614443389962302,0.447305066131087,
-0.0711000000000014));
#57104=CARTESIAN_POINT('Ctrl Pts',(0.610532753409042,0.451897160166506,
-0.0711000000000004));
#57105=CARTESIAN_POINT('Ctrl Pts',(0.606568433677576,0.456438943152013,
-0.0711000000000004));
#57106=CARTESIAN_POINT('Ctrl Pts',(0.58313660419168,0.483283973746704,-0.0711000000000006));
#57107=CARTESIAN_POINT('Ctrl Pts',(0.557832078686923,0.508374602396631,
-0.0711000000000008));
#57108=CARTESIAN_POINT('Ctrl Pts',(0.530883792611114,0.531563679938661,
-0.0711000000000007));
#57109=CARTESIAN_POINT('Ctrl Pts',(0.504174176005348,0.554547381716453,
-0.0711000000000006));
#57110=CARTESIAN_POINT('Ctrl Pts',(0.475848664779934,0.575663628147837,
-0.0711000000000008));
#57111=CARTESIAN_POINT('Ctrl Pts',(0.446106434425362,0.594724507602636,
-0.071100000000001));
#57112=CARTESIAN_POINT('Ctrl Pts',(0.435751912723322,0.601360401670492,
-0.071100000000001));
#57113=CARTESIAN_POINT('Ctrl Pts',(0.425225545807383,0.607746741139793,
-0.0711000000000012));
#57114=CARTESIAN_POINT('Ctrl Pts',(0.414535431121882,0.613874117881312,
-0.0711000000000012));
#57115=CARTESIAN_POINT('Ctrl Pts',(0.408223415711616,0.617492048797379,
-0.0711000000000012));
#57116=CARTESIAN_POINT('Ctrl Pts',(0.401862277040809,0.621015092498111,
-0.0711000000000001));
#57117=CARTESIAN_POINT('Ctrl Pts',(0.395455743413018,0.624441054785095,
-0.0711000000000001));
#57118=CARTESIAN_POINT('Ctrl Pts',(0.365742774357445,0.640330382357987,
-0.0711));
#57119=CARTESIAN_POINT('Ctrl Pts',(0.3350422875416,0.654141967795412,-0.0711000000000001));
#57120=CARTESIAN_POINT('Ctrl Pts',(0.303539059002828,0.665732433051718,
-0.0710999999999999));
#57121=CARTESIAN_POINT('Ctrl Pts',(0.275530358755668,0.676037213931223,
-0.0710999999999998));
#57122=CARTESIAN_POINT('Ctrl Pts',(0.246886289233648,0.684585758484945,
-0.0710999999999995));
#57123=CARTESIAN_POINT('Ctrl Pts',(0.217777992627247,0.691347378539147,
-0.0710999999999995));
#57124=CARTESIAN_POINT('Ctrl Pts',(0.202137684730114,0.694980494587163,
-0.0710999999999995));
#57125=CARTESIAN_POINT('Ctrl Pts',(0.186363322806913,0.698097230410341,
-0.0710999999999994));
#57126=CARTESIAN_POINT('Ctrl Pts',(0.170481817352287,0.700689439048332,
-0.0710999999999994));
#57127=CARTESIAN_POINT('Ctrl Pts',(0.163380351267642,0.701848553452165,
-0.0710999999999993));
#57128=CARTESIAN_POINT('Ctrl Pts',(0.156257469551547,0.702902759038939,
-0.0710999999999998));
#57129=CARTESIAN_POINT('Ctrl Pts',(0.149115623612038,0.703851173059788,
-0.0710999999999999));
#57130=CARTESIAN_POINT('Ctrl Pts',(0.141353010569289,0.704882022942371,
-0.0710999999999999));
#57131=CARTESIAN_POINT('Ctrl Pts',(0.13357626627858,0.705786728185342,-0.0711000000000005));
#57132=CARTESIAN_POINT('Ctrl Pts',(0.12579468693895,0.706564431715505,-0.0711000000000005));
#57133=CARTESIAN_POINT('Ctrl Pts',(0.0920135096877081,0.709940576795407,
-0.0711000000000001));
#57134=CARTESIAN_POINT('Ctrl Pts',(0.058104255206695,0.710932267880054,
-0.0710999999999991));
#57135=CARTESIAN_POINT('Ctrl Pts',(0.0243216192917772,0.709505711937895,
-0.0710999999999992));
#57136=CARTESIAN_POINT('Ctrl Pts',(-0.000340213743341033,0.708464304614045,
-0.0710999999999992));
#57137=CARTESIAN_POINT('Ctrl Pts',(-0.0249347689083127,0.706133099639931,
-0.0711000000000011));
#57138=CARTESIAN_POINT('Ctrl Pts',(-0.0493592836677601,0.702481730021055,
-0.0711000000000013));
#57139=CARTESIAN_POINT('Ctrl Pts',(-0.0651808582794006,0.700116466373908,
-0.0711000000000014));
#57140=CARTESIAN_POINT('Ctrl Pts',(-0.0809309971795266,0.697196915910823,
-0.0710999999999999));
#57141=CARTESIAN_POINT('Ctrl Pts',(-0.0965819268706004,0.693730207786549,
-0.0710999999999999));
#57142=CARTESIAN_POINT('Ctrl Pts',(-0.104866815817021,0.691895090487693,
-0.0710999999999998));
#57143=CARTESIAN_POINT('Ctrl Pts',(-0.113123881048993,0.689906614697153,
-0.0711000000000002));
#57144=CARTESIAN_POINT('Ctrl Pts',(-0.121348819670347,0.687765605816627,
-0.0711000000000001));
#57145=CARTESIAN_POINT('Ctrl Pts',(-0.127458595159029,0.686175188649826,
-0.0711000000000001));
#57146=CARTESIAN_POINT('Ctrl Pts',(-0.133548886198576,0.684500970614239,
-0.0711000000000011));
#57147=CARTESIAN_POINT('Ctrl Pts',(-0.139609180249646,0.682746165691243,
-0.071100000000001));
#57148=CARTESIAN_POINT('Ctrl Pts',(-0.171636625378093,0.673472371728645,
-0.0711000000000007));
#57149=CARTESIAN_POINT('Ctrl Pts',(-0.202898352839185,0.661933786898764,
-0.0711000000000011));
#57150=CARTESIAN_POINT('Ctrl Pts',(-0.233159168168239,0.648235814607184,
-0.071100000000001));
#57151=CARTESIAN_POINT('Ctrl Pts',(-0.262858401786809,0.634792049964209,
-0.071100000000001));
#57152=CARTESIAN_POINT('Ctrl Pts',(-0.291594498854259,0.619267592208833,
-0.0711000000000003));
#57153=CARTESIAN_POINT('Ctrl Pts',(-0.319116683345441,0.601722036612944,
-0.0711000000000002));
#57154=CARTESIAN_POINT('Ctrl Pts',(-0.334495563251145,0.591917909601351,
-0.0711000000000001));
#57155=CARTESIAN_POINT('Ctrl Pts',(-0.349494822078873,0.58148206204072,
-0.0711000000000004));
#57156=CARTESIAN_POINT('Ctrl Pts',(-0.364065050236245,0.570420484551949,
-0.0711000000000004));
#57157=CARTESIAN_POINT('Ctrl Pts',(-0.292601934307099,0.610169646934149,
-3.87494887079529));
#57158=CARTESIAN_POINT('Ctrl Pts',(-0.393874364065824,0.561605269816615,
-3.86966574736363));
#57159=CARTESIAN_POINT('Ctrl Pts',(-0.57167140911708,0.413129829644052,
-3.85909950050031));
#57160=CARTESIAN_POINT('Ctrl Pts',(-0.699554853645959,0.0898747877851167,
-3.84325013020534));
#57161=CARTESIAN_POINT('Ctrl Pts',(-0.657542948589637,-0.255117175027513,
-3.82740075991035));
#57162=CARTESIAN_POINT('Ctrl Pts',(-0.455854483614461,-0.538198316628701,
-3.81155138961538));
#57163=CARTESIAN_POINT('Ctrl Pts',(-0.143460319648273,-0.690557636244561,
-3.79570201932039));
#57164=CARTESIAN_POINT('Ctrl Pts',(0.203771242261294,-0.675228509254,-3.77985264902541));
#57165=CARTESIAN_POINT('Ctrl Pts',(0.501518367203066,-0.495916548685635,
-3.76400327873043));
#57166=CARTESIAN_POINT('Ctrl Pts',(0.677472975891979,-0.19617577998387,
-3.74815390843546));
#57167=CARTESIAN_POINT('Ctrl Pts',(0.688905638980991,0.15120714934306,-3.73230453814047));
#57168=CARTESIAN_POINT('Ctrl Pts',(0.533039672552928,0.46186914013689,-3.71645516784549));
#57169=CARTESIAN_POINT('Ctrl Pts',(0.24772677985824,0.66036808055943,-3.70060579755051));
#57170=CARTESIAN_POINT('Ctrl Pts',(-0.097745794456612,0.698498547043651,
-3.68475642725553));
#57171=CARTESIAN_POINT('Ctrl Pts',(-0.419481102114336,0.567000979985795,
-3.66890705696055));
#57172=CARTESIAN_POINT('Ctrl Pts',(-0.639346774094541,0.297808988211044,
-3.65305768666557));
#57173=CARTESIAN_POINT('Ctrl Pts',(-0.703949125559012,-0.0437049361714047,
-3.63720831637059));
#57174=CARTESIAN_POINT('Ctrl Pts',(-0.597599687597092,-0.374605270350371,
-3.62135894607561));
#57175=CARTESIAN_POINT('Ctrl Pts',(-0.346125077999637,-0.614533907095192,
-3.60550957578063));
#57176=CARTESIAN_POINT('Ctrl Pts',(-0.0105951019105329,-0.705224955685239,
-3.58966020548565));
#57177=CARTESIAN_POINT('Ctrl Pts',(0.32750786099247,-0.624654379983339,
-3.57381083519067));
#57178=CARTESIAN_POINT('Ctrl Pts',(0.586076588355783,-0.392388489065435,
-3.55796146489568));
#57179=CARTESIAN_POINT('Ctrl Pts',(0.702318492816257,-0.0648323094657422,
-3.54211209460071));
#57180=CARTESIAN_POINT('Ctrl Pts',(0.648004599968331,0.278468188664054,
-3.52626272430573));
#57181=CARTESIAN_POINT('Ctrl Pts',(0.436324864834359,0.55414357890779,-3.51041335401075));
#57182=CARTESIAN_POINT('Ctrl Pts',(0.118685033304739,0.695246975223788,
-3.49456398371577));
#57183=CARTESIAN_POINT('Ctrl Pts',(-0.227777078549499,0.667511869700924,
-3.47871461342078));
#57184=CARTESIAN_POINT('Ctrl Pts',(-0.518924256183446,0.477673643863711,
-3.46286524312581));
#57185=CARTESIAN_POINT('Ctrl Pts',(-0.684052339708951,0.171833903051996,
-3.44701587283082));
#57186=CARTESIAN_POINT('Ctrl Pts',(-0.683060502755426,-0.175735150937388,
-3.43116650253584));
#57187=CARTESIAN_POINT('Ctrl Pts',(-0.51618960975049,-0.480627486193364,
-3.41531713224086));
#57188=CARTESIAN_POINT('Ctrl Pts',(-0.223963722768737,-0.6688009753155,
-3.39946776194589));
#57189=CARTESIAN_POINT('Ctrl Pts',(0.122651037193902,-0.694558288968156,
-3.3836183916509));
#57190=CARTESIAN_POINT('Ctrl Pts',(0.43948038548163,-0.551644346002168,
-3.36776902135592));
#57191=CARTESIAN_POINT('Ctrl Pts',(0.649583329296276,-0.274765339880352,
-3.35191965106094));
#57192=CARTESIAN_POINT('Ctrl Pts',(0.701937041446152,0.0688395492796521,
-3.33607028076596));
#57193=CARTESIAN_POINT('Ctrl Pts',(0.583827590563321,0.39572697430961,-3.32022091047098));
#57194=CARTESIAN_POINT('Ctrl Pts',(0.323937478628386,0.626513370678621,
-3.304371540176));
#57195=CARTESIAN_POINT('Ctrl Pts',(-0.0146198127989899,0.705153000967117,
-3.28852216988102));
#57196=CARTESIAN_POINT('Ctrl Pts',(-0.349626729498273,0.612548482750179,
-3.27267279958604));
#57197=CARTESIAN_POINT('Ctrl Pts',(-0.599727914383955,0.371188526772956,
-3.25682342929106));
#57198=CARTESIAN_POINT('Ctrl Pts',(-0.704187095487817,0.0396866255511638,
-3.24097405899607));
#57199=CARTESIAN_POINT('Ctrl Pts',(-0.637636695139234,-0.301453045615932,
-3.22512468870111));
#57200=CARTESIAN_POINT('Ctrl Pts',(-0.41623826497985,-0.56938580985635,
-3.20927531840611));
#57201=CARTESIAN_POINT('Ctrl Pts',(-0.0937577048939214,-0.699045053249238,
-3.19342594811114));
#57202=CARTESIAN_POINT('Ctrl Pts',(0.251491613629344,-0.658943443683383,
-3.17757657781615));
#57203=CARTESIAN_POINT('Ctrl Pts',(0.535666999015903,-0.458819528643346,
-3.16172720752118));
#57204=CARTESIAN_POINT('Ctrl Pts',(0.689757368805666,-0.147272760134018,
-3.1458778372262));
#57205=CARTESIAN_POINT('Ctrl Pts',(0.676342370066224,0.20003872663164,-3.13002846693121));
#57206=CARTESIAN_POINT('Ctrl Pts',(0.498679792288921,0.498771449124632,
-3.11417909663624));
#57207=CARTESIAN_POINT('Ctrl Pts',(0.199914423641749,0.676379122178673,
-3.09832972634125));
#57208=CARTESIAN_POINT('Ctrl Pts',(-0.147399522694991,0.689730291062018,
-3.08248035604627));
#57209=CARTESIAN_POINT('Ctrl Pts',(-0.458917966893342,0.535582667159503,
-3.0666309857513));
#57210=CARTESIAN_POINT('Ctrl Pts',(-0.658989652208569,0.251370507381504,
-3.05078161545631));
#57211=CARTESIAN_POINT('Ctrl Pts',(-0.699027810457228,-0.093886175268675,
-3.03493224516134));
#57212=CARTESIAN_POINT('Ctrl Pts',(-0.569309303103972,-0.416342900862349,
-3.01908287486635));
#57213=CARTESIAN_POINT('Ctrl Pts',(-0.301335854323042,-0.63769208604044,
-3.00323350457137));
#57214=CARTESIAN_POINT('Ctrl Pts',(0.0398160418543145,-0.704179789904724,
-2.98738413427639));
#57215=CARTESIAN_POINT('Ctrl Pts',(0.371298739751515,-0.599659686454028,
-2.97153476398141));
#57216=CARTESIAN_POINT('Ctrl Pts',(0.612612727535191,-0.349514148155837,
-2.95568539368643));
#57217=CARTESIAN_POINT('Ctrl Pts',(0.705155675918236,-0.0144902180625897,
-2.93983602339145));
#57218=CARTESIAN_POINT('Ctrl Pts',(0.62645382619254,0.324052615091952,-2.92398665309647));
#57219=CARTESIAN_POINT('Ctrl Pts',(0.39561967057411,0.583900308232526,-2.90813728280149));
#57220=CARTESIAN_POINT('Ctrl Pts',(0.0687105446633539,0.70194968106786,
-2.89228791250651));
#57221=CARTESIAN_POINT('Ctrl Pts',(-0.274884717019473,0.649532821378821,
-2.87643854221153));
#57222=CARTESIAN_POINT('Ctrl Pts',(-0.551725105308022,0.439378995711058,
-2.86058917191655));
#57223=CARTESIAN_POINT('Ctrl Pts',(-0.694580818302046,0.122523387751345,
-2.84473980162157));
#57224=CARTESIAN_POINT('Ctrl Pts',(-0.668759803500533,-0.22408663262483,
-2.82889043132659));
#57225=CARTESIAN_POINT('Ctrl Pts',(-0.48053261167355,-0.516277931755177,
-2.81304106103161));
#57226=CARTESIAN_POINT('Ctrl Pts',(-0.175609613684971,-0.683092788192513,
-2.79719169073663));
#57227=CARTESIAN_POINT('Ctrl Pts',(0.171959616715022,-0.684020748163701,
-2.78134232044165));
#57228=CARTESIAN_POINT('Ctrl Pts',(0.477769004781086,-0.518836459560908,
-2.76549295014667));
#57229=CARTESIAN_POINT('Ctrl Pts',(0.667553719770789,-0.227654397979453,
-2.74964357985169));
#57230=CARTESIAN_POINT('Ctrl Pts',(0.695225151307124,0.118812805240822,
-2.7337942095567));
#57231=CARTESIAN_POINT('Ctrl Pts',(0.55406338084068,0.436426699126669,-2.71794483926173));
#57232=CARTESIAN_POINT('Ctrl Pts',(0.278349092353365,0.648055766493336,
-2.70209546896675));
#57233=CARTESIAN_POINT('Ctrl Pts',(-0.0649613819857274,0.702306565930941,
-2.68624609867177));
#57234=CARTESIAN_POINT('Ctrl Pts',(-0.392496192704833,0.586004464497855,
-2.67039672837678));
#57235=CARTESIAN_POINT('Ctrl Pts',(-0.624714559731321,0.327393055147643,
-2.6545473580818));
#57236=CARTESIAN_POINT('Ctrl Pts',(-0.705222996156349,-0.0107247093885438,
-2.63869798778683));
#57237=CARTESIAN_POINT('Ctrl Pts',(-0.614470285968358,-0.346238012588408,
-2.62284861749184));
#57238=CARTESIAN_POINT('Ctrl Pts',(-0.374495434261829,-0.597668523026142,
-2.60699924719686));
#57239=CARTESIAN_POINT('Ctrl Pts',(-0.0435755654152151,-0.703957146279481,
-2.59114987690188));
#57240=CARTESIAN_POINT('Ctrl Pts',(0.29792648997097,-0.639292030509363,
-2.5753005066069));
#57241=CARTESIAN_POINT('Ctrl Pts',(0.567078051177426,-0.419376892033906,
-2.55945113631192));
#57242=CARTESIAN_POINT('Ctrl Pts',(0.698516523342481,-0.097617418101175,
-2.54360176601694));
#57243=CARTESIAN_POINT('Ctrl Pts',(0.660322494344382,0.247848133263131,
-2.52775239572196));
#57244=CARTESIAN_POINT('Ctrl Pts',(0.461771261834565,0.533124559031865,
-2.51190302542698));
#57245=CARTESIAN_POINT('Ctrl Pts',(0.151080356900915,0.688933392613464,
-2.496053655132));
#57246=CARTESIAN_POINT('Ctrl Pts',(-0.196299928972631,0.67743695764591,
-2.48020428483702));
#57247=CARTESIAN_POINT('Ctrl Pts',(-0.496009405614011,0.501427126551448,
-2.46435491454204));
#57248=CARTESIAN_POINT('Ctrl Pts',(-0.675264586239405,0.203647323257959,
-2.44850554424706));
#57249=CARTESIAN_POINT('Ctrl Pts',(-0.690533924178398,-0.143587580444789,
-2.43265617395207));
#57250=CARTESIAN_POINT('Ctrl Pts',(-0.538109309602317,-0.455952699979421,
-2.4168068036571));
#57251=CARTESIAN_POINT('Ctrl Pts',(-0.255006572123388,-0.657591166206698,
-2.40095743336211));
#57252=CARTESIAN_POINT('Ctrl Pts',(0.0900236949082282,-0.699535723215246,
-2.38510806306714));
#57253=CARTESIAN_POINT('Ctrl Pts',(0.413191995871872,-0.571600269634842,
-2.36925869277215));
#57254=CARTESIAN_POINT('Ctrl Pts',(0.63601794360821,-0.304853520740027,
-2.35340932247718));
#57255=CARTESIAN_POINT('Ctrl Pts',(0.704388970160089,0.0359259295776118,
-2.33755995218219));
#57256=CARTESIAN_POINT('Ctrl Pts',(0.601701390641733,0.367980882926015,
-2.32171058188722));
#57257=CARTESIAN_POINT('Ctrl Pts',(0.352892554951089,0.610672857067759,
-2.30586121159223));
#57258=CARTESIAN_POINT('Ctrl Pts',(0.0183848921922413,0.705064883140754,
-2.29001184129726));
#57259=CARTESIAN_POINT('Ctrl Pts',(-0.320587482770208,0.628234159840316,
-2.27416247100227));
#57260=CARTESIAN_POINT('Ctrl Pts',(-0.581706214008261,0.398838782321105,
-2.2583131007073));
#57261=CARTESIAN_POINT('Ctrl Pts',(-0.701559453698322,0.0725866835288543,
-2.24246373041231));
#57262=CARTESIAN_POINT('Ctrl Pts',(-0.651041226331259,-0.271292858948218,
-2.22661436011734));
#57263=CARTESIAN_POINT('Ctrl Pts',(-0.442419721672428,-0.549289799263099,
-2.21076498982235));
#57264=CARTESIAN_POINT('Ctrl Pts',(-0.126358004157817,-0.693893470559033,
-2.19491561952737));
#57265=CARTESIAN_POINT('Ctrl Pts',(0.220389350089783,-0.669987334258051,
-2.17906624923239));
#57266=CARTESIAN_POINT('Ctrl Pts',(0.513615856317125,-0.483376919017481,
-2.16321687893741));
#57267=CARTESIAN_POINT('Ctrl Pts',(0.682112396348077,-0.179379966683827,
-2.14736750864243));
#57268=CARTESIAN_POINT('Ctrl Pts',(0.684960124933254,0.168178836214988,
-2.13151813834745));
#57269=CARTESIAN_POINT('Ctrl Pts',(0.521467480303687,0.474895947218893,
-2.11566876805247));
#57270=CARTESIAN_POINT('Ctrl Pts',(0.231338127732153,0.666286097976378,
-2.09981939775749));
#57271=CARTESIAN_POINT('Ctrl Pts',(-0.114970948453971,0.695870803174554,
-2.08397002746251));
#57272=CARTESIAN_POINT('Ctrl Pts',(-0.433359697925381,0.556465511881219,
-2.06812065716753));
#57273=CARTESIAN_POINT('Ctrl Pts',(-0.646508432299333,0.28192435273503,
-2.05227128687255));
#57274=CARTESIAN_POINT('Ctrl Pts',(-0.702654663898939,-0.0610812327992534,
-2.03642191657757));
#57275=CARTESIAN_POINT('Ctrl Pts',(-0.588163460150873,-0.38925343651991,
-2.02057254628259));
#57276=CARTESIAN_POINT('Ctrl Pts',(-0.330838643304082,-0.622896689504703,
-2.00472317598761));
#57277=CARTESIAN_POINT('Ctrl Pts',(0.00682927878028947,-0.705271475852064,
-1.98887380569263));
#57278=CARTESIAN_POINT('Ctrl Pts',(0.342838732379053,-0.616373342447522,
-1.97302443539765));
#57279=CARTESIAN_POINT('Ctrl Pts',(0.59559089753061,-0.377790916351739,
-1.95717506510267));
#57280=CARTESIAN_POINT('Ctrl Pts',(0.703705720197163,-0.0474631758419071,
-1.94132569480769));
#57281=CARTESIAN_POINT('Ctrl Pts',(0.640927861859323,0.294390844952153,
-1.92547632451271));
#57282=CARTESIAN_POINT('Ctrl Pts',(0.422502724410463,0.56475299163877,-1.90962695421772));
#57283=CARTESIAN_POINT('Ctrl Pts',(0.101474153120063,0.697966682548511,
-1.89377758392275));
#57284=CARTESIAN_POINT('Ctrl Pts',(-0.244197091352646,0.661681399371415,
-1.87792821362777));
#57285=CARTESIAN_POINT('Ctrl Pts',(-0.53056585406773,0.464708906947766,
-1.86207884333278));
#57286=CARTESIAN_POINT('Ctrl Pts',(-0.688088397903683,0.154883344390378,
-1.8462294730378));
#57287=CARTESIAN_POINT('Ctrl Pts',(-0.678510877450221,-0.192555142442203,
-1.83038010274283));
#57288=CARTESIAN_POINT('Ctrl Pts',(-0.504159162883881,-0.493232229461368,
-1.81453073244784));
#57289=CARTESIAN_POINT('Ctrl Pts',(-0.207374009842694,-0.67412944880117,
-1.79868136215287));
#57290=CARTESIAN_POINT('Ctrl Pts',(0.139771257512638,-0.691316489946928,
-1.78283199185788));
#57291=CARTESIAN_POINT('Ctrl Pts',(0.45297352250471,-0.540619534986371,
-1.7669826215629));
#57292=CARTESIAN_POINT('Ctrl Pts',(0.656172617900346,-0.258634856925766,
-1.75113325126792));
#57293=CARTESIAN_POINT('Ctrl Pts',(0.700022293991506,0.0861584680346388,
-1.73528388097294));
#57294=CARTESIAN_POINT('Ctrl Pts',(0.573873797338617,0.410028484897529,
-1.71943451067796));
#57295=CARTESIAN_POINT('Ctrl Pts',(0.308361886447897,0.634324397044211,
-1.70358514038298));
#57296=CARTESIAN_POINT('Ctrl Pts',(-0.0320347212446137,0.704576660367049,
-1.687735770088));
#57297=CARTESIAN_POINT('Ctrl Pts',(-0.364651799452575,0.603724737653847,
-1.67188639979302));
#57298=CARTESIAN_POINT('Ctrl Pts',(-0.608714355716241,0.356260195424872,
-1.65603702949804));
#57299=CARTESIAN_POINT('Ctrl Pts',(-0.704952579693588,0.0222790054212492,
-1.64018765920306));
#57300=CARTESIAN_POINT('Ctrl Pts',(-0.629995326830073,-0.317112569715355,
-1.62433828890808));
#57301=CARTESIAN_POINT('Ctrl Pts',(-0.402045725983278,-0.579494372636858,
-1.6084889186131));
#57302=CARTESIAN_POINT('Ctrl Pts',(-0.0764606078631723,-0.701147822605475,
-1.59263954831812));
#57303=CARTESIAN_POINT('Ctrl Pts',(0.267692724062702,-0.652529768809897,
-1.57679017802314));
#57304=CARTESIAN_POINT('Ctrl Pts',(0.54683773505632,-0.445446949947669,
-1.56094080772816));
#57305=CARTESIAN_POINT('Ctrl Pts',(0.693184952972512,-0.130188765535679,
-1.54509143743318));
#57306=CARTESIAN_POINT('Ctrl Pts',(0.671194424519117,0.216685343744462,
-1.5292420671382));
#57307=CARTESIAN_POINT('Ctrl Pts',(0.486206479121138,0.510938111085708,
-1.51339269684322));
#57308=CARTESIAN_POINT('Ctrl Pts',(0.183144847018672,0.681111194086335,
-1.49754332654823));
#57309=CARTESIAN_POINT('Ctrl Pts',(-0.16439292478377,0.685878604404777,
-1.48169395625326));
#57310=CARTESIAN_POINT('Ctrl Pts',(-0.472008401160537,0.524082591709629,
-1.46584458595827));
#57311=CARTESIAN_POINT('Ctrl Pts',(-0.664998148605724,0.235014799640717,
-1.4499952156633));
#57312=CARTESIAN_POINT('Ctrl Pts',(-0.696495224872468,-0.111125584043703,
-1.43414584536831));
#57313=CARTESIAN_POINT('Ctrl Pts',(-0.558850665837655,-0.430279475448245,
-1.41829647507333));
#57314=CARTESIAN_POINT('Ctrl Pts',(-0.285491011948519,-0.64494137392155,
-1.40244710477835));
#57315=CARTESIAN_POINT('Ctrl Pts',(0.0571992200988665,-0.7029813247301,
-1.38659773448337));
#57316=CARTESIAN_POINT('Ctrl Pts',(0.385998804687375,-0.590304511654048,
-1.37074836418839));
#57317=CARTESIAN_POINT('Ctrl Pts',(0.62105981545978,-0.334274137977006,
-1.35489899389341));
#57318=CARTESIAN_POINT('Ctrl Pts',(0.705298438575201,0.00293363981907094,
-1.33904962359843));
#57319=CARTESIAN_POINT('Ctrl Pts',(0.618257594127741,0.339428992578101,
-1.32320025330345));
#57320=CARTESIAN_POINT('Ctrl Pts',(0.381074872501545,0.593495101283185,
-1.30735088300847));
#57321=CARTESIAN_POINT('Ctrl Pts',(0.0513493382249849,0.703432824911564,
-1.29150151271349));
#57322=CARTESIAN_POINT('Ctrl Pts',(-0.290846218427701,0.642544139281894,
-1.27565214241851));
#57323=CARTESIAN_POINT('Ctrl Pts',(-0.562410702175123,0.425615666744179,
-1.25980277212353));
#57324=CARTESIAN_POINT('Ctrl Pts',(-0.6973955476423,0.105327792286287,-1.24395340182855));
#57325=CARTESIAN_POINT('Ctrl Pts',(-0.66302011730594,-0.240538599286731,
-1.22810403153357));
#57326=CARTESIAN_POINT('Ctrl Pts',(-0.467632374358977,-0.527990962186469,
-1.21225466123859));
#57327=CARTESIAN_POINT('Ctrl Pts',(-0.158681606577905,-0.687222410456076,
-1.19640529094361));
#57328=CARTESIAN_POINT('Ctrl Pts',(0.188804481289216,-0.679564096715178,
-1.18055592064863));
#57329=CARTESIAN_POINT('Ctrl Pts',(0.490440005394944,-0.506875817935137,
-1.16470655035365));
#57330=CARTESIAN_POINT('Ctrl Pts',(0.67297374449562,-0.211094369699316,
-1.14885718005867));
#57331=CARTESIAN_POINT('Ctrl Pts',(0.692077964492487,0.135950670329878,
-1.13300780976369));
#57332=CARTESIAN_POINT('Ctrl Pts',(0.543113266727756,0.449980525360276,
-1.1171584394687));
#57333=CARTESIAN_POINT('Ctrl Pts',(0.262255251094087,0.654734050567698,
-1.10130906917373));
#57334=CARTESIAN_POINT('Ctrl Pts',(-0.0822906125712717,0.700487507941325,
-1.08545969887874));
#57335=CARTESIAN_POINT('Ctrl Pts',(-0.406852464454183,0.576129816852735,
-1.06961032858376));
#57336=CARTESIAN_POINT('Ctrl Pts',(-0.63261149801648,0.311860844410696,
-1.05376095828879));
#57337=CARTESIAN_POINT('Ctrl Pts',(-0.704742854799411,-0.0281425355713375,
-1.0379115879938));
#57338=CARTESIAN_POINT('Ctrl Pts',(-0.605729665760521,-0.361311590897459,
-1.02206221769882));
#57339=CARTESIAN_POINT('Ctrl Pts',(-0.359616966834596,-0.606737283232118,
-1.00621284740384));
#57340=CARTESIAN_POINT('Ctrl Pts',(-0.0261724389449761,-0.704818769002982,
-0.990363477108863));
#57341=CARTESIAN_POINT('Ctrl Pts',(0.313627981942751,-0.631737273430753,
-0.974514106813883));
#57342=CARTESIAN_POINT('Ctrl Pts',(0.5772648515989,-0.405240403720689,-0.958664736518902));
#57343=CARTESIAN_POINT('Ctrl Pts',(0.700714800347687,-0.0803321994775939,
-0.942815366223922));
#57344=CARTESIAN_POINT('Ctrl Pts',(0.653998403401114,0.264084422198656,
-0.926965995928941));
#57345=CARTESIAN_POINT('Ctrl Pts',(0.44846058817974,0.544368987497165,-0.911116625633962));
#57346=CARTESIAN_POINT('Ctrl Pts',(0.134015555013097,0.692455287158485,
-0.89526725533898));
#57347=CARTESIAN_POINT('Ctrl Pts',(-0.212974726593566,0.672381037456889,
-0.879417885044001));
#57348=CARTESIAN_POINT('Ctrl Pts',(-0.508244777755666,0.489021205658097,
-0.86356851474902));
#57349=CARTESIAN_POINT('Ctrl Pts',(-0.680089211952753,0.186904139827591,
-0.847719144454039));
#57350=CARTESIAN_POINT('Ctrl Pts',(-0.686776158556577,-0.160601997924922,
-0.831869774159059));
#57351=CARTESIAN_POINT('Ctrl Pts',(-0.526681713994867,-0.469106454701526,
-0.816020403864078));
#57352=CARTESIAN_POINT('Ctrl Pts',(-0.23868430153437,-0.66368991095259,
-0.800171033569099));
#57353=CARTESIAN_POINT('Ctrl Pts',(0.107276829327393,-0.697098397350523,
-0.784321663274117));
#57354=CARTESIAN_POINT('Ctrl Pts',(0.427186125669077,-0.561218769941854,
-0.768472292979137));
#57355=CARTESIAN_POINT('Ctrl Pts',(0.643354639169021,-0.289048961179428,
-0.752622922684157));
#57356=CARTESIAN_POINT('Ctrl Pts',(0.703286538458407,0.0533154623200356,
-0.736773552389177));
#57357=CARTESIAN_POINT('Ctrl Pts',(0.592427553686509,0.38273239650208,-0.720924182094196));
#57358=CARTESIAN_POINT('Ctrl Pts',(0.337699434353656,0.619203993637335,
-0.705074811799215));
#57359=CARTESIAN_POINT('Ctrl Pts',(0.00096208864391743,0.705303883503167,
-0.689225441504236));
#57360=CARTESIAN_POINT('Ctrl Pts',(-0.336008897212553,0.620122983522791,
-0.673376071209255));
#57361=CARTESIAN_POINT('Ctrl Pts',(-0.591381198224044,0.384347202521759,
-0.657526700914275));
#57362=CARTESIAN_POINT('Ctrl Pts',(-0.703138468748386,0.0552339340023888,
-0.641677330619294));
#57363=CARTESIAN_POINT('Ctrl Pts',(-0.644140813466435,-0.287292718539838,
-0.625827960324315));
#57364=CARTESIAN_POINT('Ctrl Pts',(-0.42871562406298,-0.560051254246869,
-0.609978590029332));
#57365=CARTESIAN_POINT('Ctrl Pts',(-0.109178218030051,-0.69680313604847,
-0.594129219734354));
#57366=CARTESIAN_POINT('Ctrl Pts',(0.236872768681544,-0.664338607305327,
-0.578279849439372));
#57367=CARTESIAN_POINT('Ctrl Pts',(0.525399961944826,-0.470541574876744,
-0.562430479144392));
#57368=CARTESIAN_POINT('Ctrl Pts',(0.686335456690993,-0.162475027583201,
-0.546581108849412));
#57369=CARTESIAN_POINT('Ctrl Pts',(0.680596583308102,0.185048059941882,
-0.530731738554432));
#57370=CARTESIAN_POINT('Ctrl Pts',(0.509577008823849,0.487632818601885,
-0.514882368259451));
#57371=CARTESIAN_POINT('Ctrl Pts',(0.214808289323237,0.67179750858231,-0.499032997964472));
#57372=CARTESIAN_POINT('Ctrl Pts',(-0.132125935456141,0.692818324582584,
-0.48318362766949));
#57373=CARTESIAN_POINT('Ctrl Pts',(-0.446973799862388,0.545590428747379,
-0.46733425737451));
#57374=CARTESIAN_POINT('Ctrl Pts',(-0.653275508090676,0.265867644171376,
-0.451484887079529));
#57375=CARTESIAN_POINT('Ctrl Pts',(-0.700931350885312,-0.0784202465154788,
-0.43563551678455));
#57376=CARTESIAN_POINT('Ctrl Pts',(-0.57836825932194,-0.40366403145049,
-0.419786146489569));
#57377=CARTESIAN_POINT('Ctrl Pts',(-0.315350287932037,-0.63087929875971,
-0.403936776194589));
#57378=CARTESIAN_POINT('Ctrl Pts',(0.0242494914065197,-0.704887548433319,
-0.388087405899608));
#57379=CARTESIAN_POINT('Ctrl Pts',(0.357960358964906,-0.607716113702729,
-0.372238035604628));
#57380=CARTESIAN_POINT('Ctrl Pts',(0.604741700327879,-0.362962766947641,
-0.356388665309647));
#57381=CARTESIAN_POINT('Ctrl Pts',(0.704663454379142,-0.030065073630256,
-0.340539295014667));
#57382=CARTESIAN_POINT('Ctrl Pts',(0.633459948009497,0.310133825079147,
-0.324689924719686));
#57383=CARTESIAN_POINT('Ctrl Pts',(0.408422715107778,0.575017720253068,
-0.308840554424706));
#57384=CARTESIAN_POINT('Ctrl Pts',(0.0842013460493761,0.700260397514991,
-0.292991184129726));
#57385=CARTESIAN_POINT('Ctrl Pts',(-0.260468074786106,0.655447090429983,
-0.277141813834745));
#57386=CARTESIAN_POINT('Ctrl Pts',(-0.541883609692458,0.451460534380044,
-0.261292443539765));
#57387=CARTESIAN_POINT('Ctrl Pts',(-0.691704538864457,0.137838275507889,
-0.245443073244785));
#57388=CARTESIAN_POINT('Ctrl Pts',(-0.6735470517312,-0.209257650350784,
-0.229593702949804));
#57389=CARTESIAN_POINT('Ctrl Pts',(-0.491821179438923,-0.505535863107229,
-0.213744332654824));
#57390=CARTESIAN_POINT('Ctrl Pts',(-0.190657404081973,-0.679046628726581,
-0.197894962359843));
#57391=CARTESIAN_POINT('Ctrl Pts',(0.156805532386105,-0.687652471031271,
-0.182045592064863));
#57392=CARTESIAN_POINT('Ctrl Pts',(0.466191447257558,-0.529265333633324,
-0.166196221769883));
#57393=CARTESIAN_POINT('Ctrl Pts',(0.662358975760562,-0.242345413653074,
-0.150346851474902));
#57394=CARTESIAN_POINT('Ctrl Pts',(0.697685099148249,0.103422631371823,
-0.134497481179922));
#57395=CARTESIAN_POINT('Ctrl Pts',(0.563560339571208,0.424084008064863,
-0.118648110884941));
#57396=CARTESIAN_POINT('Ctrl Pts',(0.292616745553076,0.64173975329643,-0.102798740589961));
#57397=CARTESIAN_POINT('Ctrl Pts',(-0.0494690429576347,0.703588850062655,
-0.0869493702949807));
#57398=CARTESIAN_POINT('Ctrl Pts',(-0.269389956604521,0.630845896423734,
-0.0763831234316606));
#57399=CARTESIAN_POINT('Ctrl Pts',(-0.364065050236245,0.570420484551949,
-0.0711000000000004));
#57400=CARTESIAN_POINT('Ctrl Pts',(-0.309090610374644,0.644553868208604,
-3.8529325805302));
#57401=CARTESIAN_POINT('Ctrl Pts',(-0.416069934357496,0.593252795981349,
-3.84764945709854));
#57402=CARTESIAN_POINT('Ctrl Pts',(-0.60388618139578,0.436410482080527,
-3.83708321023521));
#57403=CARTESIAN_POINT('Ctrl Pts',(-0.738976101494388,0.0949394031846672,
-3.82123383994024));
#57404=CARTESIAN_POINT('Ctrl Pts',(-0.694596745603902,-0.269493513544402,
-3.80538446964525));
#57405=CARTESIAN_POINT('Ctrl Pts',(-0.481542751643377,-0.56852681641803,
-3.78953509935028));
#57406=CARTESIAN_POINT('Ctrl Pts',(-0.151544581786972,-0.729471873763095,
-3.77368572905529));
#57407=CARTESIAN_POINT('Ctrl Pts',(0.215254139712002,-0.713278921282305,
-3.75783635876032));
#57408=CARTESIAN_POINT('Ctrl Pts',(0.529779882009245,-0.523862390353358,
-3.74198698846533));
#57409=CARTESIAN_POINT('Ctrl Pts',(0.715649867888453,-0.207230658674656,
-3.72613761817036));
#57410=CARTESIAN_POINT('Ctrl Pts',(0.727726783308574,0.159727960083829,
-3.71028824787537));
#57411=CARTESIAN_POINT('Ctrl Pts',(0.563077472927324,0.487896345511823,
-3.69443887758039));
#57412=CARTESIAN_POINT('Ctrl Pts',(0.261686655537168,0.697581079138808,
-3.67858950728541));
#57413=CARTESIAN_POINT('Ctrl Pts',(-0.103253956067285,0.737860270003995,
-3.66274013699043));
#57414=CARTESIAN_POINT('Ctrl Pts',(-0.443119660846356,0.59895256469117,
-3.64689076669546));
#57415=CARTESIAN_POINT('Ctrl Pts',(-0.675375182033268,0.31459109167952,
-3.63104139640047));
#57416=CARTESIAN_POINT('Ctrl Pts',(-0.743617998995764,-0.0461677925321744,
-3.6151920261055));
#57417=CARTESIAN_POINT('Ctrl Pts',(-0.631275567731624,-0.395714990525769,
-3.5993426558105));
#57418=CARTESIAN_POINT('Ctrl Pts',(-0.365629885114147,-0.649164062738602,
-3.58349328551553));
#57419=CARTESIAN_POINT('Ctrl Pts',(-0.0111921560746506,-0.74496572457859,
-3.56764391522055));
#57420=CARTESIAN_POINT('Ctrl Pts',(0.345963552484283,-0.659854843541832,
-3.55179454492557));
#57421=CARTESIAN_POINT('Ctrl Pts',(0.619103119909842,-0.414500327471964,
-3.53594517463059));
#57422=CARTESIAN_POINT('Ctrl Pts',(0.741895476993479,-0.0684857335349459,
-3.52009580433561));
#57423=CARTESIAN_POINT('Ctrl Pts',(0.684520892878228,0.294160401256122,
-3.50424643404063));
#57424=CARTESIAN_POINT('Ctrl Pts',(0.460912601663608,0.585370624583888,
-3.48839706374565));
#57425=CARTESIAN_POINT('Ctrl Pts',(0.125373160889622,0.734425465921584,
-3.47254769345066));
#57426=CARTESIAN_POINT('Ctrl Pts',(-0.24061275057849,0.705127434399112,
-3.45669832315569));
#57427=CARTESIAN_POINT('Ctrl Pts',(-0.548166625971821,0.504591463113016,
-3.44084895286071));
#57428=CARTESIAN_POINT('Ctrl Pts',(-0.722599991382613,0.181517070634459,
-3.42499958256572));
#57429=CARTESIAN_POINT('Ctrl Pts',(-0.721552262528453,-0.185638161265563,
-3.40915021227075));
#57430=CARTESIAN_POINT('Ctrl Pts',(-0.545277877006026,-0.507711760081603,
-3.39330084197576));
#57431=CARTESIAN_POINT('Ctrl Pts',(-0.236584504939444,-0.706489183569325,
-3.37745147168079));
#57432=CARTESIAN_POINT('Ctrl Pts',(0.129562656648595,-0.733697970884298,
-3.3616021013858));
#57433=CARTESIAN_POINT('Ctrl Pts',(0.464245941906974,-0.582730555145881,
-3.34575273109082));
#57434=CARTESIAN_POINT('Ctrl Pts',(0.686188586609458,-0.290248889893811,
-3.32990336079585));
#57435=CARTESIAN_POINT('Ctrl Pts',(0.741492530112445,0.0727187889415322,
-3.31405399050086));
#57436=CARTESIAN_POINT('Ctrl Pts',(0.616727386810033,0.418026942715604,
-3.29820462020588));
#57437=CARTESIAN_POINT('Ctrl Pts',(0.342191972276529,0.661818591902024,
-3.2823552499109));
#57438=CARTESIAN_POINT('Ctrl Pts',(-0.015443667084096,0.74488971507511,
-3.26650587961592));
#57439=CARTESIAN_POINT('Ctrl Pts',(-0.369328861341332,0.647066755951808,
-3.25065650932095));
#57440=CARTESIAN_POINT('Ctrl Pts',(-0.633523724149739,0.392105706942817,
-3.23480713902596));
#57441=CARTESIAN_POINT('Ctrl Pts',(-0.743869378983116,0.041923042458244,
-3.21895776873098));
#57442=CARTESIAN_POINT('Ctrl Pts',(-0.673568736873105,-0.318440498656892,
-3.203108398436));
#57443=CARTESIAN_POINT('Ctrl Pts',(-0.439694083665483,-0.601471784265275,
-3.18725902814102));
#57444=CARTESIAN_POINT('Ctrl Pts',(-0.0990411300650332,-0.73843757287473,
-3.17140965784604));
#57445=CARTESIAN_POINT('Ctrl Pts',(0.265663644858933,-0.696076161262508,
-3.15556028755106));
#57446=CARTESIAN_POINT('Ctrl Pts',(0.565852854238509,-0.484674882604632,
-3.13971091725608));
#57447=CARTESIAN_POINT('Ctrl Pts',(0.728626509730431,-0.155571860552392,
-3.1238615469611));
#57448=CARTESIAN_POINT('Ctrl Pts',(0.714455550271918,0.211311289720478,
-3.10801217666611));
#57449=CARTESIAN_POINT('Ctrl Pts',(0.526781347994482,0.526878169867379,
-3.09216280637114));
#57450=CARTESIAN_POINT('Ctrl Pts',(0.211179982020463,0.714494373435872,
-3.07631343607615));
#57451=CARTESIAN_POINT('Ctrl Pts',(-0.155705766425003,0.728597906104378,
-3.06046406578118));
#57452=CARTESIAN_POINT('Ctrl Pts',(-0.48477886803742,0.565763770121453,
-3.04461469548619));
#57453=CARTESIAN_POINT('Ctrl Pts',(-0.696124973726058,0.265535714043468,
-3.02876532519122));
#57454=CARTESIAN_POINT('Ctrl Pts',(-0.738419358418565,-0.0991768399899824,
-3.01291595489623));
#57455=CARTESIAN_POINT('Ctrl Pts',(-0.60139096621175,-0.439804615979164,
-2.99706658460126));
#57456=CARTESIAN_POINT('Ctrl Pts',(-0.318316703411543,-0.673627249157046,
-2.98121721430627));
#57457=CARTESIAN_POINT('Ctrl Pts',(0.0420597516164567,-0.743861661716508,
-2.9653678440113));
#57458=CARTESIAN_POINT('Ctrl Pts',(0.392222130632537,-0.633451651446071,
-2.94951847371631));
#57459=CARTESIAN_POINT('Ctrl Pts',(0.647134621052763,-0.36920993582592,
-2.93366910342134));
#57460=CARTESIAN_POINT('Ctrl Pts',(0.744892540764818,-0.0153067694375815,
-2.91781973312635));
#57461=CARTESIAN_POINT('Ctrl Pts',(0.661755691970793,0.342313596899012,
-2.90197036283138));
#57462=CARTESIAN_POINT('Ctrl Pts',(0.417913592210328,0.616804202258335,
-2.88612099253639));
#57463=CARTESIAN_POINT('Ctrl Pts',(0.0725825146695105,0.7415058820009,-2.87027162224141));
#57464=CARTESIAN_POINT('Ctrl Pts',(-0.290374994161988,0.686135232474697,
-2.85442225194643));
#57465=CARTESIAN_POINT('Ctrl Pts',(-0.582815865392368,0.464138838629808,
-2.83857288165145));
#57466=CARTESIAN_POINT('Ctrl Pts',(-0.733721769789043,0.129427813916935,
-2.82272351135647));
#57467=CARTESIAN_POINT('Ctrl Pts',(-0.706445691644203,-0.23671434099992,
-2.80687414106149));
#57468=CARTESIAN_POINT('Ctrl Pts',(-0.507611539201978,-0.545371176123821,
-2.79102477076651));
#57469=CARTESIAN_POINT('Ctrl Pts',(-0.185505549749978,-0.721586367311385,
-2.77517540047153));
#57470=CARTESIAN_POINT('Ctrl Pts',(0.181649868501726,-0.722566619593644,
-2.75932603017655));
#57471=CARTESIAN_POINT('Ctrl Pts',(0.504692197799631,-0.548073881842458,
-2.74347665988157));
#57472=CARTESIAN_POINT('Ctrl Pts',(0.705171642800086,-0.240483156724765,
-2.72762728958659));
#57473=CARTESIAN_POINT('Ctrl Pts',(0.734402412185669,0.125508133017552,
-2.71177791929161));
#57474=CARTESIAN_POINT('Ctrl Pts',(0.585285907203018,0.46102017451216,-2.69592854899663));
#57475=CARTESIAN_POINT('Ctrl Pts',(0.294034593641594,0.684574942734325,
-2.68007917870165));
#57476=CARTESIAN_POINT('Ctrl Pts',(-0.068622079537157,0.741882878005469,
-2.66422980840666));
#57477=CARTESIAN_POINT('Ctrl Pts',(-0.414614100416485,0.619026931735213,
-2.64838043811169));
#57478=CARTESIAN_POINT('Ctrl Pts',(-0.659918414533182,0.345842277111536,
-2.6325310678167));
#57479=CARTESIAN_POINT('Ctrl Pts',(-0.744963654626517,-0.0113290671807901,
-2.61668169752173));
#57480=CARTESIAN_POINT('Ctrl Pts',(-0.649096856440149,-0.365749183781997,
-2.60083232722674));
#57481=CARTESIAN_POINT('Ctrl Pts',(-0.395598964964535,-0.631348282168147,
-2.58498295693176));
#57482=CARTESIAN_POINT('Ctrl Pts',(-0.0460311314875812,-0.743626471699101,
-2.56913358663678));
#57483=CARTESIAN_POINT('Ctrl Pts',(0.314715214887314,-0.675317353542847,
-2.5532842163418));
#57484=CARTESIAN_POINT('Ctrl Pts',(0.599033978991175,-0.443009578329501,
-2.53743484604682));
#57485=CARTESIAN_POINT('Ctrl Pts',(0.737879259301487,-0.10311834545982,
-2.52158547575185));
#57486=CARTESIAN_POINT('Ctrl Pts',(0.697532924053757,0.261814847437454,
-2.50573610545686));
#57487=CARTESIAN_POINT('Ctrl Pts',(0.487792951580825,0.563167142920953,
-2.48988673516189));
#57488=CARTESIAN_POINT('Ctrl Pts',(0.159594022646185,0.727756100911073,
-2.4740373648669));
#57489=CARTESIAN_POINT('Ctrl Pts',(-0.207361803695285,0.715611819945646,
-2.45818799457192));
#57490=CARTESIAN_POINT('Ctrl Pts',(-0.523960479946426,0.529683499773207,
-2.44233862427694));
#57491=CARTESIAN_POINT('Ctrl Pts',(-0.713317031274519,0.215123237636915,
-2.42648925398196));
#57492=CARTESIAN_POINT('Ctrl Pts',(-0.729446825476861,-0.151679013971647,
-2.41063988368698));
#57493=CARTESIAN_POINT('Ctrl Pts',(-0.568432793676261,-0.481646502687485,
-2.394790513392));
#57494=CARTESIAN_POINT('Ctrl Pts',(-0.269376677956068,-0.694647680375479,
-2.37894114309702));
#57495=CARTESIAN_POINT('Ctrl Pts',(0.0950967015076525,-0.738955893027485,
-2.36309177280204));
#57496=CARTESIAN_POINT('Ctrl Pts',(0.436476151493632,-0.603811033068285,
-2.34724240250705));
#57497=CARTESIAN_POINT('Ctrl Pts',(0.671858765611449,-0.322032597028224,
-2.33139303221208));
#57498=CARTESIAN_POINT('Ctrl Pts',(0.744082629677508,0.037950424106782,
-2.3155436619171));
#57499=CARTESIAN_POINT('Ctrl Pts',(0.635608409551846,0.388717306258229,
-2.29969429162212));
#57500=CARTESIAN_POINT('Ctrl Pts',(0.372778722276054,0.645085435191274,
-2.28384492132714));
#57501=CARTESIAN_POINT('Ctrl Pts',(0.0194209158693028,0.744796631641469,
-2.26799555103216));
#57502=CARTESIAN_POINT('Ctrl Pts',(-0.338653197773854,0.663636350809105,
-2.25214618073718));
#57503=CARTESIAN_POINT('Ctrl Pts',(-0.614486466647313,0.421314107032963,
-2.23629681044219));
#57504=CARTESIAN_POINT('Ctrl Pts',(-0.741093664576154,0.0766770813396573,
-2.22044744014722));
#57505=CARTESIAN_POINT('Ctrl Pts',(-0.687728638917978,-0.286580728050069,
-2.20459806985223));
#57506=CARTESIAN_POINT('Ctrl Pts',(-0.467350915288179,-0.580243325215363,
-2.18874869955726));
#57507=CARTESIAN_POINT('Ctrl Pts',(-0.133478518258434,-0.732995688692106,
-2.17289932926227));
#57508=CARTESIAN_POINT('Ctrl Pts',(0.232808709554962,-0.707742396096938,
-2.1570499589673));
#57509=CARTESIAN_POINT('Ctrl Pts',(0.542559087666651,-0.510616128679865,
-2.14120058867231));
#57510=CARTESIAN_POINT('Ctrl Pts',(0.720550728519998,-0.189488369318495,
-2.12535121837734));
#57511=CARTESIAN_POINT('Ctrl Pts',(0.723558932032592,0.177656033822487,
-2.10950184808235));
#57512=CARTESIAN_POINT('Ctrl Pts',(0.550853165613154,0.501657237973947,
-2.09365247778737));
#57513=CARTESIAN_POINT('Ctrl Pts',(0.244374471662288,0.703832588104202,
-2.07780310749239));
#57514=CARTESIAN_POINT('Ctrl Pts',(-0.121449780286455,0.735084447765053,
-2.06195373719741));
#57515=CARTESIAN_POINT('Ctrl Pts',(-0.457780341954077,0.587823402900981,
-2.04610436690243));
#57516=CARTESIAN_POINT('Ctrl Pts',(-0.682940413312603,0.297811326752515,
-2.03025499660745));
#57517=CARTESIAN_POINT('Ctrl Pts',(-0.74225059195669,-0.0645232765568143,
-2.01440562631247));
#57518=CARTESIAN_POINT('Ctrl Pts',(-0.621307590903676,-0.41118860874683,
-1.99855625601749));
#57519=CARTESIAN_POINT('Ctrl Pts',(-0.349482030720463,-0.657998103858348,
-1.98270688572251));
#57520=CARTESIAN_POINT('Ctrl Pts',(0.00721412164145659,-0.745014866245382,
-1.96685751542753));
#57521=CARTESIAN_POINT('Ctrl Pts',(0.362158347661135,-0.651107153775044,
-1.95100814513255));
#57522=CARTESIAN_POINT('Ctrl Pts',(0.629153578520462,-0.399080153744305,
-1.93515877483757));
#57523=CARTESIAN_POINT('Ctrl Pts',(0.743360877278368,-0.0501378161632328,
-1.91930940454259));
#57524=CARTESIAN_POINT('Ctrl Pts',(0.67704536710375,0.310980329540358,-1.90346003424761));
#57525=CARTESIAN_POINT('Ctrl Pts',(0.446311557311583,0.596577897920959,
-1.88761066395263));
#57526=CARTESIAN_POINT('Ctrl Pts',(0.107192414839656,0.737298433931963,
-1.87176129365765));
#57527=CARTESIAN_POINT('Ctrl Pts',(-0.257958062364287,0.69896840596621,
-1.85591192336267));
#57528=CARTESIAN_POINT('Ctrl Pts',(-0.560464250060707,0.490896138588981,
-1.84006255306769));
#57529=CARTESIAN_POINT('Ctrl Pts',(-0.726863489140655,0.163611315720987,
-1.8242131827727));
#57530=CARTESIAN_POINT('Ctrl Pts',(-0.716746257175511,-0.203405991314366,
-1.80836381247773));
#57531=CARTESIAN_POINT('Ctrl Pts',(-0.532569491554352,-0.521026804630263,
-1.79251444218274));
#57532=CARTESIAN_POINT('Ctrl Pts',(-0.219059930105742,-0.712117926680512,
-1.77666507188777));
#57533=CARTESIAN_POINT('Ctrl Pts',(0.147647633976574,-0.730273490316333,
-1.76081570159278));
#57534=CARTESIAN_POINT('Ctrl Pts',(0.478499442890174,-0.571084475039791,
-1.7449663312978));
#57535=CARTESIAN_POINT('Ctrl Pts',(0.693149194171365,-0.27320942351476,
-1.72911696100282));
#57536=CARTESIAN_POINT('Ctrl Pts',(0.739469882993344,0.0910136617409349,
-1.71326759070784));
#57537=CARTESIAN_POINT('Ctrl Pts',(0.606212678386616,0.433134370653044,
-1.69741822041286));
#57538=CARTESIAN_POINT('Ctrl Pts',(0.325738665823124,0.670069784474314,
-1.68156885011788));
#57539=CARTESIAN_POINT('Ctrl Pts',(-0.0338399387759541,0.744280896584965,
-1.6657194798229));
#57540=CARTESIAN_POINT('Ctrl Pts',(-0.385200622592994,0.637745776020236,
-1.64987010952792));
#57541=CARTESIAN_POINT('Ctrl Pts',(-0.64301656855991,0.376336135702008,
-1.63402073923294));
#57542=CARTESIAN_POINT('Ctrl Pts',(-0.744677999681247,0.0235344697925616,
-1.61817136893796));
#57543=CARTESIAN_POINT('Ctrl Pts',(-0.665496762911727,-0.334982466752658,
-1.60232199864298));
#57544=CARTESIAN_POINT('Ctrl Pts',(-0.424701768076029,-0.612149983803623,
-1.586472628348));
#57545=CARTESIAN_POINT('Ctrl Pts',(-0.0807693086855734,-0.740658837287543,
-1.57062325805302));
#57546=CARTESIAN_POINT('Ctrl Pts',(0.282777718709647,-0.689301063599245,
-1.55477388775804));
#57547=CARTESIAN_POINT('Ctrl Pts',(0.577653082522177,-0.470548733640108,
-1.53892451746306));
#57548=CARTESIAN_POINT('Ctrl Pts',(0.732247244790675,-0.137525150333124,
-1.52307514716808));
#57549=CARTESIAN_POINT('Ctrl Pts',(0.709017508192331,0.228895975400221,
-1.5072257768731));
#57550=CARTESIAN_POINT('Ctrl Pts',(0.513605139882413,0.539730446393427,
-1.49137640657812));
#57551=CARTESIAN_POINT('Ctrl Pts',(0.193465407827965,0.719493106604671,
-1.47552703628314));
#57552=CARTESIAN_POINT('Ctrl Pts',(-0.173656779074324,0.72452916957098,
-1.45967766598816));
#57553=CARTESIAN_POINT('Ctrl Pts',(-0.498606973197754,0.553615643525593,
-1.44382829569318));
#57554=CARTESIAN_POINT('Ctrl Pts',(-0.702472060334454,0.24825833103272,
-1.4279789253982));
#57555=CARTESIAN_POINT('Ctrl Pts',(-0.735744056814447,-0.117387722270682,
-1.41212955510321));
#57556=CARTESIAN_POINT('Ctrl Pts',(-0.59034296482383,-0.454526543076082,
-1.39628018480824));
#57557=CARTESIAN_POINT('Ctrl Pts',(-0.301578974003058,-0.681285048211793,
-1.38043081451325));
#57558=CARTESIAN_POINT('Ctrl Pts',(0.0604225050500024,-0.742595660747599,
-1.36458144421827));
#57559=CARTESIAN_POINT('Ctrl Pts',(0.407750572214209,-0.62356929473529,
-1.3487320739233));
#57560=CARTESIAN_POINT('Ctrl Pts',(0.656057718463867,-0.353111122058863,
-1.33288270362831));
#57561=CARTESIAN_POINT('Ctrl Pts',(0.7450433483693,0.00309895600807202,
-1.31703333333333));
#57562=CARTESIAN_POINT('Ctrl Pts',(0.653097586624771,0.358556462530776,
-1.30118396303835));
#57563=CARTESIAN_POINT('Ctrl Pts',(0.402549167075302,0.626939680164418,
-1.28533459274337));
#57564=CARTESIAN_POINT('Ctrl Pts',(0.0542429711952568,0.743072603823875,
-1.26948522244839));
#57565=CARTESIAN_POINT('Ctrl Pts',(-0.307235956562828,0.678752724836228,
-1.25363585215341));
#57566=CARTESIAN_POINT('Ctrl Pts',(-0.594103615986673,0.44959991987237,
-1.23778648185843));
#57567=CARTESIAN_POINT('Ctrl Pts',(-0.736695114486434,0.111263213909636,
-1.22193711156345));
#57568=CARTESIAN_POINT('Ctrl Pts',(-0.70038256320506,-0.254093407305248,
-1.20608774126847));
#57569=CARTESIAN_POINT('Ctrl Pts',(-0.49398434895465,-0.557744258119735,
-1.19023837097349));
#57570=CARTESIAN_POINT('Ctrl Pts',(-0.167623617214091,-0.72594870165167,
-1.17438900067851));
#57571=CARTESIAN_POINT('Ctrl Pts',(0.199443973264722,-0.717858827351214,
-1.15853963038353));
#57572=CARTESIAN_POINT('Ctrl Pts',(0.518077233421729,-0.535439235289842,
-1.14269026008855));
#57573=CARTESIAN_POINT('Ctrl Pts',(0.710897096237059,-0.222989939323281,
-1.12684088979357));
#57574=CARTESIAN_POINT('Ctrl Pts',(0.731077875402266,0.143611749432251,
-1.11099151949859));
#57575=CARTESIAN_POINT('Ctrl Pts',(0.573718733312487,0.475337784658443,
-1.09514214920361));
#57576=CARTESIAN_POINT('Ctrl Pts',(0.277033833787142,0.691629560830709,
-1.07929277890863));
#57577=CARTESIAN_POINT('Ctrl Pts',(-0.086927845258402,0.739961312634932,
-1.06344340861365));
#57578=CARTESIAN_POINT('Ctrl Pts',(-0.429779375411057,0.60859582889547,
-1.04759403831867));
#57579=CARTESIAN_POINT('Ctrl Pts',(-0.668260360325273,0.329434796728608,
-1.03174466802369));
#57580=CARTESIAN_POINT('Ctrl Pts',(-0.744456456389999,-0.0297284210298624,
-1.01589529772871));
#57581=CARTESIAN_POINT('Ctrl Pts',(-0.639863685642797,-0.381672186926551,
-1.00004592743373));
#57582=CARTESIAN_POINT('Ctrl Pts',(-0.379882067571449,-0.640928084277264,
-0.984196557138746));
#57583=CARTESIAN_POINT('Ctrl Pts',(-0.0276473057078523,-0.744536648503469,
-0.968347186843765));
#57584=CARTESIAN_POINT('Ctrl Pts',(0.331301515824945,-0.667336871519755,
-0.952497816548785));
#57585=CARTESIAN_POINT('Ctrl Pts',(0.60979482501051,-0.428076471986122,
-0.936648446253804));
#57586=CARTESIAN_POINT('Ctrl Pts',(0.740201413401119,-0.0848590718583864,
-0.920799075958824));
#57587=CARTESIAN_POINT('Ctrl Pts',(0.690852458545734,0.278966082165907,
-0.904949705663843));
#57588=CARTESIAN_POINT('Ctrl Pts',(0.473732196124063,0.575045216337946,
-0.889100335368864));
#57589=CARTESIAN_POINT('Ctrl Pts',(0.141567586683216,0.731476460918855,
-0.873250965073882));
#57590=CARTESIAN_POINT('Ctrl Pts',(-0.224976257908425,0.710270989028275,
-0.857401594778903));
#57591=CARTESIAN_POINT('Ctrl Pts',(-0.53688533860254,0.516578481618539,
-0.841552224483921));
#57592=CARTESIAN_POINT('Ctrl Pts',(-0.718413533832164,0.197436543943786,
-0.825702854188942));
#57593=CARTESIAN_POINT('Ctrl Pts',(-0.72547730260804,-0.169652226269635,
-0.809853483893961));
#57594=CARTESIAN_POINT('Ctrl Pts',(-0.556361231299935,-0.495541496530917,
-0.79400411359898));
#57595=CARTESIAN_POINT('Ctrl Pts',(-0.252134616344252,-0.701090100998879,
-0.778154743304001));
#57596=CARTESIAN_POINT('Ctrl Pts',(0.113322082898667,-0.736381219209989,
-0.762305373009019));
#57597=CARTESIAN_POINT('Ctrl Pts',(0.451258877147593,-0.592844516102809,
-0.74645600271404));
#57598=CARTESIAN_POINT('Ctrl Pts',(0.679608897935057,-0.305337420446921,
-0.730606632419059));
#57599=CARTESIAN_POINT('Ctrl Pts',(0.742918073850576,0.0563198901262535,
-0.714757262124078));
#57600=CARTESIAN_POINT('Ctrl Pts',(0.625811974228227,0.404300095708931,
-0.698907891829099));
#57601=CARTESIAN_POINT('Ctrl Pts',(0.356729440407579,0.654097317548526,
-0.683058521534117));
#57602=CARTESIAN_POINT('Ctrl Pts',(0.00101630417067649,0.745049100129323,
-0.667209151239138));
#57603=CARTESIAN_POINT('Ctrl Pts',(-0.354943638280041,0.655068094263647,
-0.651359780944157));
#57604=CARTESIAN_POINT('Ctrl Pts',(-0.624706654643346,0.406005899122171,
-0.635510410649177));
#57605=CARTESIAN_POINT('Ctrl Pts',(-0.742761660130492,0.0583464713403934,
-0.619661040354196));
#57606=CARTESIAN_POINT('Ctrl Pts',(-0.680439374650891,-0.303482210190962,
-0.603811670059217));
#57607=CARTESIAN_POINT('Ctrl Pts',(-0.452874565687931,-0.591611208675634,
-0.587962299764235));
#57608=CARTESIAN_POINT('Ctrl Pts',(-0.115330618474684,-0.736069319371431,
-0.572112929469256));
#57609=CARTESIAN_POINT('Ctrl Pts',(0.250221000166279,-0.701775352626115,
-0.556263559174274));
#57610=CARTESIAN_POINT('Ctrl Pts',(0.555007250081607,-0.497057488460266,
-0.540414188879294));
#57611=CARTESIAN_POINT('Ctrl Pts',(0.7250117663533,-0.171630804715129,-0.524564818584314));
#57612=CARTESIAN_POINT('Ctrl Pts',(0.718949496529346,0.195475870422815,
-0.508715448289334));
#57613=CARTESIAN_POINT('Ctrl Pts',(0.538292643427788,0.515111856308425,
-0.492866077994354));
#57614=CARTESIAN_POINT('Ctrl Pts',(0.226913145388744,0.709654577190661,
-0.477016707699373));
#57615=CARTESIAN_POINT('Ctrl Pts',(-0.139571483466669,0.731859956192972,
-0.461167337404393));
#57616=CARTESIAN_POINT('Ctrl Pts',(-0.472161624454404,0.576335488128052,
-0.445317967109412));
#57617=CARTESIAN_POINT('Ctrl Pts',(-0.690088826708267,0.280849792091782,
-0.429468596814432));
#57618=CARTESIAN_POINT('Ctrl Pts',(-0.740430166973819,-0.0828393767067807,
-0.413619226519452));
#57619=CARTESIAN_POINT('Ctrl Pts',(-0.61096041185947,-0.426411268137316,
-0.397769856224471));
#57620=CARTESIAN_POINT('Ctrl Pts',(-0.333120877035743,-0.666430548342542,
-0.381920485929491));
#57621=CARTESIAN_POINT('Ctrl Pts',(0.0256159964145952,-0.744609303785652,
-0.36607111563451));
#57622=CARTESIAN_POINT('Ctrl Pts',(0.378132106694367,-0.641962073708442,
-0.35022174533953));
#57623=CARTESIAN_POINT('Ctrl Pts',(0.638820046477084,-0.383416409890756,
-0.334372375044549));
#57624=CARTESIAN_POINT('Ctrl Pts',(0.744372581604882,-0.0317592977686295,
-0.318523004749569));
#57625=CARTESIAN_POINT('Ctrl Pts',(0.66915662209072,0.327610456569737,-0.302673634454589));
#57626=CARTESIAN_POINT('Ctrl Pts',(0.431438112678508,0.607421063535145,
-0.286824264159608));
#57627=CARTESIAN_POINT('Ctrl Pts',(0.0889462522057513,0.739721404103688,
-0.270974893864627));
#57628=CARTESIAN_POINT('Ctrl Pts',(-0.275145946691687,0.692382781846757,
-0.255125523569648));
#57629=CARTESIAN_POINT('Ctrl Pts',(-0.572419782762165,0.476901195004193,
-0.239276153274667));
#57630=CARTESIAN_POINT('Ctrl Pts',(-0.730683406529149,0.145605724755764,
-0.223426782979687));
#57631=CARTESIAN_POINT('Ctrl Pts',(-0.711502710426857,-0.221049717342616,
-0.207577412684706));
#57632=CARTESIAN_POINT('Ctrl Pts',(-0.519536239252636,-0.534023771456305,
-0.191728042389726));
#57633=CARTESIAN_POINT('Ctrl Pts',(-0.201401311784543,-0.717312199056277,
-0.175878672094745));
#57634=CARTESIAN_POINT('Ctrl Pts',(0.165641822669815,-0.726402996959048,
-0.160029301799765));
#57635=CARTESIAN_POINT('Ctrl Pts',(0.492462222867754,-0.559090442823836,
-0.144179931504785));
#57636=CARTESIAN_POINT('Ctrl Pts',(0.699684165074883,-0.256002039101042,
-0.128330561209804));
#57637=CARTESIAN_POINT('Ctrl Pts',(0.737000982771008,0.109250693550497,
-0.112481190914824));
#57638=CARTESIAN_POINT('Ctrl Pts',(0.595318037638767,0.447981949310424,
-0.0966318206198438));
#57639=CARTESIAN_POINT('Ctrl Pts',(0.309106256262539,0.67790301016905,-0.0807824503248628));
#57640=CARTESIAN_POINT('Ctrl Pts',(-0.0522567177097866,0.743237421289278,
-0.0649330800298829));
#57641=CARTESIAN_POINT('Ctrl Pts',(-0.284570593536469,0.666395263721345,
-0.0543668331665628));
#57642=CARTESIAN_POINT('Ctrl Pts',(-0.384580808941244,0.60256476484984,
-0.0490837097349025));
#57643=CARTESIAN_POINT('Ctrl Pts',(-0.325579286442189,0.678938089483059,
-3.8309162902651));
#57644=CARTESIAN_POINT('Ctrl Pts',(-0.438265504649167,0.624900322146083,
-3.82563316683344));
#57645=CARTESIAN_POINT('Ctrl Pts',(-0.63610095367448,0.459691134517002,
-3.81506691997012));
#57646=CARTESIAN_POINT('Ctrl Pts',(-0.778397349342817,0.100004018584218,
-3.79921754967514));
#57647=CARTESIAN_POINT('Ctrl Pts',(-0.731650542618167,-0.283869852061292,
-3.78336817938015));
#57648=CARTESIAN_POINT('Ctrl Pts',(-0.507231019672293,-0.598855316207359,
-3.76751880908518));
#57649=CARTESIAN_POINT('Ctrl Pts',(-0.159628843925671,-0.76838611128163,
-3.75166943879019));
#57650=CARTESIAN_POINT('Ctrl Pts',(0.22673703716271,-0.751329333310609,
-3.73582006849522));
#57651=CARTESIAN_POINT('Ctrl Pts',(0.558041396815425,-0.551808232021081,
-3.71997069820023));
#57652=CARTESIAN_POINT('Ctrl Pts',(0.753826759884924,-0.218285537365442,
-3.70412132790526));
#57653=CARTESIAN_POINT('Ctrl Pts',(0.766547927636159,0.168248770824598,
-3.68827195761027));
#57654=CARTESIAN_POINT('Ctrl Pts',(0.59311527330172,0.513923550886757,-3.67242258731529));
#57655=CARTESIAN_POINT('Ctrl Pts',(0.275646531216097,0.734794077718187,
-3.65657321702032));
#57656=CARTESIAN_POINT('Ctrl Pts',(-0.108762117677957,0.777221992964339,
-3.64072384672533));
#57657=CARTESIAN_POINT('Ctrl Pts',(-0.466758219578375,0.630904149396545,
-3.62487447643035));
#57658=CARTESIAN_POINT('Ctrl Pts',(-0.711403589971996,0.331373195147995,
-3.60902510613537));
#57659=CARTESIAN_POINT('Ctrl Pts',(-0.783286872432518,-0.0486306488929434,
-3.59317573584039));
#57660=CARTESIAN_POINT('Ctrl Pts',(-0.664951447866154,-0.416824710701167,
-3.57732636554541));
#57661=CARTESIAN_POINT('Ctrl Pts',(-0.385134692228658,-0.68379421838201,
-3.56147699525044));
#57662=CARTESIAN_POINT('Ctrl Pts',(-0.0117892102387679,-0.78470649347194,
-3.54562762495545));
#57663=CARTESIAN_POINT('Ctrl Pts',(0.364419243976096,-0.695055307100327,
-3.52977825466047));
#57664=CARTESIAN_POINT('Ctrl Pts',(0.652129651463901,-0.436612165878492,
-3.51392888436549));
#57665=CARTESIAN_POINT('Ctrl Pts',(0.781472461170702,-0.0721391576041502,
-3.49807951407051));
#57666=CARTESIAN_POINT('Ctrl Pts',(0.721037185788124,0.30985261384819,-3.48223014377553));
#57667=CARTESIAN_POINT('Ctrl Pts',(0.485500338492858,0.616597670259985,
-3.46638077348055));
#57668=CARTESIAN_POINT('Ctrl Pts',(0.132061288474505,0.773603956619382,
-3.45053140318557));
#57669=CARTESIAN_POINT('Ctrl Pts',(-0.25344842260748,0.742742999097299,
-3.43468203289059));
#57670=CARTESIAN_POINT('Ctrl Pts',(-0.577408995760196,0.531509282362323,
-3.41883266259561));
#57671=CARTESIAN_POINT('Ctrl Pts',(-0.761147643056275,0.191200238216922,
-3.40298329230063));
#57672=CARTESIAN_POINT('Ctrl Pts',(-0.760044022301481,-0.195541171593737,
-3.38713392200565));
#57673=CARTESIAN_POINT('Ctrl Pts',(-0.574366144261561,-0.534796033969841,
-3.37128455171067));
#57674=CARTESIAN_POINT('Ctrl Pts',(-0.249205287110151,-0.74417739182315,
-3.35543518141569));
#57675=CARTESIAN_POINT('Ctrl Pts',(0.136474276103288,-0.772837652800438,
-3.33958581112071));
#57676=CARTESIAN_POINT('Ctrl Pts',(0.489011498332319,-0.613816764289597,
-3.32373644082573));
#57677=CARTESIAN_POINT('Ctrl Pts',(0.722793843922638,-0.305732439907269,
-3.30788707053074));
#57678=CARTESIAN_POINT('Ctrl Pts',(0.781048018778739,0.0765980286034119,
-3.29203770023577));
#57679=CARTESIAN_POINT('Ctrl Pts',(0.649627183056744,0.4403269111216,-3.27618832994078));
#57680=CARTESIAN_POINT('Ctrl Pts',(0.360446465924673,0.697123813125427,
-3.2603389596458));
#57681=CARTESIAN_POINT('Ctrl Pts',(-0.0162675213692028,0.784626429183104,
-3.24448958935083));
#57682=CARTESIAN_POINT('Ctrl Pts',(-0.38903099318439,0.681585029153437,
-3.22864021905584));
#57683=CARTESIAN_POINT('Ctrl Pts',(-0.667319533915525,0.413022887112677,
-3.21279084876086));
#57684=CARTESIAN_POINT('Ctrl Pts',(-0.783551662478414,0.0441594593653245,
-3.19694147846588));
#57685=CARTESIAN_POINT('Ctrl Pts',(-0.709500778606978,-0.335427951697853,
-3.1810921081709));
#57686=CARTESIAN_POINT('Ctrl Pts',(-0.463149902351115,-0.633557758674201,
-3.16524273787593));
#57687=CARTESIAN_POINT('Ctrl Pts',(-0.104324555236145,-0.777830092500222,
-3.14939336758094));
#57688=CARTESIAN_POINT('Ctrl Pts',(0.27983567608852,-0.733208878841634,
-3.13354399728597));
#57689=CARTESIAN_POINT('Ctrl Pts',(0.596038709461116,-0.510530236565918,
-3.11769462699098));
#57690=CARTESIAN_POINT('Ctrl Pts',(0.767495650655195,-0.163870960970766,
-3.101845256696));
#57691=CARTESIAN_POINT('Ctrl Pts',(0.752568730477612,0.222583852809316,
-3.08599588640102));
#57692=CARTESIAN_POINT('Ctrl Pts',(0.554882903700043,0.554984890610126,
-3.07014651610604));
#57693=CARTESIAN_POINT('Ctrl Pts',(0.222445540399176,0.75260962469307,-3.05429714581105));
#57694=CARTESIAN_POINT('Ctrl Pts',(-0.164012010155015,0.767465521146739,
-3.03844777551608));
#57695=CARTESIAN_POINT('Ctrl Pts',(-0.510639769181497,0.595944873083403,
-3.02259840522109));
#57696=CARTESIAN_POINT('Ctrl Pts',(-0.733260295243549,0.279700920705432,
-3.00674903492612));
#57697=CARTESIAN_POINT('Ctrl Pts',(-0.777810906379899,-0.104467504711289,
-2.99089966463113));
#57698=CARTESIAN_POINT('Ctrl Pts',(-0.633472629319529,-0.463266331095978,
-2.97505029433616));
#57699=CARTESIAN_POINT('Ctrl Pts',(-0.335297552500043,-0.709562412273652,
-2.95920092404117));
#57700=CARTESIAN_POINT('Ctrl Pts',(0.0443034613785977,-0.78354353352829,
-2.9433515537462));
#57701=CARTESIAN_POINT('Ctrl Pts',(0.413145521513561,-0.667243616438114,
-2.92750218345121));
#57702=CARTESIAN_POINT('Ctrl Pts',(0.681656514570333,-0.388905723496004,
-2.91165281315624));
#57703=CARTESIAN_POINT('Ctrl Pts',(0.7846294056114,-0.0161233208125725,
-2.89580344286125));
#57704=CARTESIAN_POINT('Ctrl Pts',(0.697057557749046,0.36057457870607,-2.87995407256628));
#57705=CARTESIAN_POINT('Ctrl Pts',(0.440207513846546,0.649708096284145,
-2.86410470227129));
#57706=CARTESIAN_POINT('Ctrl Pts',(0.0764544846756664,0.781062082933939,
-2.84825533197632));
#57707=CARTESIAN_POINT('Ctrl Pts',(-0.305865271304502,0.722737643570575,
-2.83240596168133));
#57708=CARTESIAN_POINT('Ctrl Pts',(-0.613906625476715,0.488898681548557,
-2.81655659138636));
#57709=CARTESIAN_POINT('Ctrl Pts',(-0.772862721276039,0.136332240082525,
-2.80070722109137));
#57710=CARTESIAN_POINT('Ctrl Pts',(-0.744131579787873,-0.249342049375011,
-2.78485785079639));
#57711=CARTESIAN_POINT('Ctrl Pts',(-0.534690466730406,-0.574464420492465,
-2.76900848050141));
#57712=CARTESIAN_POINT('Ctrl Pts',(-0.195401485814985,-0.760079946430257,
-2.75315911020643));
#57713=CARTESIAN_POINT('Ctrl Pts',(0.191340120288431,-0.761112491023588,
-2.73730973991145));
#57714=CARTESIAN_POINT('Ctrl Pts',(0.531615390818176,-0.577311304124008,
-2.72146036961647));
#57715=CARTESIAN_POINT('Ctrl Pts',(0.742789565829382,-0.253311915470078,
-2.70561099932149));
#57716=CARTESIAN_POINT('Ctrl Pts',(0.773579673064216,0.132203460794283,
-2.68976162902651));
#57717=CARTESIAN_POINT('Ctrl Pts',(0.616508433565354,0.485613649897649,
-2.67391225873153));
#57718=CARTESIAN_POINT('Ctrl Pts',(0.309720094929824,0.721094118975316,
-2.65806288843655));
#57719=CARTESIAN_POINT('Ctrl Pts',(-0.0722827770885867,0.781459190079997,
-2.64221351814157));
#57720=CARTESIAN_POINT('Ctrl Pts',(-0.436732008128137,0.652049398972571,
-2.62636414784659));
#57721=CARTESIAN_POINT('Ctrl Pts',(-0.695122269335044,0.364291499075428,
-2.61051477755161));
#57722=CARTESIAN_POINT('Ctrl Pts',(-0.784704313096684,-0.0119334249730362,
-2.59466540725663));
#57723=CARTESIAN_POINT('Ctrl Pts',(-0.683723426911941,-0.385260354975586,
-2.57881603696165));
#57724=CARTESIAN_POINT('Ctrl Pts',(-0.41670249566724,-0.665028041310152,
-2.56296666666666));
#57725=CARTESIAN_POINT('Ctrl Pts',(-0.0484866975599475,-0.783295797118723,
-2.54711729637169));
#57726=CARTESIAN_POINT('Ctrl Pts',(0.331503939803658,-0.711342676576329,
-2.53126792607671));
#57727=CARTESIAN_POINT('Ctrl Pts',(0.630989906804924,-0.466642264625097,
-2.51541855578172));
#57728=CARTESIAN_POINT('Ctrl Pts',(0.777241995260494,-0.108619272818464,
-2.49956918548675));
#57729=CARTESIAN_POINT('Ctrl Pts',(0.734743353763132,0.275781561611777,
-2.48371981519176));
#57730=CARTESIAN_POINT('Ctrl Pts',(0.513814641327085,0.593209726810042,
-2.46787044489679));
#57731=CARTESIAN_POINT('Ctrl Pts',(0.168107688391456,0.766578809208684,
-2.4520210746018));
#57732=CARTESIAN_POINT('Ctrl Pts',(-0.218423678417938,0.753786682245382,
-2.43617170430682));
#57733=CARTESIAN_POINT('Ctrl Pts',(-0.551911554278842,0.557939872994966,
-2.42032233401184));
#57734=CARTESIAN_POINT('Ctrl Pts',(-0.751369476309632,0.226599152015872,
-2.40447296371687));
#57735=CARTESIAN_POINT('Ctrl Pts',(-0.768359726775325,-0.159770447498504,
-2.38862359342188));
#57736=CARTESIAN_POINT('Ctrl Pts',(-0.598756277750203,-0.507340305395548,
-2.3727742231269));
#57737=CARTESIAN_POINT('Ctrl Pts',(-0.28374678378875,-0.73170419454426,
-2.35692485283192));
#57738=CARTESIAN_POINT('Ctrl Pts',(0.100169708107077,-0.778376062839723,
-2.34107548253694));
#57739=CARTESIAN_POINT('Ctrl Pts',(0.459760307115391,-0.636021796501728,
-2.32522611224196));
#57740=CARTESIAN_POINT('Ctrl Pts',(0.707699587614688,-0.339211673316421,
-2.30937674194698));
#57741=CARTESIAN_POINT('Ctrl Pts',(0.783776289194928,0.039974918635952,
-2.293527371652));
#57742=CARTESIAN_POINT('Ctrl Pts',(0.669515428461959,0.409453729590444,
-2.27767800135702));
#57743=CARTESIAN_POINT('Ctrl Pts',(0.39266488960102,0.679498013314787,-2.26182863106204));
#57744=CARTESIAN_POINT('Ctrl Pts',(0.0204569395463645,0.784528380142186,
-2.24597926076706));
#57745=CARTESIAN_POINT('Ctrl Pts',(-0.356718912777502,0.699038541777891,
-2.23012989047208));
#57746=CARTESIAN_POINT('Ctrl Pts',(-0.647266719286364,0.443789431744821,
-2.2142805201771));
#57747=CARTESIAN_POINT('Ctrl Pts',(-0.780627875453987,0.0807674791504598,
-2.19843114988212));
#57748=CARTESIAN_POINT('Ctrl Pts',(-0.724416051504697,-0.301868597151919,
-2.18258177958714));
#57749=CARTESIAN_POINT('Ctrl Pts',(-0.492282108903929,-0.611196851167628,
-2.16673240929215));
#57750=CARTESIAN_POINT('Ctrl Pts',(-0.140599032359052,-0.772097906825179,
-2.15088303899718));
#57751=CARTESIAN_POINT('Ctrl Pts',(0.245228069020143,-0.745497457935825,
-2.13503366870219));
#57752=CARTESIAN_POINT('Ctrl Pts',(0.571502319016177,-0.537855338342251,
-2.11918429840722));
#57753=CARTESIAN_POINT('Ctrl Pts',(0.758989060691919,-0.199596771953163,
-2.10333492811223));
#57754=CARTESIAN_POINT('Ctrl Pts',(0.762157739131931,0.187133231429987,
-2.08748555781726));
#57755=CARTESIAN_POINT('Ctrl Pts',(0.580238850922621,0.528418528729,-2.07163618752227));
#57756=CARTESIAN_POINT('Ctrl Pts',(0.257410815592424,0.741379078232026,
-2.0557868172273));
#57757=CARTESIAN_POINT('Ctrl Pts',(-0.127928612118938,0.774298092355551,
-2.03993744693231));
#57758=CARTESIAN_POINT('Ctrl Pts',(-0.482200985982773,0.619181293920742,
-2.02408807663734));
#57759=CARTESIAN_POINT('Ctrl Pts',(-0.719372394325873,0.31369830077,-2.00823870634235));
#57760=CARTESIAN_POINT('Ctrl Pts',(-0.781846520014441,-0.0679653203143754,
-1.99238933604737));
#57761=CARTESIAN_POINT('Ctrl Pts',(-0.654451721656478,-0.433123780973749,
-1.97653996575239));
#57762=CARTESIAN_POINT('Ctrl Pts',(-0.368125418136845,-0.693099518211992,
-1.96069059545741));
#57763=CARTESIAN_POINT('Ctrl Pts',(0.00759896450262343,-0.784758256638701,
-1.94484122516243));
#57764=CARTESIAN_POINT('Ctrl Pts',(0.381477962943217,-0.685840965102565,
-1.92899185486745));
#57765=CARTESIAN_POINT('Ctrl Pts',(0.662716259510312,-0.42036939113687,
-1.91314248457247));
#57766=CARTESIAN_POINT('Ctrl Pts',(0.783016034359574,-0.0528124564845589,
-1.89729311427749));
#57767=CARTESIAN_POINT('Ctrl Pts',(0.713162872348176,0.327569814128564,
-1.88144374398251));
#57768=CARTESIAN_POINT('Ctrl Pts',(0.470120390212704,0.628402804203147,
-1.86559437368753));
#57769=CARTESIAN_POINT('Ctrl Pts',(0.112910676559248,0.776630185315416,
-1.84974500339255));
#57770=CARTESIAN_POINT('Ctrl Pts',(-0.271719033375929,0.736255412561006,
-1.83389563309757));
#57771=CARTESIAN_POINT('Ctrl Pts',(-0.590362646053683,0.517083370230197,
-1.81804626280259));
#57772=CARTESIAN_POINT('Ctrl Pts',(-0.765638580377628,0.172339287051596,
-1.8021968925076));
#57773=CARTESIAN_POINT('Ctrl Pts',(-0.754981636900799,-0.214256840186529,
-1.78634752221263));
#57774=CARTESIAN_POINT('Ctrl Pts',(-0.560979820224823,-0.548821379799159,
-1.77049815191765));
#57775=CARTESIAN_POINT('Ctrl Pts',(-0.23074585036879,-0.750106404559852,
-1.75464878162267));
#57776=CARTESIAN_POINT('Ctrl Pts',(0.155524010440509,-0.76923049068574,
-1.73879941132768));
#57777=CARTESIAN_POINT('Ctrl Pts',(0.504025363275639,-0.601549415093211,
-1.72295004103271));
#57778=CARTESIAN_POINT('Ctrl Pts',(0.730125770442385,-0.287783990103754,
-1.70710067073772));
#57779=CARTESIAN_POINT('Ctrl Pts',(0.77891747199518,0.0958688554472317,
-1.69125130044275));
#57780=CARTESIAN_POINT('Ctrl Pts',(0.638551559434616,0.456240256408558,
-1.67540193014776));
#57781=CARTESIAN_POINT('Ctrl Pts',(0.34311544519835,0.705815171904418,-1.65955255985279));
#57782=CARTESIAN_POINT('Ctrl Pts',(-0.0356451563072939,0.783985132802881,
-1.6437031895578));
#57783=CARTESIAN_POINT('Ctrl Pts',(-0.405749445733414,0.671766814386624,
-1.62785381926282));
#57784=CARTESIAN_POINT('Ctrl Pts',(-0.677318781403579,0.396412075979144,
-1.61200444896784));
#57785=CARTESIAN_POINT('Ctrl Pts',(-0.784403419668906,0.0247899341638738,
-1.59615507867286));
#57786=CARTESIAN_POINT('Ctrl Pts',(-0.700998198993379,-0.352852363789961,
-1.58030570837788));
#57787=CARTESIAN_POINT('Ctrl Pts',(-0.447357810168782,-0.644805594970389,
-1.5644563380829));
#57788=CARTESIAN_POINT('Ctrl Pts',(-0.0850780095079747,-0.780169851969611,
-1.54860696778792));
#57789=CARTESIAN_POINT('Ctrl Pts',(0.297862713356593,-0.726072358388593,
-1.53275759749294));
#57790=CARTESIAN_POINT('Ctrl Pts',(0.608468429988034,-0.495650517332548,
-1.51690822719796));
#57791=CARTESIAN_POINT('Ctrl Pts',(0.771309536608839,-0.144861535130568,
-1.50105885690298));
#57792=CARTESIAN_POINT('Ctrl Pts',(0.746840591865543,0.24110660705598,-1.485209486608));
#57793=CARTESIAN_POINT('Ctrl Pts',(0.541003800643689,0.568522781701145,
-1.46936011631302));
#57794=CARTESIAN_POINT('Ctrl Pts',(0.203785968637258,0.757875019123007,
-1.45351074601804));
#57795=CARTESIAN_POINT('Ctrl Pts',(-0.182920633364878,0.763179734737182,
-1.43766137572306));
#57796=CARTESIAN_POINT('Ctrl Pts',(-0.525205545234974,0.583148695341557,
-1.42181200542808));
#57797=CARTESIAN_POINT('Ctrl Pts',(-0.739945972063181,0.261501862424725,
-1.4059626351331));
#57798=CARTESIAN_POINT('Ctrl Pts',(-0.774992888756427,-0.123649860497661,
-1.39011326483812));
#57799=CARTESIAN_POINT('Ctrl Pts',(-0.621835263810005,-0.478773610703918,
-1.37426389454314));
#57800=CARTESIAN_POINT('Ctrl Pts',(-0.317666936057598,-0.717628722502035,
-1.35841452424816));
#57801=CARTESIAN_POINT('Ctrl Pts',(0.0636457900011377,-0.782209996765098,
-1.34256515395318));
#57802=CARTESIAN_POINT('Ctrl Pts',(0.429502339741044,-0.656834077816532,
-1.3267157836582));
#57803=CARTESIAN_POINT('Ctrl Pts',(0.691055621467951,-0.371948106140721,
-1.31086641336322));
#57804=CARTESIAN_POINT('Ctrl Pts',(0.784788258163402,0.00326427219707354,
-1.29501704306824));
#57805=CARTESIAN_POINT('Ctrl Pts',(0.687937579121799,0.377683932483451,
-1.27916767277326));
#57806=CARTESIAN_POINT('Ctrl Pts',(0.424023461649061,0.660384259045651,
-1.26331830247827));
#57807=CARTESIAN_POINT('Ctrl Pts',(0.0571366041655278,0.782712382736185,
-1.2474689321833));
#57808=CARTESIAN_POINT('Ctrl Pts',(-0.323625694697954,0.714961310390562,
-1.23161956188831));
#57809=CARTESIAN_POINT('Ctrl Pts',(-0.625796529798224,0.473584173000561,
-1.21577019159333));
#57810=CARTESIAN_POINT('Ctrl Pts',(-0.775994681330568,0.117198635532986,
-1.19992082129835));
#57811=CARTESIAN_POINT('Ctrl Pts',(-0.73774500910418,-0.267648215323767,
-1.18407145100337));
#57812=CARTESIAN_POINT('Ctrl Pts',(-0.520336323550321,-0.587497554053001,
-1.16822208070839));
#57813=CARTESIAN_POINT('Ctrl Pts',(-0.176565627850278,-0.764674992847263,
-1.15237271041341));
#57814=CARTESIAN_POINT('Ctrl Pts',(0.210083465240229,-0.756153557987252,
-1.13652334011843));
#57815=CARTESIAN_POINT('Ctrl Pts',(0.545714461448512,-0.564002652644547,
-1.12067396982345));
#57816=CARTESIAN_POINT('Ctrl Pts',(0.748820447978499,-0.234885508947245,
-1.10482459952847));
#57817=CARTESIAN_POINT('Ctrl Pts',(0.770077786312045,0.151272828534624,
-1.08897522923349));
#57818=CARTESIAN_POINT('Ctrl Pts',(0.604324199897217,0.50069504395661,-1.07312585893851));
#57819=CARTESIAN_POINT('Ctrl Pts',(0.291812416480199,0.72852507109372,-1.05727648864353));
#57820=CARTESIAN_POINT('Ctrl Pts',(-0.091565077945533,0.779435117328539,
-1.04142711834855));
#57821=CARTESIAN_POINT('Ctrl Pts',(-0.452706286367931,0.641061840938205,
-1.02557774805357));
#57822=CARTESIAN_POINT('Ctrl Pts',(-0.703909222634067,0.34700874904652,
-1.00972837775859));
#57823=CARTESIAN_POINT('Ctrl Pts',(-0.784170057980586,-0.0313143064883875,
-0.993879007463609));
#57824=CARTESIAN_POINT('Ctrl Pts',(-0.673997705525074,-0.402032782955643,
-0.978029637168627));
#57825=CARTESIAN_POINT('Ctrl Pts',(-0.400147168308302,-0.675118885322409,
-0.962180266873648));
#57826=CARTESIAN_POINT('Ctrl Pts',(-0.0291221724707292,-0.784254528003958,
-0.946330896578668));
#57827=CARTESIAN_POINT('Ctrl Pts',(0.348975049707139,-0.702936469608757,
-0.930481526283687));
#57828=CARTESIAN_POINT('Ctrl Pts',(0.642324798422119,-0.450912540251555,
-0.914632155988707));
#57829=CARTESIAN_POINT('Ctrl Pts',(0.779688026454552,-0.0893859442391789,
-0.898782785693727));
#57830=CARTESIAN_POINT('Ctrl Pts',(0.727706513690353,0.293847742133158,
-0.882933415398745));
#57831=CARTESIAN_POINT('Ctrl Pts',(0.499003804068385,0.605721445178727,
-0.867084045103767));
#57832=CARTESIAN_POINT('Ctrl Pts',(0.149119618353334,0.770497634679226,
-0.851234674808784));
#57833=CARTESIAN_POINT('Ctrl Pts',(-0.236977789223283,0.748160940599662,
-0.835385304513805));
#57834=CARTESIAN_POINT('Ctrl Pts',(-0.565525899449417,0.54413575757898,
-0.819535934218824));
#57835=CARTESIAN_POINT('Ctrl Pts',(-0.756737855711574,0.20796894805998,
-0.803686563923844));
#57836=CARTESIAN_POINT('Ctrl Pts',(-0.764178446659503,-0.178702454614348,
-0.787837193628863));
#57837=CARTESIAN_POINT('Ctrl Pts',(-0.586040748605003,-0.521976538360308,
-0.771987823333882));
#57838=CARTESIAN_POINT('Ctrl Pts',(-0.265584931154134,-0.73849029104517,
-0.756138453038903));
#57839=CARTESIAN_POINT('Ctrl Pts',(0.119367336469941,-0.775664041069455,
-0.740289082743921));
#57840=CARTESIAN_POINT('Ctrl Pts',(0.475331628626109,-0.624470262263764,
-0.724439712448942));
#57841=CARTESIAN_POINT('Ctrl Pts',(0.715863156701094,-0.321625879714412,
-0.708590342153962));
#57842=CARTESIAN_POINT('Ctrl Pts',(0.782549609242745,0.0593243179324704,
-0.692740971858981));
#57843=CARTESIAN_POINT('Ctrl Pts',(0.659196394769945,0.425867794915784,
-0.676891601564001));
#57844=CARTESIAN_POINT('Ctrl Pts',(0.375759446461501,0.688990641459715,
-0.66104223126902));
#57845=CARTESIAN_POINT('Ctrl Pts',(0.0010705196974362,0.78479431675548,
-0.64519286097404));
#57846=CARTESIAN_POINT('Ctrl Pts',(-0.373878379347529,0.690013205004504,
-0.629343490679059));
#57847=CARTESIAN_POINT('Ctrl Pts',(-0.658032111062648,0.427664595722584,
-0.613494120384079));
#57848=CARTESIAN_POINT('Ctrl Pts',(-0.782384851512599,0.0614590086783985,
-0.597644750089098));
#57849=CARTESIAN_POINT('Ctrl Pts',(-0.716737935835347,-0.319671701842087,
-0.581795379794119));
#57850=CARTESIAN_POINT('Ctrl Pts',(-0.477033507312882,-0.623171163104398,
-0.565946009499137));
#57851=CARTESIAN_POINT('Ctrl Pts',(-0.121483018919316,-0.775335502694393,
-0.550096639204157));
#57852=CARTESIAN_POINT('Ctrl Pts',(0.263569231651014,-0.739212097946903,
-0.534247268909177));
#57853=CARTESIAN_POINT('Ctrl Pts',(0.58461453821839,-0.523573402043788,
-0.518397898614196));
#57854=CARTESIAN_POINT('Ctrl Pts',(0.763688076015605,-0.180786581847057,
-0.502548528319217));
#57855=CARTESIAN_POINT('Ctrl Pts',(0.757302409750591,0.205903680903747,
-0.486699158024236));
#57856=CARTESIAN_POINT('Ctrl Pts',(0.567008278031727,0.542590894014966,
-0.470849787729256));
#57857=CARTESIAN_POINT('Ctrl Pts',(0.239018001454253,0.747511645799011,
-0.455000417434275));
#57858=CARTESIAN_POINT('Ctrl Pts',(-0.147017031477197,0.770901587803361,
-0.439151047139295));
#57859=CARTESIAN_POINT('Ctrl Pts',(-0.497349449046418,0.607080547508727,
-0.423301676844315));
#57860=CARTESIAN_POINT('Ctrl Pts',(-0.726902145325857,0.295831940012187,
-0.407452306549334));
#57861=CARTESIAN_POINT('Ctrl Pts',(-0.779928983062327,-0.0872585068980811,
-0.391602936254354));
#57862=CARTESIAN_POINT('Ctrl Pts',(-0.643552564396997,-0.449158504824145,
-0.375753565959373));
#57863=CARTESIAN_POINT('Ctrl Pts',(-0.350891466139449,-0.701981797925372,
-0.359904195664393));
#57864=CARTESIAN_POINT('Ctrl Pts',(0.0269825014226717,-0.784331059137986,
-0.344054825369413));
#57865=CARTESIAN_POINT('Ctrl Pts',(0.398303854423826,-0.676208033714155,
-0.328205455074432));
#57866=CARTESIAN_POINT('Ctrl Pts',(0.672898392626291,-0.403870052833872,
-0.312356084779451));
#57867=CARTESIAN_POINT('Ctrl Pts',(0.784081708830621,-0.0334535219070024,
-0.296506714484472));
#57868=CARTESIAN_POINT('Ctrl Pts',(0.704853296171943,0.345087088060326,
-0.28065734418949));
#57869=CARTESIAN_POINT('Ctrl Pts',(0.454453510249238,0.639824406817222,
-0.26480797389451));
#57870=CARTESIAN_POINT('Ctrl Pts',(0.0936911583621272,0.779182410692385,
-0.24895860359953));
#57871=CARTESIAN_POINT('Ctrl Pts',(-0.289823818597269,0.729318473263532,
-0.23310923330455));
#57872=CARTESIAN_POINT('Ctrl Pts',(-0.602955955831871,0.502341855628342,
-0.217259863009569));
#57873=CARTESIAN_POINT('Ctrl Pts',(-0.769662274193841,0.15337317400364,
-0.201410492714589));
#57874=CARTESIAN_POINT('Ctrl Pts',(-0.749458369122514,-0.232841784334449,
-0.185561122419608));
#57875=CARTESIAN_POINT('Ctrl Pts',(-0.547251299066349,-0.562511679805382,
-0.169711752124628));
#57876=CARTESIAN_POINT('Ctrl Pts',(-0.212145219487114,-0.755577769385975,
-0.153862381829647));
#57877=CARTESIAN_POINT('Ctrl Pts',(0.174478112953526,-0.765153522886825,
-0.138013011534667));
#57878=CARTESIAN_POINT('Ctrl Pts',(0.518732998477949,-0.588915552014349,
-0.122163641239687));
#57879=CARTESIAN_POINT('Ctrl Pts',(0.737009354389205,-0.269658664549011,
-0.106314270944705));
#57880=CARTESIAN_POINT('Ctrl Pts',(0.776316866393766,0.115078755729171,
-0.090464900649726));
#57881=CARTESIAN_POINT('Ctrl Pts',(0.627075735706326,0.471879890555984,
-0.0746155303547465));
#57882=CARTESIAN_POINT('Ctrl Pts',(0.325595766972002,0.714066267041671,
-0.0587661600597641));
#57883=CARTESIAN_POINT('Ctrl Pts',(-0.0550443924619386,0.782885992515902,
-0.0429167897647847));
#57884=CARTESIAN_POINT('Ctrl Pts',(-0.299751230468417,0.701944631018955,
-0.0323505429014654));
#57885=CARTESIAN_POINT('Ctrl Pts',(-0.405096567646243,0.634709045147731,
-0.0270674194698051));
#57886=CARTESIAN_POINT('Ctrl Pts',(-0.342067962509734,0.713322310757514,
-3.8089));
#57887=CARTESIAN_POINT('Ctrl Pts',(-0.460461074940839,0.656547848310817,
-3.80361687656834));
#57888=CARTESIAN_POINT('Ctrl Pts',(-0.668315725953181,0.482971786953477,
-3.79305062970501));
#57889=CARTESIAN_POINT('Ctrl Pts',(-0.817818597191245,0.105068633983768,
-3.77720125941004));
#57890=CARTESIAN_POINT('Ctrl Pts',(-0.768704339632432,-0.298246190578182,
-3.76135188911506));
#57891=CARTESIAN_POINT('Ctrl Pts',(-0.532919287701208,-0.629183815996688,
-3.74550251882008));
#57892=CARTESIAN_POINT('Ctrl Pts',(-0.16771310606437,-0.807300348800163,
-3.7296531485251));
#57893=CARTESIAN_POINT('Ctrl Pts',(0.238219934613418,-0.789379745338913,
-3.71380377823012));
#57894=CARTESIAN_POINT('Ctrl Pts',(0.586302911621603,-0.579754073688803,
-3.69795440793514));
#57895=CARTESIAN_POINT('Ctrl Pts',(0.792003651881398,-0.229340416056228,
-3.68210503764016));
#57896=CARTESIAN_POINT('Ctrl Pts',(0.805369071963743,0.176769581565368,
-3.66625566734517));
#57897=CARTESIAN_POINT('Ctrl Pts',(0.623153073676116,0.53995075626169,-3.6504062970502));
#57898=CARTESIAN_POINT('Ctrl Pts',(0.289606406895025,0.772007076297564,
-3.63455692675521));
#57899=CARTESIAN_POINT('Ctrl Pts',(-0.11427027928863,0.816583715924684,
-3.61870755646024));
#57900=CARTESIAN_POINT('Ctrl Pts',(-0.490396778310394,0.662855734101919,
-3.60285818616526));
#57901=CARTESIAN_POINT('Ctrl Pts',(-0.747431997910723,0.348155298616472,
-3.58700881587027));
#57902=CARTESIAN_POINT('Ctrl Pts',(-0.82295574586927,-0.0510935052537138,
-3.5711594455753));
#57903=CARTESIAN_POINT('Ctrl Pts',(-0.698627328000686,-0.437934430876563,
-3.55531007528031));
#57904=CARTESIAN_POINT('Ctrl Pts',(-0.404639499343168,-0.71842437402542,
-3.53946070498534));
#57905=CARTESIAN_POINT('Ctrl Pts',(-0.0123862644028858,-0.824447262365292,
-3.52361133469035));
#57906=CARTESIAN_POINT('Ctrl Pts',(0.382874935467909,-0.730255770658821,
-3.50776196439537));
#57907=CARTESIAN_POINT('Ctrl Pts',(0.68515618301796,-0.458724004285021,
-3.49191259410039));
#57908=CARTESIAN_POINT('Ctrl Pts',(0.821049445347924,-0.0757925816733543,
-3.47606322380541));
#57909=CARTESIAN_POINT('Ctrl Pts',(0.75755347869802,0.325544826440259,-3.46021385351043));
#57910=CARTESIAN_POINT('Ctrl Pts',(0.510088075322107,0.647824715936081,
-3.44436448321545));
#57911=CARTESIAN_POINT('Ctrl Pts',(0.138749416059389,0.812782447317181,
-3.42851511292047));
#57912=CARTESIAN_POINT('Ctrl Pts',(-0.26628409463647,0.780358563795485,
-3.41266574262549));
#57913=CARTESIAN_POINT('Ctrl Pts',(-0.606651365548571,0.558427101611629,
-3.39681637233051));
#57914=CARTESIAN_POINT('Ctrl Pts',(-0.799695294729937,0.200883405799385,
-3.38096700203553));
#57915=CARTESIAN_POINT('Ctrl Pts',(-0.798535782074509,-0.205444181921911,
-3.36511763174055));
#57916=CARTESIAN_POINT('Ctrl Pts',(-0.603454411517097,-0.561880307858081,
-3.34926826144557));
#57917=CARTESIAN_POINT('Ctrl Pts',(-0.261826069280859,-0.781865600076974,
-3.33341889115059));
#57918=CARTESIAN_POINT('Ctrl Pts',(0.143385895557981,-0.81197733471658,
-3.31756952085561));
#57919=CARTESIAN_POINT('Ctrl Pts',(0.513777054757662,-0.64490297343331,
-3.30172015056063));
#57920=CARTESIAN_POINT('Ctrl Pts',(0.759399101235821,-0.321215989920727,
-3.28587078026565));
#57921=CARTESIAN_POINT('Ctrl Pts',(0.82060350744503,0.0804772682652918,
-3.27002140997067));
#57922=CARTESIAN_POINT('Ctrl Pts',(0.682526979303457,0.462626879527595,
-3.25417203967569));
#57923=CARTESIAN_POINT('Ctrl Pts',(0.378700959572816,0.73242903434883,-3.23832266938071));
#57924=CARTESIAN_POINT('Ctrl Pts',(-0.017091375654309,0.824363143291098,
-3.22247329908572));
#57925=CARTESIAN_POINT('Ctrl Pts',(-0.408733125027448,0.716103302355065,
-3.20662392879075));
#57926=CARTESIAN_POINT('Ctrl Pts',(-0.70111534368131,0.433940067282538,
-3.19077455849577));
#57927=CARTESIAN_POINT('Ctrl Pts',(-0.823233945973712,0.0463958762724045,
-3.17492518820078));
#57928=CARTESIAN_POINT('Ctrl Pts',(-0.745432820340849,-0.352415404738813,
-3.15907581790581));
#57929=CARTESIAN_POINT('Ctrl Pts',(-0.486605721036748,-0.665643733083127,
-3.14322644761082));
#57930=CARTESIAN_POINT('Ctrl Pts',(-0.109607980407257,-0.817222612125714,
-3.12737707731585));
#57931=CARTESIAN_POINT('Ctrl Pts',(0.294007707318109,-0.77034159642076,
-3.11152770702086));
#57932=CARTESIAN_POINT('Ctrl Pts',(0.626224564683723,-0.536385590527203,
-3.09567833672589));
#57933=CARTESIAN_POINT('Ctrl Pts',(0.80636479157996,-0.172170061389141,
-3.0798289664309));
#57934=CARTESIAN_POINT('Ctrl Pts',(0.790681910683307,0.233856415898155,
-3.06397959613592));
#57935=CARTESIAN_POINT('Ctrl Pts',(0.582984459405604,0.583091611352872,
-3.04813022584094));
#57936=CARTESIAN_POINT('Ctrl Pts',(0.233711098777889,0.790724875950268,
-3.03228085554596));
#57937=CARTESIAN_POINT('Ctrl Pts',(-0.172318253885027,0.8063331361891,-3.01643148525098));
#57938=CARTESIAN_POINT('Ctrl Pts',(-0.536500670325573,0.626125976045352,
-3.000582114956));
#57939=CARTESIAN_POINT('Ctrl Pts',(-0.77039561676104,0.293866127367396,
-2.98473274466102));
#57940=CARTESIAN_POINT('Ctrl Pts',(-0.817202454341236,-0.109758169432597,
-2.96888337436604));
#57941=CARTESIAN_POINT('Ctrl Pts',(-0.665554292427307,-0.486728046212792,
-2.95303400407106));
#57942=CARTESIAN_POINT('Ctrl Pts',(-0.352278401588544,-0.745497575390258,
-2.93718463377608));
#57943=CARTESIAN_POINT('Ctrl Pts',(0.0465471711407394,-0.823225405340074,
-2.9213352634811));
#57944=CARTESIAN_POINT('Ctrl Pts',(0.434068912394584,-0.701035581430156,
-2.90548589318612));
#57945=CARTESIAN_POINT('Ctrl Pts',(0.716178408087904,-0.408601511166088,
-2.88963652289114));
#57946=CARTESIAN_POINT('Ctrl Pts',(0.824366270457982,-0.0169398721875644,
-2.87378715259615));
#57947=CARTESIAN_POINT('Ctrl Pts',(0.732359423527299,0.37883556051313,-2.85793778230118));
#57948=CARTESIAN_POINT('Ctrl Pts',(0.462501435482764,0.682611990309953,
-2.84208841200619));
#57949=CARTESIAN_POINT('Ctrl Pts',(0.0803264546818227,0.820618283866978,
-2.82623904171122));
#57950=CARTESIAN_POINT('Ctrl Pts',(-0.321355548447016,0.759340054666452,
-2.81038967141623));
#57951=CARTESIAN_POINT('Ctrl Pts',(-0.64499738556106,0.513658524467306,
-2.79454030112126));
#57952=CARTESIAN_POINT('Ctrl Pts',(-0.812003672763037,0.143236666248114,
-2.77869093082627));
#57953=CARTESIAN_POINT('Ctrl Pts',(-0.781817467931542,-0.261969757750101,
-2.7628415605313));
#57954=CARTESIAN_POINT('Ctrl Pts',(-0.561769394258834,-0.603557664861111,
-2.74699219023631));
#57955=CARTESIAN_POINT('Ctrl Pts',(-0.205297421879992,-0.798573525549128,
-2.73114281994133));
#57956=CARTESIAN_POINT('Ctrl Pts',(0.201030372075136,-0.799658362453533,
-2.71529344964635));
#57957=CARTESIAN_POINT('Ctrl Pts',(0.558538583836721,-0.606548726405558,
-2.69944407935137));
#57958=CARTESIAN_POINT('Ctrl Pts',(0.78040748885868,-0.26614067421539,-2.68359470905639));
#57959=CARTESIAN_POINT('Ctrl Pts',(0.812756933942761,0.138898788571012,
-2.66774533876141));
#57960=CARTESIAN_POINT('Ctrl Pts',(0.647730959927692,0.51020712528314,-2.65189596846643));
#57961=CARTESIAN_POINT('Ctrl Pts',(0.325405596218053,0.757613295216305,
-2.63604659817145));
#57962=CARTESIAN_POINT('Ctrl Pts',(-0.075943474640016,0.821035502154527,
-2.62019722787647));
#57963=CARTESIAN_POINT('Ctrl Pts',(-0.458849915839789,0.685071866209927,
-2.60434785758149));
#57964=CARTESIAN_POINT('Ctrl Pts',(-0.730326124136905,0.382740721039322,
-2.58849848728651));
#57965=CARTESIAN_POINT('Ctrl Pts',(-0.82444497156685,-0.0125377827652834,
-2.57264911699154));
#57966=CARTESIAN_POINT('Ctrl Pts',(-0.718349997383733,-0.404771526169174,
-2.55679974669655));
#57967=CARTESIAN_POINT('Ctrl Pts',(-0.437806026369945,-0.698707800452159,
-2.54095037640157));
#57968=CARTESIAN_POINT('Ctrl Pts',(-0.0509422636323139,-0.822965122538343,
-2.52510100610659));
#57969=CARTESIAN_POINT('Ctrl Pts',(0.348292664720002,-0.747367999609815,
-2.50925163581161));
#57970=CARTESIAN_POINT('Ctrl Pts',(0.662945834618673,-0.49027495092069,
-2.49340226551663));
#57971=CARTESIAN_POINT('Ctrl Pts',(0.816604731219499,-0.114120200177109,
-2.47755289522165));
#57972=CARTESIAN_POINT('Ctrl Pts',(0.771953783472506,0.2897482757861,-2.46170352492666));
#57973=CARTESIAN_POINT('Ctrl Pts',(0.539836331073344,0.62325231069913,-2.44585415463169));
#57974=CARTESIAN_POINT('Ctrl Pts',(0.176621354136727,0.805401517506294,
-2.43000478433671));
#57975=CARTESIAN_POINT('Ctrl Pts',(-0.229485553140592,0.791961544545119,
-2.41415541404173));
#57976=CARTESIAN_POINT('Ctrl Pts',(-0.579862628611256,0.586196246216725,
-2.39830604374674));
#57977=CARTESIAN_POINT('Ctrl Pts',(-0.789421921344748,0.238075066394829,
-2.38245667345177));
#57978=CARTESIAN_POINT('Ctrl Pts',(-0.807272628073788,-0.167861881025363,
-2.36660730315678));
#57979=CARTESIAN_POINT('Ctrl Pts',(-0.629079761824146,-0.53303410810361,
-2.35075793286181));
#57980=CARTESIAN_POINT('Ctrl Pts',(-0.29811688962143,-0.768760708713042,
-2.33490856256682));
#57981=CARTESIAN_POINT('Ctrl Pts',(0.105242714706501,-0.817796232651961,
-2.31905919227185));
#57982=CARTESIAN_POINT('Ctrl Pts',(0.483044462737151,-0.668232559935171,
-2.30320982197686));
#57983=CARTESIAN_POINT('Ctrl Pts',(0.743540409617926,-0.356390749604617,
-2.28736045168189));
#57984=CARTESIAN_POINT('Ctrl Pts',(0.823469948712349,0.0419994131651224,
-2.2715110813869));
#57985=CARTESIAN_POINT('Ctrl Pts',(0.703422447372071,0.430190152922657,
-2.25566171109193));
#57986=CARTESIAN_POINT('Ctrl Pts',(0.412551056925986,0.713910591438302,
-2.23981234079694));
#57987=CARTESIAN_POINT('Ctrl Pts',(0.0214929632234256,0.824260128642901,
-2.22396297050196));
#57988=CARTESIAN_POINT('Ctrl Pts',(-0.374784627781147,0.73444073274668,
-2.20811360020698));
#57989=CARTESIAN_POINT('Ctrl Pts',(-0.680046971925417,0.466264756456678,
-2.192264229912));
#57990=CARTESIAN_POINT('Ctrl Pts',(-0.820162086331818,0.084857876961263,
-2.17641485961702));
#57991=CARTESIAN_POINT('Ctrl Pts',(-0.761103464091417,-0.31715646625377,
-2.16056548932204));
#57992=CARTESIAN_POINT('Ctrl Pts',(-0.517213302519679,-0.642150377119893,
-2.14471611902706));
#57993=CARTESIAN_POINT('Ctrl Pts',(-0.147719546459669,-0.811200124958251,
-2.12886674873208));
#57994=CARTESIAN_POINT('Ctrl Pts',(0.257647428485322,-0.783252519774712,
-2.1130173784371));
#57995=CARTESIAN_POINT('Ctrl Pts',(0.600445550365703,-0.565094548004635,
-2.09716800814212));
#57996=CARTESIAN_POINT('Ctrl Pts',(0.79742739286384,-0.209705174587831,
-2.08131863784714));
#57997=CARTESIAN_POINT('Ctrl Pts',(0.80075654623127,0.196610429037486,-2.06546926755216));
#57998=CARTESIAN_POINT('Ctrl Pts',(0.609624536232087,0.555179819484054,
-2.04961989725718));
#57999=CARTESIAN_POINT('Ctrl Pts',(0.270447159522559,0.778925568359848,
-2.0337705269622));
#58000=CARTESIAN_POINT('Ctrl Pts',(-0.134407443951421,0.813511736946051,
-2.01792115666722));
#58001=CARTESIAN_POINT('Ctrl Pts',(-0.506621630011469,0.650539184940502,
-2.00207178637223));
#58002=CARTESIAN_POINT('Ctrl Pts',(-0.755804375339143,0.329585274787486,
-1.98622241607726));
#58003=CARTESIAN_POINT('Ctrl Pts',(-0.821442448072192,-0.0714073640719366,
-1.97037304578228));
#58004=CARTESIAN_POINT('Ctrl Pts',(-0.687595852409281,-0.455058953200669,
-1.9545236754873));
#58005=CARTESIAN_POINT('Ctrl Pts',(-0.386768805553227,-0.728200932565636,
-1.93867430519231));
#58006=CARTESIAN_POINT('Ctrl Pts',(0.00798380736379087,-0.82450164703202,
-1.92282493489733));
#58007=CARTESIAN_POINT('Ctrl Pts',(0.400797578225299,-0.720574776430087,
-1.90697556460235));
#58008=CARTESIAN_POINT('Ctrl Pts',(0.696278940500164,-0.441658628529436,
-1.89112619430737));
#58009=CARTESIAN_POINT('Ctrl Pts',(0.822671191440778,-0.055487096805885,
-1.8752768240124));
#58010=CARTESIAN_POINT('Ctrl Pts',(0.749280377592604,0.34415929871677,-1.85942745371741));
#58011=CARTESIAN_POINT('Ctrl Pts',(0.493929223113824,0.660227710485335,
-1.84357808342243));
#58012=CARTESIAN_POINT('Ctrl Pts',(0.118628938278841,0.81596193669887,-1.82772871312745));
#58013=CARTESIAN_POINT('Ctrl Pts',(-0.28548000438757,0.773542419155801,
-1.81187934283247));
#58014=CARTESIAN_POINT('Ctrl Pts',(-0.62026104204666,0.543270601871413,
-1.79602997253749));
#58015=CARTESIAN_POINT('Ctrl Pts',(-0.804413671614601,0.181067258382205,
-1.78018060224251));
#58016=CARTESIAN_POINT('Ctrl Pts',(-0.793217016626087,-0.225107689058692,
-1.76433123194753));
#58017=CARTESIAN_POINT('Ctrl Pts',(-0.589390148895294,-0.576615954968053,
-1.74848186165255));
#58018=CARTESIAN_POINT('Ctrl Pts',(-0.242431770631838,-0.788094882439194,
-1.73263249135757));
#58019=CARTESIAN_POINT('Ctrl Pts',(0.163400386904445,-0.808187491055145,
-1.71678312106259));
#58020=CARTESIAN_POINT('Ctrl Pts',(0.529551283661103,-0.632014355146631,
-1.70093375076761));
#58021=CARTESIAN_POINT('Ctrl Pts',(0.767102346713403,-0.302358556692748,
-1.68508438047263));
#58022=CARTESIAN_POINT('Ctrl Pts',(0.818365060997018,0.100724049153528,
-1.66923501017765));
#58023=CARTESIAN_POINT('Ctrl Pts',(0.670890440482616,0.479346142164072,
-1.65338563988267));
#58024=CARTESIAN_POINT('Ctrl Pts',(0.360492224573578,0.741560559334522,
-1.63753626958769));
#58025=CARTESIAN_POINT('Ctrl Pts',(-0.037450373838634,0.823689369020797,
-1.62168689929271));
#58026=CARTESIAN_POINT('Ctrl Pts',(-0.426298268873834,0.705787852753012,
-1.60583752899773));
#58027=CARTESIAN_POINT('Ctrl Pts',(-0.711620994247248,0.416488016256281,
-1.58998815870274));
#58028=CARTESIAN_POINT('Ctrl Pts',(-0.824128839656565,0.0260453985351858,
-1.57413878840777));
#58029=CARTESIAN_POINT('Ctrl Pts',(-0.736499635075034,-0.370722260827263,
-1.55828941811278));
#58030=CARTESIAN_POINT('Ctrl Pts',(-0.470013852261533,-0.677461206137155,
-1.54244004781781));
#58031=CARTESIAN_POINT('Ctrl Pts',(-0.0893867103303759,-0.819680866651678,
-1.52659067752282));
#58032=CARTESIAN_POINT('Ctrl Pts',(0.312947708003538,-0.762843653177941,
-1.51074130722784));
#58033=CARTESIAN_POINT('Ctrl Pts',(0.639283777453891,-0.520752301024987,
-1.49489193693286));
#58034=CARTESIAN_POINT('Ctrl Pts',(0.810371828427002,-0.152197919928012,
-1.47904256663788));
#58035=CARTESIAN_POINT('Ctrl Pts',(0.784663675538757,0.25331723871174,-1.4631931963429));
#58036=CARTESIAN_POINT('Ctrl Pts',(0.568402461404965,0.597315117008862,
-1.44734382604792));
#58037=CARTESIAN_POINT('Ctrl Pts',(0.214106529446551,0.796256931641343,
-1.43149445575294));
#58038=CARTESIAN_POINT('Ctrl Pts',(-0.192184487655432,0.801830299903386,
-1.41564508545796));
#58039=CARTESIAN_POINT('Ctrl Pts',(-0.551804117272192,0.612681747157521,
-1.39979571516298));
#58040=CARTESIAN_POINT('Ctrl Pts',(-0.77741988379191,0.274745393816729,
-1.383946344868));
#58041=CARTESIAN_POINT('Ctrl Pts',(-0.814241720698406,-0.12991199872464,
-1.36809697457302));
#58042=CARTESIAN_POINT('Ctrl Pts',(-0.65332756279618,-0.503020678331755,
-1.35224760427804));
#58043=CARTESIAN_POINT('Ctrl Pts',(-0.333754898112137,-0.753972396792277,
-1.33639823398306));
#58044=CARTESIAN_POINT('Ctrl Pts',(0.0668690749522735,-0.821824332782597,
-1.32054886368808));
#58045=CARTESIAN_POINT('Ctrl Pts',(0.451254107267879,-0.690098860897773,
-1.3046994933931));
#58046=CARTESIAN_POINT('Ctrl Pts',(0.726053524472037,-0.390785090222578,
-1.28885012309812));
#58047=CARTESIAN_POINT('Ctrl Pts',(0.824533167957502,0.00342958838607511,
-1.27300075280314));
#58048=CARTESIAN_POINT('Ctrl Pts',(0.722777571618828,0.396811402436126,
-1.25715138250816));
#58049=CARTESIAN_POINT('Ctrl Pts',(0.445497756222818,0.693828837926884,
-1.24130201221318));
#58050=CARTESIAN_POINT('Ctrl Pts',(0.0600302371357995,0.822352161648496,
-1.2254526419182));
#58051=CARTESIAN_POINT('Ctrl Pts',(-0.34001543283308,0.751169895944896,
-1.20960327162322));
#58052=CARTESIAN_POINT('Ctrl Pts',(-0.657489443609774,0.497568426128753,
-1.19375390132824));
#58053=CARTESIAN_POINT('Ctrl Pts',(-0.815294248174704,0.123134057156335,
-1.17790453103326));
#58054=CARTESIAN_POINT('Ctrl Pts',(-0.775107455003299,-0.281203023342284,
-1.16205516073828));
#58055=CARTESIAN_POINT('Ctrl Pts',(-0.546688298145994,-0.617250849986269,
-1.14620579044329));
#58056=CARTESIAN_POINT('Ctrl Pts',(-0.185507638486464,-0.803401284042857,
-1.13035642014831));
#58057=CARTESIAN_POINT('Ctrl Pts',(0.220722957215736,-0.794448288623288,
-1.11450704985333));
#58058=CARTESIAN_POINT('Ctrl Pts',(0.573351689475297,-0.592566069999252,
-1.09865767955836));
#58059=CARTESIAN_POINT('Ctrl Pts',(0.786743799719937,-0.24678107857121,
-1.08280830926337));
#58060=CARTESIAN_POINT('Ctrl Pts',(0.809077697221824,0.158933907636998,
-1.06695893896839));
#58061=CARTESIAN_POINT('Ctrl Pts',(0.634929666481948,0.526052303254776,
-1.05110956867341));
#58062=CARTESIAN_POINT('Ctrl Pts',(0.306590999173255,0.765420581356732,
-1.03526019837843));
#58063=CARTESIAN_POINT('Ctrl Pts',(-0.0962023106326629,0.818908922022144,
-1.01941082808345));
#58064=CARTESIAN_POINT('Ctrl Pts',(-0.475633197324806,0.673527852980943,
-1.00356145778847));
#58065=CARTESIAN_POINT('Ctrl Pts',(-0.739558084942859,0.364582701364431,
-0.987712087493491));
#58066=CARTESIAN_POINT('Ctrl Pts',(-0.823883659571175,-0.0329001919469118,
-0.971862717198511));
#58067=CARTESIAN_POINT('Ctrl Pts',(-0.70813172540735,-0.422393378984735,
-0.956013346903529));
#58068=CARTESIAN_POINT('Ctrl Pts',(-0.420412269045156,-0.709309686367555,
-0.940163976608551));
#58069=CARTESIAN_POINT('Ctrl Pts',(-0.0305970392336053,-0.823972407504445,
-0.92431460631357));
#58070=CARTESIAN_POINT('Ctrl Pts',(0.366648583589333,-0.738536067697759,
-0.908465236018589));
#58071=CARTESIAN_POINT('Ctrl Pts',(0.674854771833728,-0.473748608516987,
-0.892615865723609));
#58072=CARTESIAN_POINT('Ctrl Pts',(0.819174639507985,-0.0939128166199715,
-0.876766495428628));
#58073=CARTESIAN_POINT('Ctrl Pts',(0.764560568834973,0.30872940210041,-0.860917125133647));
#58074=CARTESIAN_POINT('Ctrl Pts',(0.524275412012708,0.636397674019507,
-0.845067754838669));
#58075=CARTESIAN_POINT('Ctrl Pts',(0.156671650023453,0.809518808439597,
-0.829218384543686));
#58076=CARTESIAN_POINT('Ctrl Pts',(-0.248979320538142,0.786050892171048,
-0.813369014248708));
#58077=CARTESIAN_POINT('Ctrl Pts',(-0.594166460296292,0.571693033539423,
-0.797519643953725));
#58078=CARTESIAN_POINT('Ctrl Pts',(-0.795062177590985,0.218501352176174,
-0.781670273658746));
#58079=CARTESIAN_POINT('Ctrl Pts',(-0.802879590710967,-0.18775268295906,
-0.765820903363765));
#58080=CARTESIAN_POINT('Ctrl Pts',(-0.615720265910071,-0.5484115801897,
-0.749971533068785));
#58081=CARTESIAN_POINT('Ctrl Pts',(-0.279035245964017,-0.775890481091459,
-0.734122162773804));
#58082=CARTESIAN_POINT('Ctrl Pts',(0.125412590041216,-0.814946862928921,
-0.718272792478824));
#58083=CARTESIAN_POINT('Ctrl Pts',(0.499404380104624,-0.656096008424718,
-0.702423422183844));
#58084=CARTESIAN_POINT('Ctrl Pts',(0.752117415467132,-0.337914338981905,
-0.686574051888864));
#58085=CARTESIAN_POINT('Ctrl Pts',(0.822181144634913,0.0623287457386882,
-0.670724681593882));
#58086=CARTESIAN_POINT('Ctrl Pts',(0.692580815311664,0.447435494122635,
-0.654875311298904));
#58087=CARTESIAN_POINT('Ctrl Pts',(0.394789452515422,0.723883965370905,
-0.639025941003921));
#58088=CARTESIAN_POINT('Ctrl Pts',(0.00112473522419552,0.824539533381638,
-0.623176570708943));
#58089=CARTESIAN_POINT('Ctrl Pts',(-0.392813120415017,0.72495831574536,
-0.607327200413961));
#58090=CARTESIAN_POINT('Ctrl Pts',(-0.691357567481951,0.449323292322997,
-0.591477830118982));
#58091=CARTESIAN_POINT('Ctrl Pts',(-0.822008042894706,0.0645715460164029,
-0.575628459824001));
#58092=CARTESIAN_POINT('Ctrl Pts',(-0.753036497019803,-0.335861193493211,
-0.559779089529021));
#58093=CARTESIAN_POINT('Ctrl Pts',(-0.501192448937833,-0.654731117533164,
-0.543929719234039));
#58094=CARTESIAN_POINT('Ctrl Pts',(-0.127635419363948,-0.814601686017354,
-0.52808034893906));
#58095=CARTESIAN_POINT('Ctrl Pts',(0.276917463135748,-0.776648843267691,
-0.512230978644079));
#58096=CARTESIAN_POINT('Ctrl Pts',(0.614221826355172,-0.550089315627309,
-0.496381608349099));
#58097=CARTESIAN_POINT('Ctrl Pts',(0.802364385677912,-0.189942358978986,
-0.480532238054119));
#58098=CARTESIAN_POINT('Ctrl Pts',(0.795655322971835,0.21633149138468,-0.464682867759138));
#58099=CARTESIAN_POINT('Ctrl Pts',(0.595723912635665,0.570069931721507,
-0.448833497464158));
#58100=CARTESIAN_POINT('Ctrl Pts',(0.251122857519761,0.785368714407362,
-0.432984127169178));
#58101=CARTESIAN_POINT('Ctrl Pts',(-0.154462579487725,0.809943219413749,
-0.417134756874197));
#58102=CARTESIAN_POINT('Ctrl Pts',(-0.522537273638433,0.637825606889401,
-0.401285386579217));
#58103=CARTESIAN_POINT('Ctrl Pts',(-0.763715463943447,0.310814087932593,
-0.385436016284235));
#58104=CARTESIAN_POINT('Ctrl Pts',(-0.819427799150836,-0.091677637089383,
-0.369586645989256));
#58105=CARTESIAN_POINT('Ctrl Pts',(-0.676144716934526,-0.471905741510971,
-0.353737275694275));
#58106=CARTESIAN_POINT('Ctrl Pts',(-0.368662055243155,-0.737533047508205,
-0.337887905399296));
#58107=CARTESIAN_POINT('Ctrl Pts',(0.0283490064307482,-0.82405281449032,
-0.322038535104314));
#58108=CARTESIAN_POINT('Ctrl Pts',(0.418475602153286,-0.710453993719867,
-0.306189164809335));
#58109=CARTESIAN_POINT('Ctrl Pts',(0.706976738775498,-0.424323695776988,
-0.290339794514353));
#58110=CARTESIAN_POINT('Ctrl Pts',(0.82379083605636,-0.0351477460453753,
-0.274490424219374));
#58111=CARTESIAN_POINT('Ctrl Pts',(0.740549970253167,0.362563719550915,
-0.258641053924393));
#58112=CARTESIAN_POINT('Ctrl Pts',(0.477468907819966,0.6722277500993,-0.242791683629412));
#58113=CARTESIAN_POINT('Ctrl Pts',(0.0984360645185036,0.818643417281081,
-0.226942313334432));
#58114=CARTESIAN_POINT('Ctrl Pts',(-0.304501690502851,0.766254164680306,
-0.211092943039452));
#58115=CARTESIAN_POINT('Ctrl Pts',(-0.633492128901577,0.527782516252492,
-0.195243572744471));
#58116=CARTESIAN_POINT('Ctrl Pts',(-0.808641141858534,0.161140623251515,
-0.179394202449491));
#58117=CARTESIAN_POINT('Ctrl Pts',(-0.787414027818169,-0.244633851326282,
-0.16354483215451));
#58118=CARTESIAN_POINT('Ctrl Pts',(-0.574966358880064,-0.590999588154458,
-0.147695461859531));
#58119=CARTESIAN_POINT('Ctrl Pts',(-0.222889127189683,-0.793843339715672,
-0.131846091564549));
#58120=CARTESIAN_POINT('Ctrl Pts',(0.183314403237236,-0.803904048814602,
-0.11599672126957));
#58121=CARTESIAN_POINT('Ctrl Pts',(0.545003774088144,-0.618740661204861,
-0.100147350974589));
#58122=CARTESIAN_POINT('Ctrl Pts',(0.774334543703527,-0.28331528999698,
-0.0842979806796076));
#58123=CARTESIAN_POINT('Ctrl Pts',(0.815632750016524,0.120906817907845,
-0.0684486103846281));
#58124=CARTESIAN_POINT('Ctrl Pts',(0.658833433773886,0.495777831801544,
-0.0525992400896487));
#58125=CARTESIAN_POINT('Ctrl Pts',(0.342085277681465,0.750229523914293,
-0.0367498697946663));
#58126=CARTESIAN_POINT('Ctrl Pts',(-0.05783206721409,0.822534563742525,
-0.0209004994996869));
#58127=CARTESIAN_POINT('Ctrl Pts',(-0.314931867400366,0.737493998316566,
-0.0103342526363675));
#58128=CARTESIAN_POINT('Ctrl Pts',(-0.425612326351242,0.666853325445622,
-0.00505112920470729));
#58129=CARTESIAN_POINT('Ctrl Pts',(-0.791044518748003,1.1964098827608E-5,
-0.173133150823703));
#58130=CARTESIAN_POINT('Ctrl Pts',(-0.79100173359616,-0.0794357270706935,
-0.169937044600639));
#58131=CARTESIAN_POINT('Ctrl Pts',(-0.779104790250919,-0.158895943316062,
-0.166740938377575));
#58132=CARTESIAN_POINT('Ctrl Pts',(-0.755543935335212,-0.234732395034678,
-0.163544832154511));
#58133=CARTESIAN_POINT('Ctrl Pts',(-0.716598138172134,-0.360089096935673,
-0.158261708722851));
#58134=CARTESIAN_POINT('Ctrl Pts',(-0.645782248526095,-0.47554434254507,
-0.15297858529119));
#58135=CARTESIAN_POINT('Ctrl Pts',(-0.551694765088015,-0.567079257276634,
-0.14769546185953));
#58136=CARTESIAN_POINT('Ctrl Pts',(-0.457607281649931,-0.6586141720082,
-0.14241233842787));
#58137=CARTESIAN_POINT('Ctrl Pts',(-0.340248204419803,-0.726228755861938,
-0.137129214996209));
#58138=CARTESIAN_POINT('Ctrl Pts',(-0.213868077400249,-0.761712832638628,
-0.131846091564549));
#58139=CARTESIAN_POINT('Ctrl Pts',(-0.0874879503807029,-0.797196909415316,
-0.126562968132889));
#58140=CARTESIAN_POINT('Ctrl Pts',(0.047913226428263,-0.800550479114958,
-0.121279844701229));
#58141=CARTESIAN_POINT('Ctrl Pts',(0.175895376641231,-0.771366699363157,
-0.11599672126957));
#58142=CARTESIAN_POINT('Ctrl Pts',(0.303877526854205,-0.742182919611355,
-0.110713597837909));
#58143=CARTESIAN_POINT('Ctrl Pts',(0.424440650471175,-0.680461790408108,
-0.105430474406249));
#58144=CARTESIAN_POINT('Ctrl Pts',(0.522944007215559,-0.593696997271835,
-0.100147350974589));
#58145=CARTESIAN_POINT('Ctrl Pts',(0.621447363959938,-0.506932204135567,
-0.0948642275429287));
#58146=CARTESIAN_POINT('Ctrl Pts',(0.697890953831734,-0.39512374706627,
-0.089581104111268));
#58147=CARTESIAN_POINT('Ctrl Pts',(0.74299578315313,-0.271849167214156,
-0.084297980679608));
#58148=CARTESIAN_POINT('Ctrl Pts',(0.780555172255761,-0.169196790943382,
-0.079898653786405));
#58149=CARTESIAN_POINT('Ctrl Pts',(0.796383908785544,-0.0585936748802548,
-0.0754993268932024));
#58150=CARTESIAN_POINT('Ctrl Pts',(0.789513386643969,0.0505148782186592,
-0.0710999999999996));
#58151=CARTESIAN_POINT('',(-0.392914082828325,-0.550975096793568,-3.8089));
#58152=CARTESIAN_POINT('Ctrl Pts',(-0.392914082828323,-0.55097509679357,
-3.8089));
#58153=CARTESIAN_POINT('Ctrl Pts',(-0.40918120771343,-0.541286508891915,
-3.8089));
#58154=CARTESIAN_POINT('Ctrl Pts',(-0.425015397297533,-0.530925220216701,
-3.8089));
#58155=CARTESIAN_POINT('Ctrl Pts',(-0.440371919198835,-0.519915908540044,
-3.8089));
#58156=CARTESIAN_POINT('Ctrl Pts',(-0.463863529910594,-0.503074434554289,
-3.8089));
#58157=CARTESIAN_POINT('Ctrl Pts',(-0.486238252705378,-0.484717838355465,
-3.8089));
#58158=CARTESIAN_POINT('Ctrl Pts',(-0.507401942220326,-0.464998685887743,
-3.8089));
#58159=CARTESIAN_POINT('Ctrl Pts',(-0.515792943867532,-0.457180415792574,
-3.8089));
#58160=CARTESIAN_POINT('Ctrl Pts',(-0.523993416640949,-0.449147646509594,
-3.8089));
#58161=CARTESIAN_POINT('Ctrl Pts',(-0.531996773114634,-0.440908761680904,
-3.8089));
#58162=CARTESIAN_POINT('Ctrl Pts',(-0.538443563678603,-0.434272250468907,
-3.8089));
#58163=CARTESIAN_POINT('Ctrl Pts',(-0.544756551181799,-0.427507946632577,
-3.8089));
#58164=CARTESIAN_POINT('Ctrl Pts',(-0.550928946975755,-0.420625294631357,
-3.8089));
#58165=CARTESIAN_POINT('Ctrl Pts',(-0.573001593541319,-0.396012753548773,
-3.8089));
#58166=CARTESIAN_POINT('Ctrl Pts',(-0.593294908866083,-0.369873018445606,
-3.8089));
#58167=CARTESIAN_POINT('Ctrl Pts',(-0.611667100237218,-0.342421230741072,
-3.8089));
#58168=CARTESIAN_POINT('Ctrl Pts',(-0.619162124335873,-0.331222141517567,
-3.8089));
#58169=CARTESIAN_POINT('Ctrl Pts',(-0.62633709313012,-0.319804236221353,
-3.8089));
#58170=CARTESIAN_POINT('Ctrl Pts',(-0.633180820484676,-0.308180442575769,
-3.8089));
#58171=CARTESIAN_POINT('Ctrl Pts',(-0.63932108837351,-0.297751446332822,
-3.8089));
#58172=CARTESIAN_POINT('Ctrl Pts',(-0.64519767546254,-0.287150351905675,
-3.8089));
#58173=CARTESIAN_POINT('Ctrl Pts',(-0.650785040045425,-0.276419954666599,
-3.8089));
#58174=CARTESIAN_POINT('Ctrl Pts',(-0.654235318101704,-0.269793779914632,
-3.8089));
#58175=CARTESIAN_POINT('Ctrl Pts',(-0.657576472430511,-0.263116566740529,
-3.8089));
#58176=CARTESIAN_POINT('Ctrl Pts',(-0.660807074331226,-0.256390831914409,
-3.8089));
#58177=CARTESIAN_POINT('Ctrl Pts',(-0.675536657386884,-0.225725564952934,
-3.8089));
#58178=CARTESIAN_POINT('Ctrl Pts',(-0.68797141621589,-0.194054477335829,
-3.8089));
#58179=CARTESIAN_POINT('Ctrl Pts',(-0.698114300840514,-0.161654804678165,
-3.8089));
#58180=CARTESIAN_POINT('Ctrl Pts',(-0.704963477685347,-0.139776306010412,
-3.8089));
#58181=CARTESIAN_POINT('Ctrl Pts',(-0.710766765544529,-0.117564703199071,
-3.8089));
#58182=CARTESIAN_POINT('Ctrl Pts',(-0.715513681283513,-0.0950982670235596,
-3.8089));
#58183=CARTESIAN_POINT('Ctrl Pts',(-0.719157231569141,-0.0778538931089195,
-3.8089));
#58184=CARTESIAN_POINT('Ctrl Pts',(-0.722178239005175,-0.0604592545141676,
-3.8089));
#58185=CARTESIAN_POINT('Ctrl Pts',(-0.72456797160588,-0.0429485118438729,
-3.8089));
#58186=CARTESIAN_POINT('Ctrl Pts',(-0.725925391688996,-0.0330020292274042,
-3.8089));
#58187=CARTESIAN_POINT('Ctrl Pts',(-0.727079334996212,-0.0230129598479465,
-3.8089));
#58188=CARTESIAN_POINT('Ctrl Pts',(-0.728025398727401,-0.0130183828336468,
-3.8089));
#58189=CARTESIAN_POINT('Ctrl Pts',(-0.731393629154257,0.0225648842268292,
-3.8089));
#58190=CARTESIAN_POINT('Ctrl Pts',(-0.732142255374346,0.0582803512346346,
-3.8089));
#58191=CARTESIAN_POINT('Ctrl Pts',(-0.730254992650321,0.0938353307035594,
-3.8089));
#58192=CARTESIAN_POINT('Ctrl Pts',(-0.72860412584696,0.124936742580253,
-3.8089));
#58193=CARTESIAN_POINT('Ctrl Pts',(-0.724935845899013,0.15591642275622,
-3.8089));
#58194=CARTESIAN_POINT('Ctrl Pts',(-0.719327670522454,0.186600715052318,
-3.8089));
#58195=CARTESIAN_POINT('Ctrl Pts',(-0.716083605646998,0.204350130536374,
-3.8089));
#58196=CARTESIAN_POINT('Ctrl Pts',(-0.712189804953552,0.222000777314424,
-3.8089));
#58197=CARTESIAN_POINT('Ctrl Pts',(-0.707656253686562,0.23951869490032,
-3.8089));
#58198=CARTESIAN_POINT('Ctrl Pts',(-0.7049639395012,0.249921960516378,-3.8089));
#58199=CARTESIAN_POINT('Ctrl Pts',(-0.702043919906257,0.260284226662841,
-3.8089));
#58200=CARTESIAN_POINT('Ctrl Pts',(-0.69890838365347,0.270565505236912,
-3.8089));
#58201=CARTESIAN_POINT('Ctrl Pts',(-0.688429596994019,0.30492496278372,
-3.8089));
#58202=CARTESIAN_POINT('Ctrl Pts',(-0.675536134189328,0.338436818685454,
-3.8089));
#58203=CARTESIAN_POINT('Ctrl Pts',(-0.660358260231301,0.37084656623089,
-3.8089));
#58204=CARTESIAN_POINT('Ctrl Pts',(-0.648063055903144,0.397100867024078,
-3.8089));
#58205=CARTESIAN_POINT('Ctrl Pts',(-0.634267661582395,0.422632407626466,
-3.8089));
#58206=CARTESIAN_POINT('Ctrl Pts',(-0.619016563283335,0.447302153870391,
-3.8089));
#58207=CARTESIAN_POINT('Ctrl Pts',(-0.610140667155518,0.46165955298139,
-3.8089));
#58208=CARTESIAN_POINT('Ctrl Pts',(-0.600771307583703,0.475724949322109,
-3.8089));
#58209=CARTESIAN_POINT('Ctrl Pts',(-0.590928823493088,0.48948061897489,
-3.8089));
#58210=CARTESIAN_POINT('Ctrl Pts',(-0.585588676888875,0.49694390689171,
-3.8089));
#58211=CARTESIAN_POINT('Ctrl Pts',(-0.580109216265542,0.504315997059902,
-3.8089));
#58212=CARTESIAN_POINT('Ctrl Pts',(-0.574493428009887,0.511593875250418,
-3.8089));
#58213=CARTESIAN_POINT('Ctrl Pts',(-0.569979146106706,0.517444237178845,
-3.8089));
#58214=CARTESIAN_POINT('Ctrl Pts',(-0.565377157064798,0.523233006723831,
-3.8089));
#58215=CARTESIAN_POINT('Ctrl Pts',(-0.560697658032463,0.528948601785265,
-3.8089));
#58216=CARTESIAN_POINT('Ctrl Pts',(-0.53768323827103,0.557058684300788,
-3.8089));
#58217=CARTESIAN_POINT('Ctrl Pts',(-0.512747626910434,0.583466684665809,
-3.8089));
#58218=CARTESIAN_POINT('Ctrl Pts',(-0.486128957191253,0.608022959642477,
-3.8089));
#58219=CARTESIAN_POINT('Ctrl Pts',(-0.459292913757588,0.632779766379819,
-3.8089));
#58220=CARTESIAN_POINT('Ctrl Pts',(-0.43074544663,0.655655429636067,-3.8089));
#58221=CARTESIAN_POINT('Ctrl Pts',(-0.400686420987431,0.676468800819551,
-3.8089));
#58222=CARTESIAN_POINT('Ctrl Pts',(-0.38173423202165,0.689591612861925,
-3.8089));
#58223=CARTESIAN_POINT('Ctrl Pts',(-0.362180310994124,0.701894004325692,
-3.8089));
#58224=CARTESIAN_POINT('Ctrl Pts',(-0.342067962509734,0.713322310757514,
-3.8089));
#58225=CARTESIAN_POINT('Ctrl Pts',(-0.392914082828325,-0.550975096793569,
-3.8089));
#58226=CARTESIAN_POINT('Ctrl Pts',(-0.316721006496901,-0.605194430403013,
-3.8045006731068));
#58227=CARTESIAN_POINT('Ctrl Pts',(-0.124097906710261,-0.689702849642968,
-3.79481822278193));
#58228=CARTESIAN_POINT('Ctrl Pts',(0.203771242261294,-0.675228509254,-3.77985264902541));
#58229=CARTESIAN_POINT('Ctrl Pts',(0.501518367203066,-0.495916548685635,
-3.76400327873043));
#58230=CARTESIAN_POINT('Ctrl Pts',(0.677472975891979,-0.19617577998387,
-3.74815390843546));
#58231=CARTESIAN_POINT('Ctrl Pts',(0.688905638980991,0.15120714934306,-3.73230453814047));
#58232=CARTESIAN_POINT('Ctrl Pts',(0.533039672552928,0.46186914013689,-3.71645516784549));
#58233=CARTESIAN_POINT('Ctrl Pts',(0.24772677985824,0.66036808055943,-3.70060579755051));
#58234=CARTESIAN_POINT('Ctrl Pts',(-0.097745794456612,0.698498547043651,
-3.68475642725553));
#58235=CARTESIAN_POINT('Ctrl Pts',(-0.419481102114336,0.567000979985795,
-3.66890705696055));
#58236=CARTESIAN_POINT('Ctrl Pts',(-0.630220227894166,0.308983052482088,
-3.65371558841504));
#58237=CARTESIAN_POINT('Ctrl Pts',(-0.676650477069334,0.0982983612630573,
-3.64380724330119));
#58238=CARTESIAN_POINT('Ctrl Pts',(-0.67673605652177,-1.28860430050285E-5,
-3.639182021619));
#58239=CARTESIAN_POINT('Origin',(-1.87869726832665E-16,-4.25270154953079E-17,
-3.8089));
#58240=CARTESIAN_POINT('',(-0.7911,-9.68818082805471E-17,-3.8089));
#58241=CARTESIAN_POINT('Origin',(0.,0.,-3.8089));
#58242=CARTESIAN_POINT('Origin',(0.,0.,-3.8089));
#58243=CARTESIAN_POINT('',(0.392888236737271,-0.550964357679767,-3.8089));
#58244=CARTESIAN_POINT('Ctrl Pts',(0.342095581308743,0.713339856610552,
-3.8089));
#58245=CARTESIAN_POINT('Ctrl Pts',(0.36121279300994,0.702501567673476,-3.8089));
#58246=CARTESIAN_POINT('Ctrl Pts',(0.37984607702609,0.690878787228922,-3.8089));
#58247=CARTESIAN_POINT('Ctrl Pts',(0.397940630435775,0.678487386031165,
-3.8089));
#58248=CARTESIAN_POINT('Ctrl Pts',(0.424451217565607,0.660332568187579,
-3.8089));
#58249=CARTESIAN_POINT('Ctrl Pts',(0.449806577768339,0.640528540279525,
-3.8089));
#58250=CARTESIAN_POINT('Ctrl Pts',(0.473876877114966,0.619209890699569,
-3.8089));
#58251=CARTESIAN_POINT('Ctrl Pts',(0.483771335729022,0.610446539112668,
-3.8089));
#58252=CARTESIAN_POINT('Ctrl Pts',(0.493448376032635,0.601427032669218,
-3.8089));
#58253=CARTESIAN_POINT('Ctrl Pts',(0.502897725274963,0.592159917140135,
-3.8089));
#58254=CARTESIAN_POINT('Ctrl Pts',(0.509419954580009,0.585763471106973,
-3.8089));
#58255=CARTESIAN_POINT('Ctrl Pts',(0.515830745518692,0.579251786110235,
-3.8089));
#58256=CARTESIAN_POINT('Ctrl Pts',(0.522120551240599,0.572634917336308,
-3.8089));
#58257=CARTESIAN_POINT('Ctrl Pts',(0.547671800606227,0.545755030812409,
-3.8089));
#58258=CARTESIAN_POINT('Ctrl Pts',(0.571263889736759,0.517108988254135,
-3.8089));
#58259=CARTESIAN_POINT('Ctrl Pts',(0.592688323170684,0.486902555544426,
-3.8089));
#58260=CARTESIAN_POINT('Ctrl Pts',(0.6060488685909,0.468065445221511,-3.8089));
#58261=CARTESIAN_POINT('Ctrl Pts',(0.618565526028434,0.448620849726152,
-3.8089));
#58262=CARTESIAN_POINT('Ctrl Pts',(0.630177040564387,0.428614402836241,
-3.8089));
#58263=CARTESIAN_POINT('Ctrl Pts',(0.634151625121932,0.42176625958897,-3.8089));
#58264=CARTESIAN_POINT('Ctrl Pts',(0.638015062537283,0.414860897563193,
-3.8089));
#58265=CARTESIAN_POINT('Ctrl Pts',(0.641765273269331,0.407900970199179,
-3.8089));
#58266=CARTESIAN_POINT('Ctrl Pts',(0.644627675464558,0.402588705692247,
-3.8089));
#58267=CARTESIAN_POINT('Ctrl Pts',(0.647424172391886,0.397244548798339,
-3.8089));
#58268=CARTESIAN_POINT('Ctrl Pts',(0.650153933287359,0.391869417938239,
-3.8089));
#58269=CARTESIAN_POINT('Ctrl Pts',(0.666288679035159,0.360098734310713,
-3.8089));
#58270=CARTESIAN_POINT('Ctrl Pts',(0.680096002267384,0.327247301124806,
-3.8089));
#58271=CARTESIAN_POINT('Ctrl Pts',(0.691525041999413,0.293582472433363,
-3.8089));
#58272=CARTESIAN_POINT('Ctrl Pts',(0.702852857674015,0.260215804447685,
-3.8089));
#58273=CARTESIAN_POINT('Ctrl Pts',(0.711844433318636,0.226048834947817,
-3.8089));
#58274=CARTESIAN_POINT('Ctrl Pts',(0.71839997405433,0.191336560614048,-3.8089));
#58275=CARTESIAN_POINT('Ctrl Pts',(0.720682240379993,0.179251721545355,
-3.8089));
#58276=CARTESIAN_POINT('Ctrl Pts',(0.722668793691289,0.167100828440312,
-3.8089));
#58277=CARTESIAN_POINT('Ctrl Pts',(0.724353936498504,0.154894909635805,
-3.8089));
#58278=CARTESIAN_POINT('Ctrl Pts',(0.725348929252383,0.147687923549573,
-3.8089));
#58279=CARTESIAN_POINT('Ctrl Pts',(0.72623754978894,0.140470862544136,-3.8089));
#58280=CARTESIAN_POINT('Ctrl Pts',(0.727019157369881,0.133248004731528,
-3.8089));
#58281=CARTESIAN_POINT('Ctrl Pts',(0.730644198307119,0.0997488986672927,
-3.8089));
#58282=CARTESIAN_POINT('Ctrl Pts',(0.731972955727726,0.0661109163631112,
-3.8089));
#58283=CARTESIAN_POINT('Ctrl Pts',(0.7309415524454,0.03255904596736,-3.8089));
#58284=CARTESIAN_POINT('Ctrl Pts',(0.730024558511494,0.00272894735187942,
-3.8089));
#58285=CARTESIAN_POINT('Ctrl Pts',(0.727241148278698,-0.0270336586862393,
-3.8089));
#58286=CARTESIAN_POINT('Ctrl Pts',(0.722626861054683,-0.0565585721414304,
-3.8089));
#58287=CARTESIAN_POINT('Ctrl Pts',(0.720147537884213,-0.0724227345747074,
-3.8089));
#58288=CARTESIAN_POINT('Ctrl Pts',(0.717139169466594,-0.088218119370617,
-3.8089));
#58289=CARTESIAN_POINT('Ctrl Pts',(0.71360426348179,-0.103916722064461,
-3.8089));
#58290=CARTESIAN_POINT('Ctrl Pts',(0.712023618639872,-0.110936403911731,
-3.8089));
#58291=CARTESIAN_POINT('Ctrl Pts',(0.710337667999657,-0.117936715941189,
-3.8089));
#58292=CARTESIAN_POINT('Ctrl Pts',(0.708546509596779,-0.124915054508574,
-3.8089));
#58293=CARTESIAN_POINT('Ctrl Pts',(0.706599664866173,-0.132499945742351,
-3.8089));
#58294=CARTESIAN_POINT('Ctrl Pts',(0.704530543424124,-0.140050769984527,
-3.8089));
#58295=CARTESIAN_POINT('Ctrl Pts',(0.702341826791288,-0.147558585047062,
-3.8089));
#58296=CARTESIAN_POINT('Ctrl Pts',(0.692840226549643,-0.180151318314681,
-3.8089));
#58297=CARTESIAN_POINT('Ctrl Pts',(0.681079279247323,-0.211971147619771,
-3.8089));
#58298=CARTESIAN_POINT('Ctrl Pts',(0.66712289065792,-0.242769220807921,
-3.8089));
#58299=CARTESIAN_POINT('Ctrl Pts',(0.656934524727168,-0.265252260570885,
-3.8089));
#58300=CARTESIAN_POINT('Ctrl Pts',(0.645575103228812,-0.287190573685416,
-3.8089));
#58301=CARTESIAN_POINT('Ctrl Pts',(0.633054891849579,-0.308477498341469,
-3.8089));
#58302=CARTESIAN_POINT('Ctrl Pts',(0.624944614015227,-0.322266632404003,
-3.8089));
#58303=CARTESIAN_POINT('Ctrl Pts',(0.61634697984595,-0.335782233726575,
-3.8089));
#58304=CARTESIAN_POINT('Ctrl Pts',(0.607278987278486,-0.349001209705128,
-3.8089));
#58305=CARTESIAN_POINT('Ctrl Pts',(0.602478801187708,-0.355998739109185,
-3.8089));
#58306=CARTESIAN_POINT('Ctrl Pts',(0.597546788253189,-0.362913113695733,
-3.8089));
#58307=CARTESIAN_POINT('Ctrl Pts',(0.592485323085494,-0.369740651388275,
-3.8089));
#58308=CARTESIAN_POINT('Ctrl Pts',(0.588725489253597,-0.374812385827705,
-3.8089));
#58309=CARTESIAN_POINT('Ctrl Pts',(0.584895221083396,-0.379834711363469,
-3.8089));
#58310=CARTESIAN_POINT('Ctrl Pts',(0.581001430593434,-0.384799080112452,
-3.8089));
#58311=CARTESIAN_POINT('Ctrl Pts',(0.560423538217804,-0.411034761280424,
-3.8089));
#58312=CARTESIAN_POINT('Ctrl Pts',(0.53803152477826,-0.435713343348598,
-3.8089));
#58313=CARTESIAN_POINT('Ctrl Pts',(0.514011098046997,-0.458656110995473,
-3.8089));
#58314=CARTESIAN_POINT('Ctrl Pts',(0.490436458056322,-0.48117309180168,
-3.8089));
#58315=CARTESIAN_POINT('Ctrl Pts',(0.465292264875717,-0.50201872351403,
-3.8089));
#58316=CARTESIAN_POINT('Ctrl Pts',(0.438727568397101,-0.520982709860239,
-3.8089));
#58317=CARTESIAN_POINT('Ctrl Pts',(0.423883704104649,-0.531579436986169,
-3.8089));
#58318=CARTESIAN_POINT('Ctrl Pts',(0.40859591590594,-0.541587847856024,
-3.8089));
#58319=CARTESIAN_POINT('Ctrl Pts',(0.392888236737278,-0.550964357679762,
-3.8089));
#58320=CARTESIAN_POINT('Origin',(0.,0.,-3.8089));
#58321=CARTESIAN_POINT('Origin',(0.,0.,-4.178617978381));
#58322=CARTESIAN_POINT('Ctrl Pts',(0.392888236737271,-0.550964357679767,
-3.8089));
#58323=CARTESIAN_POINT('Ctrl Pts',(0.484334114933679,-0.485755039979474,
-3.80361687656834));
#58324=CARTESIAN_POINT('Ctrl Pts',(0.634040615230541,-0.308993274199896,
-3.79305062970502));
#58325=CARTESIAN_POINT('Ctrl Pts',(0.704605176817581,0.0314014527883039,
-3.77720125941004));
#58326=CARTESIAN_POINT('Ctrl Pts',(0.604063223483086,0.364081211703574,
-3.76135188911506));
#58327=CARTESIAN_POINT('Ctrl Pts',(0.356824591291676,0.608388806027088,
-3.74550251882008));
#58328=CARTESIAN_POINT('Ctrl Pts',(0.0229331537905069,0.704928930307171,
-3.7296531485251));
#58329=CARTESIAN_POINT('Ctrl Pts',(-0.316527984197726,0.630290638914377,
-3.71380377823012));
#58330=CARTESIAN_POINT('Ctrl Pts',(-0.57912108147644,0.402582506643355,
-3.69795440793514));
#58331=CARTESIAN_POINT('Ctrl Pts',(-0.669368670582889,0.161732571732784,
-3.68622580798543));
#58332=CARTESIAN_POINT('Ctrl Pts',(-0.676729148312702,0.0247271568507296,
-3.67978033146739));
#58333=CARTESIAN_POINT('Ctrl Pts',(-0.676703788167417,1.73951649275021E-5,
-3.678617978381));
#58334=CARTESIAN_POINT('Ctrl Pts',(0.459308237155087,-0.644108029201225,
-3.87494887079529));
#58335=CARTESIAN_POINT('Ctrl Pts',(0.566213563357509,-0.567874703897988,
-3.86966574736363));
#58336=CARTESIAN_POINT('Ctrl Pts',(0.741228802584419,-0.36123035203125,
-3.85909950050031));
#58337=CARTESIAN_POINT('Ctrl Pts',(0.823722706340163,0.0367100477328463,
-3.84325013020534));
#58338=CARTESIAN_POINT('Ctrl Pts',(0.70618356154496,0.425631220006929,-3.82740075991035));
#58339=CARTESIAN_POINT('Ctrl Pts',(0.417147826467938,0.711240408523754,
-3.81155138961537));
#58340=CARTESIAN_POINT('Ctrl Pts',(0.026810134422462,0.824101192206298,
-3.79570201932039));
#58341=CARTESIAN_POINT('Ctrl Pts',(-0.370038847788994,0.736844871353877,
-3.77985264902541));
#58342=CARTESIAN_POINT('Ctrl Pts',(-0.677024807974,0.470641378758041,-3.76400327873043));
#58343=CARTESIAN_POINT('Ctrl Pts',(-0.819597600423394,0.0901475825088134,
-3.74815390843546));
#58344=CARTESIAN_POINT('Ctrl Pts',(-0.763133668772108,-0.312240026097584,
-3.73230453814046));
#58345=CARTESIAN_POINT('Ctrl Pts',(-0.521345205358778,-0.638800245198537,
-3.7164551678455));
#58346=CARTESIAN_POINT('Ctrl Pts',(-0.152949709560969,-0.810230329040985,
-3.70060579755051));
#58347=CARTESIAN_POINT('Ctrl Pts',(0.252589124028344,-0.784898337362364,
-3.68475642725553));
#58348=CARTESIAN_POINT('Ctrl Pts',(0.596787502422859,-0.568956417209875,
-3.66890705696055));
#58349=CARTESIAN_POINT('Ctrl Pts',(0.796057944200422,-0.214845191751947,
-3.65305768666557));
#58350=CARTESIAN_POINT('Ctrl Pts',(0.802008264329106,0.19144046943575,-3.63720831637059));
#58351=CARTESIAN_POINT('Ctrl Pts',(0.613193444716271,0.551235441505258,
-3.62135894607561));
#58352=CARTESIAN_POINT('Ctrl Pts',(0.275466560722855,0.777164643436226,
-3.60550957578063));
#58353=CARTESIAN_POINT('Ctrl Pts',(-0.12915649571277,0.814361904208446,
-3.58966020548564));
#58354=CARTESIAN_POINT('Ctrl Pts',(-0.502414310616047,0.653793981871771,
-3.57381083519067));
#58355=CARTESIAN_POINT('Ctrl Pts',(-0.753662418874675,0.334454285456363,
-3.55796146489568));
#58356=CARTESIAN_POINT('Ctrl Pts',(-0.821886021785598,-0.06610656386918,
-3.54211209460071));
#58357=CARTESIAN_POINT('Ctrl Pts',(-0.690517235855899,-0.450613645538905,
-3.52626272430572));
#58358=CARTESIAN_POINT('Ctrl Pts',(-0.391458550111,-0.725690646321452,-3.51041335401075));
#58359=CARTESIAN_POINT('Ctrl Pts',(0.00266459114198865,-0.824535997108764,
-3.49456398371576));
#58360=CARTESIAN_POINT('Ctrl Pts',(0.396140644969226,-0.723145421059153,
-3.47871461342078));
#58361=CARTESIAN_POINT('Ctrl Pts',(0.69341521153958,-0.44614129487425,-3.46286524312581));
#58362=CARTESIAN_POINT('Ctrl Pts',(0.822296114184983,-0.0607931837071266,
-3.44701587283082));
#58363=CARTESIAN_POINT('Ctrl Pts',(0.751485038352033,0.339318357478879,
-3.43116650253584));
#58364=CARTESIAN_POINT('Ctrl Pts',(0.498178227082102,0.657027521987999,
-3.41531713224086));
#58365=CARTESIAN_POINT('Ctrl Pts',(0.123890428446799,0.815179656473512,
-3.39946776194588));
#58366=CARTESIAN_POINT('Ctrl Pts',(-0.280483764060795,0.775368021449757,
-3.3836183916509));
#58367=CARTESIAN_POINT('Ctrl Pts',(-0.616743372527332,0.547260745013206,
-3.36776902135592));
#58368=CARTESIAN_POINT('Ctrl Pts',(-0.80322882768251,0.186252948885433,
-3.35191965106094));
#58369=CARTESIAN_POINT('Ctrl Pts',(-0.794652733836475,-0.219985779528958,
-3.33607028076596));
#58370=CARTESIAN_POINT('Ctrl Pts',(-0.593097767920537,-0.572801665741669,
-3.32022091047098));
#58371=CARTESIAN_POINT('Ctrl Pts',(-0.247510908062826,-0.786514501442065,
-3.304371540176));
#58372=CARTESIAN_POINT('Ctrl Pts',(0.158183183330303,-0.809224808752328,
-3.28852216988102));
#58373=CARTESIAN_POINT('Ctrl Pts',(0.525462995127194,-0.63541746225667,
-3.27267279958604));
#58374=CARTESIAN_POINT('Ctrl Pts',(0.765135801000186,-0.307301019550136,
-3.25682342929106));
#58375=CARTESIAN_POINT('Ctrl Pts',(0.818997827434396,0.0954424918287849,
-3.24097405899608));
#58376=CARTESIAN_POINT('Ctrl Pts',(0.673968853767286,0.475008099657638,
-3.2251246887011));
#58377=CARTESIAN_POINT('Ctrl Pts',(0.365268701895915,0.739219511379414,
-3.20927531840612));
#58378=CARTESIAN_POINT('Ctrl Pts',(-0.0321357847028984,0.823913831617287,
-3.19342594811114));
#58379=CARTESIAN_POINT('Ctrl Pts',(-0.421736198879906,0.708523315878227,
-3.17757657781615));
#58380=CARTESIAN_POINT('Ctrl Pts',(-0.708919327486185,0.421070181448749,
-3.16172720752118));
#58381=CARTESIAN_POINT('Ctrl Pts',(-0.823943667251017,0.0313615016492279,
-3.14587783722619));
#58382=CARTESIAN_POINT('Ctrl Pts',(-0.738875925550794,-0.365963218411641,
-3.13002846693122));
#58383=CARTESIAN_POINT('Ctrl Pts',(-0.474374531085041,-0.674414942632945,
-3.11417909663623));
#58384=CARTESIAN_POINT('Ctrl Pts',(-0.094672800611489,-0.819087157397261,
-3.09832972634126));
#58385=CARTESIAN_POINT('Ctrl Pts',(0.308019916364428,-0.764846678564796,
-3.08248035604627));
#58386=CARTESIAN_POINT('Ctrl Pts',(0.635910982878394,-0.524865632751264,
-3.06663098575129));
#58387=CARTESIAN_POINT('Ctrl Pts',(0.809373103278666,-0.157422648554173,
-3.05078161545632));
#58388=CARTESIAN_POINT('Ctrl Pts',(0.786281557022114,0.248249921803872,
-3.03493224516133));
#58389=CARTESIAN_POINT('Ctrl Pts',(0.572244052181956,0.593635793505685,
-3.01908287486635));
#58390=CARTESIAN_POINT('Ctrl Pts',(0.219238911497098,0.794859113475034,
-3.00323350457137));
#58391=CARTESIAN_POINT('Ctrl Pts',(-0.187007696879292,0.803053442740053,
-2.98738413427639));
#58392=CARTESIAN_POINT('Ctrl Pts',(-0.54784008483524,0.616228814675576,
-2.97153476398142));
#58393=CARTESIAN_POINT('Ctrl Pts',(-0.775631262279306,0.279754992026522,
-2.95568539368643));
#58394=CARTESIAN_POINT('Ctrl Pts',(-0.815062871117633,-0.124656434708484,
-2.93983602339145));
#58395=CARTESIAN_POINT('Ctrl Pts',(-0.656559071397106,-0.498795445403142,
-2.92398665309647));
#58396=CARTESIAN_POINT('Ctrl Pts',(-0.338612003377769,-0.751803579239446,
-2.90813728280149));
#58397=CARTESIAN_POINT('Ctrl Pts',(0.0615659054840728,-0.822238621004071,
-2.89228791250651));
#58398=CARTESIAN_POINT('Ctrl Pts',(0.446792731322623,-0.692995646325444,
-2.87643854221153));
#58399=CARTESIAN_POINT('Ctrl Pts',(0.723517372913463,-0.395460897790348,
-2.86058917191655));
#58400=CARTESIAN_POINT('Ctrl Pts',(0.82453813707129,-0.00188973642509855,
-2.84473980162157));
#58401=CARTESIAN_POINT('Ctrl Pts',(0.725322454671599,0.392140341380372,
-2.82889043132659));
#58402=CARTESIAN_POINT('Ctrl Pts',(0.449964536513494,0.690940392847998,
-2.8130410610316));
#58403=CARTESIAN_POINT('Ctrl Pts',(0.0653341713726577,0.821947782185582,
-2.79719169073663));
#58404=CARTESIAN_POINT('Ctrl Pts',(-0.335162388097172,0.753347784355771,
-2.78134232044164));
#58405=CARTESIAN_POINT('Ctrl Pts',(-0.654265834750312,0.501799689186061,
-2.76549295014667));
#58406=CARTESIAN_POINT('Ctrl Pts',(-0.814482918281762,0.128391146174389,
-2.74964357985169));
#58407=CARTESIAN_POINT('Ctrl Pts',(-0.776905432943641,-0.276196775599218,
-2.73379420955671));
#58408=CARTESIAN_POINT('Ctrl Pts',(-0.55065895073362,-0.613711194753442,
-2.71794483926172));
#58409=CARTESIAN_POINT('Ctrl Pts',(-0.190686705453825,-0.802187815260189,
-2.70209546896675));
#58410=CARTESIAN_POINT('Ctrl Pts',(0.21559319569918,-0.795855693299335,
-2.68624609867176));
#58411=CARTESIAN_POINT('Ctrl Pts',(0.569516979569217,-0.596252564414699,
-2.67039672837679));
#58412=CARTESIAN_POINT('Ctrl Pts',(0.78513538844694,-0.251851409360799,
-2.6545473580818));
#58413=CARTESIAN_POINT('Ctrl Pts',(0.810086182109703,0.153711054071187,
-2.63869798778682));
#58414=CARTESIAN_POINT('Ctrl Pts',(0.638310140204678,0.52194528017852,-2.62284861749184));
#58415=CARTESIAN_POINT('Ctrl Pts',(0.311522524510963,0.763426766174114,
-2.60699924719686));
#58416=CARTESIAN_POINT('Ctrl Pts',(-0.090917338818336,0.819512506366401,
-2.59114987690188));
#58417=CARTESIAN_POINT('Ctrl Pts',(-0.471278217517389,0.676582258326644,
-2.5753005066069));
#58418=CARTESIAN_POINT('Ctrl Pts',(-0.737190690044681,0.369346175153063,
-2.55945113631192));
#58419=CARTESIAN_POINT('Ctrl Pts',(-0.824078763853267,-0.0275844440730886,
-2.54360176601694));
#58420=CARTESIAN_POINT('Ctrl Pts',(-0.710841948419499,-0.417816269376767,
-2.52775239572196));
#58421=CARTESIAN_POINT('Ctrl Pts',(-0.424979441806532,-0.706582751438611,
-2.51190302542698));
#58422=CARTESIAN_POINT('Ctrl Pts',(-0.0359120384624134,-0.823757874670842,
-2.496053655132));
#58423=CARTESIAN_POINT('Ctrl Pts',(0.361876488438089,-0.740886035571238,
-2.48020428483702));
#58424=CARTESIAN_POINT('Ctrl Pts',(0.671784468788094,-0.478092394923669,
-2.46435491454204));
#58425=CARTESIAN_POINT('Ctrl Pts',(0.818551741832004,-0.0991955469390545,
-2.44850554424706));
#58426=CARTESIAN_POINT('Ctrl Pts',(0.76653634523485,0.303790622012513,-2.43265617395208));
#58427=CARTESIAN_POINT('Ctrl Pts',(0.528370051515826,0.633002211094015,
-2.4168068036571));
#58428=CARTESIAN_POINT('Ctrl Pts',(0.161890782536823,0.808491239976267,
-2.40095743336211));
#58429=CARTESIAN_POINT('Ctrl Pts',(-0.243903144634621,0.78764075988111,
-2.38510806306714));
#58430=CARTESIAN_POINT('Ctrl Pts',(-0.590465974067748,0.575514243139972,
-2.36925869277216));
#58431=CARTESIAN_POINT('Ctrl Pts',(-0.793636032269693,0.223625935150573,
-2.35340932247718));
#58432=CARTESIAN_POINT('Ctrl Pts',(-0.804074121121928,-0.182569215178101,
-2.3375599521822));
#58433=CARTESIAN_POINT('Ctrl Pts',(-0.619245384167668,-0.544428016156211,
-2.32171058188722));
#58434=CARTESIAN_POINT('Ctrl Pts',(-0.284034888386214,-0.774074216576279,
-2.30586121159224));
#58435=CARTESIAN_POINT('Ctrl Pts',(0.120152570608644,-0.815738971954194,
-2.29001184129726));
#58436=CARTESIAN_POINT('Ctrl Pts',(0.495161362539197,-0.659304129849854,
-2.27416247100227));
#58437=CARTESIAN_POINT('Ctrl Pts',(0.749921802999194,-0.342759390790666,
-2.25831310070729));
#58438=CARTESIAN_POINT('Ctrl Pts',(0.822566134722329,0.0570233688650289,
-2.24246373041231));
#58439=CARTESIAN_POINT('Ctrl Pts',(0.695452914344377,0.442958185970936,
-2.22661436011733));
#58440=CARTESIAN_POINT('Ctrl Pts',(0.399451180439311,0.721322025890232,
-2.21076498982235));
#58441=CARTESIAN_POINT('Ctrl Pts',(0.0064440063389957,0.824515121371981,
-2.19491561952737));
#58442=CARTESIAN_POINT('Ctrl Pts',(-0.388128074068138,0.727477359585098,
-2.17906624923239));
#58443=CARTESIAN_POINT('Ctrl Pts',(-0.688444494407612,0.453774050281193,
-2.16321687893741));
#58444=CARTESIAN_POINT('Ctrl Pts',(-0.821574373561847,0.0698731657734796,
-2.14736750864243));
#58445=CARTESIAN_POINT('Ctrl Pts',(-0.755187546637368,-0.330996193320378,
-2.13151813834745));
#58446=CARTESIAN_POINT('Ctrl Pts',(-0.50540584199351,-0.651484186659646,
-2.11566876805247));
#58447=CARTESIAN_POINT('Ctrl Pts',(-0.132887946844688,-0.813761331209681,
-2.09981939775749));
#58448=CARTESIAN_POINT('Ctrl Pts',(0.271901360710864,-0.778419142000201,
-2.08397002746251));
#58449=CARTESIAN_POINT('Ctrl Pts',(0.610660293399487,-0.554040356521077,
-2.06812065716753));
#58450=CARTESIAN_POINT('Ctrl Pts',(0.801122329065975,-0.195114644403376,
-2.05227128687255));
#58451=CARTESIAN_POINT('Ctrl Pts',(0.797034372175622,0.211194034383928,
-2.03642191657757));
#58452=CARTESIAN_POINT('Ctrl Pts',(0.599389169970311,0.566214918128312,
-2.02057254628259));
#58453=CARTESIAN_POINT('Ctrl Pts',(0.256184226979425,0.78373232192867,-2.00472317598761));
#58454=CARTESIAN_POINT('Ctrl Pts',(-0.149234235275289,0.810922840725644,
-1.98887380569263));
#58455=CARTESIAN_POINT('Ctrl Pts',(-0.518411641315918,0.641183344088789,
-1.97302443539765));
#58456=CARTESIAN_POINT('Ctrl Pts',(-0.761694440128485,0.315734525299501,
-1.95717506510267));
#58457=CARTESIAN_POINT('Ctrl Pts',(-0.820002182971318,-0.0863894120307608,
-1.94132569480769));
#58458=CARTESIAN_POINT('Ctrl Pts',(-0.679175021186466,-0.467533957253495,
-1.92547632451271));
#58459=CARTESIAN_POINT('Ctrl Pts',(-0.373412380108861,-0.735139377921076,
-1.90962695421773));
#58460=CARTESIAN_POINT('Ctrl Pts',(0.0230322618755374,-0.824218554451213,
-1.89377758392274));
#58461=CARTESIAN_POINT('Ctrl Pts',(0.413883592808825,-0.713138894039869,
-1.87792821362777));
#58462=CARTESIAN_POINT('Ctrl Pts',(0.704224618413045,-0.428875736559846,
-1.86207884333278));
#58463=CARTESIAN_POINT('Ctrl Pts',(0.823546950242572,-0.0404614796431028,
-1.8462294730378));
#58464=CARTESIAN_POINT('Ctrl Pts',(0.742873542062324,0.357778718054223,
-1.83038010274282));
#58465=CARTESIAN_POINT('Ctrl Pts',(0.48179567274641,0.669133499618412,-1.81453073244784));
#58466=CARTESIAN_POINT('Ctrl Pts',(0.103715266931461,0.817991353251417,
-1.79868136215286));
#58467=CARTESIAN_POINT('Ctrl Pts',(-0.299552059379227,0.768202625815879,
-1.78283199185788));
#58468=CARTESIAN_POINT('Ctrl Pts',(-0.630074127184189,0.531858350354521,
-1.7669826215629));
#58469=CARTESIAN_POINT('Ctrl Pts',(-0.807584710592181,0.166353977429135,
-1.75113325126792));
#58470=CARTESIAN_POINT('Ctrl Pts',(-0.78897593278113,-0.239548926277902,
-1.73528388097294));
#58471=CARTESIAN_POINT('Ctrl Pts',(-0.578766875860324,-0.587278140233081,
-1.71943451067796));
#58472=CARTESIAN_POINT('Ctrl Pts',(-0.228006136249502,-0.792388738196929,
-1.70358514038298));
#58473=CARTESIAN_POINT('Ctrl Pts',(0.178125163512817,-0.80507026818302,
-1.687735770088));
#58474=CARTESIAN_POINT('Ctrl Pts',(0.540999337642394,-0.622243061238324,
-1.67188639979302));
#58475=CARTESIAN_POINT('Ctrl Pts',(0.77249355481297,-0.288306119187871,
-1.65603702949804));
#58476=CARTESIAN_POINT('Ctrl Pts',(0.816390185589599,0.115645040800419,
-1.64018765920306));
#58477=CARTESIAN_POINT('Ctrl Pts',(0.662029073737689,0.491512172905988,
-1.62433828890808));
#58478=CARTESIAN_POINT('Ctrl Pts',(0.346896321032574,0.748017147559341,
-1.6084889186131));
#58479=CARTESIAN_POINT('Ctrl Pts',(-0.0524790925325479,0.822868552951023,
-1.59263954831812));
#58480=CARTESIAN_POINT('Ctrl Pts',(-0.439110126505229,0.697888964943071,
-1.57679017802314));
#58481=CARTESIAN_POINT('Ctrl Pts',(-0.71910467221172,0.40342927631993,-1.56094080772816));
#58482=CARTESIAN_POINT('Ctrl Pts',(-0.824466950721903,0.010998079654113,
-1.54509143743318));
#58483=CARTESIAN_POINT('Ctrl Pts',(-0.729610070051588,-0.384103965441732,
-1.5292420671382));
#58484=CARTESIAN_POINT('Ctrl Pts',(-0.457569719956044,-0.68592759236533,
-1.51339269684322));
#58485=CARTESIAN_POINT('Ctrl Pts',(-0.0744100284292379,-0.82117589970597,
-1.49754332654823));
#58486=CARTESIAN_POINT('Ctrl Pts',(0.326819900253411,-0.75700426906795,
-1.48169395625326));
#58487=CARTESIAN_POINT('Ctrl Pts',(0.648682662580996,-0.508996575485116,
-1.46584458595827));
#58488=CARTESIAN_POINT('Ctrl Pts',(0.813014917271852,-0.137380693265803,
-1.44999521566329));
#58489=CARTESIAN_POINT('Ctrl Pts',(0.779909102438105,0.267597650443601,
-1.43414584536831));
#58490=CARTESIAN_POINT('Ctrl Pts',(0.557404859212971,0.607590761544741,
-1.41829647507333));
#58491=CARTESIAN_POINT('Ctrl Pts',(0.19953663064309,0.800032401606555,-1.40244710477835));
#58492=CARTESIAN_POINT('Ctrl Pts',(-0.206788429796264,0.798188734505283,
-1.38659773448337));
#58493=CARTESIAN_POINT('Ctrl Pts',(-0.562895582160815,0.602507488893362,
-1.37074836418839));
#58494=CARTESIAN_POINT('Ctrl Pts',(-0.782305344693098,0.260509228729736,
-1.35489899389341));
#58495=CARTESIAN_POINT('Ctrl Pts',(-0.811734759074724,-0.144752863524866,
-1.33904962359843));
#58496=CARTESIAN_POINT('Ctrl Pts',(-0.644036986251071,-0.51486218634639,
-1.32320025330345));
#58497=CARTESIAN_POINT('Ctrl Pts',(-0.319936893412746,-0.759938875714455,
-1.30735088300847));
#58498=CARTESIAN_POINT('Ctrl Pts',(0.0818588496075917,-0.820466842309713,
-1.29150151271349));
#58499=CARTESIAN_POINT('Ctrl Pts',(0.463775433098776,-0.681747063244712,
-1.27565214241851));
#58500=CARTESIAN_POINT('Ctrl Pts',(0.733065637591628,-0.377467192708359,
-1.25980277212353));
#58501=CARTESIAN_POINT('Ctrl Pts',(0.824333199146284,0.0184793769917608,
-1.24395340182855));
#58502=CARTESIAN_POINT('Ctrl Pts',(0.71541408266233,0.409938289157241,-1.22810403153357));
#58503=CARTESIAN_POINT('Ctrl Pts',(0.432758946837499,0.701845000353243,
-1.21225466123859));
#58504=CARTESIAN_POINT('Ctrl Pts',(0.0450096863933985,0.82331090040125,
-1.19640529094361));
#58505=CARTESIAN_POINT('Ctrl Pts',(-0.353670032278012,0.744838384387658,
-1.18055592064863));
#58506=CARTESIAN_POINT('Ctrl Pts',(-0.666462116001734,0.485484251570782,
-1.16470655035365));
#58507=CARTESIAN_POINT('Ctrl Pts',(-0.817406008752267,0.108231822697566,
-1.14885718005867));
#58508=CARTESIAN_POINT('Ctrl Pts',(-0.769845469471702,-0.295304357777947,
-1.13300780976369));
#58509=CARTESIAN_POINT('Ctrl Pts',(-0.535330422843599,-0.627126820481185,
-1.11715843946871));
#58510=CARTESIAN_POINT('Ctrl Pts',(-0.170812097064488,-0.806653542783506,
-1.10130906917372));
#58511=CARTESIAN_POINT('Ctrl Pts',(0.235187399575584,-0.790287034987683,
-1.08545969887875));
#58512=CARTESIAN_POINT('Ctrl Pts',(0.584072389258597,-0.582001851109171,
-1.06961032858376));
#58513=CARTESIAN_POINT('Ctrl Pts',(0.791117269310166,-0.232379381159294,
-1.05376095828878));
#58514=CARTESIAN_POINT('Ctrl Pts',(0.806041853532098,0.173675677466042,
-1.0379115879938));
#58515=CARTESIAN_POINT('Ctrl Pts',(0.625221754432068,0.537554153898595,
-1.02206221769882));
#58516=CARTESIAN_POINT('Ctrl Pts',(0.292568554121453,0.77088932521344,-1.00621284740384));
#58517=CARTESIAN_POINT('Ctrl Pts',(-0.111133982803035,0.817016492156116,
-0.990363477108863));
#58518=CARTESIAN_POINT('Ctrl Pts',(-0.487847987835832,0.664733819925901,
-0.974514106813882));
#58519=CARTESIAN_POINT('Ctrl Pts',(-0.746089671028602,0.351022667890806,
-0.958664736518902));
#58520=CARTESIAN_POINT('Ctrl Pts',(-0.82314586646374,-0.0479332151269538,
-0.942815366223922));
#58521=CARTESIAN_POINT('Ctrl Pts',(-0.700303723800595,-0.435248670325099,
-0.926965995928941));
#58522=CARTESIAN_POINT('Ctrl Pts',(-0.407395064065358,-0.716865379526681,
-0.911116625633962));
#58523=CARTESIAN_POINT('Ctrl Pts',(-0.0155518174312369,-0.824393626590682,
-0.89526725533898));
#58524=CARTESIAN_POINT('Ctrl Pts',(0.380068138271797,-0.731720521004679,
-0.879417885044));
#58525=CARTESIAN_POINT('Ctrl Pts',(0.683389763508767,-0.461351429736789,
-0.86356851474902));
#58526=CARTESIAN_POINT('Ctrl Pts',(0.820752372774903,-0.0789446209257793,
-0.84771914445404));
#58527=CARTESIAN_POINT('Ctrl Pts',(0.758797896221531,0.322633636309872,
-0.831869774159059));
#58528=CARTESIAN_POINT('Ctrl Pts',(0.51257178011198,0.645861347985452,-0.816020403864079));
#58529=CARTESIAN_POINT('Ctrl Pts',(0.141869248369509,0.812243699240455,
-0.800171033569098));
#58530=CARTESIAN_POINT('Ctrl Pts',(-0.263285776098399,0.781375268800473,
-0.784321663274118));
#58531=CARTESIAN_POINT('Ctrl Pts',(-0.604502692836885,0.560752356162417,
-0.768472292979138));
#58532=CARTESIAN_POINT('Ctrl Pts',(-0.798918066134286,0.20395252926356,
-0.752622922684157));
#58533=CARTESIAN_POINT('Ctrl Pts',(-0.799318745070129,-0.202376516345802,
-0.736773552389177));
#58534=CARTESIAN_POINT('Ctrl Pts',(-0.605607426047752,-0.559559072935617,
-0.720924182094196));
#58535=CARTESIAN_POINT('Ctrl Pts',(-0.264826282661191,-0.780854500275564,
-0.705074811799216));
#58536=CARTESIAN_POINT('Ctrl Pts',(0.140267075541125,-0.812521912386299,
-0.689225441504235));
#58537=CARTESIAN_POINT('Ctrl Pts',(0.511297023559492,-0.646870979630369,
-0.673376071209255));
#58538=CARTESIAN_POINT('Ctrl Pts',(0.758160126492153,-0.324129500641566,
-0.657526700914275));
#58539=CARTESIAN_POINT('Ctrl Pts',(0.820906470205391,0.0773257897707563,
-0.641677330619295));
#58540=CARTESIAN_POINT('Ctrl Pts',(0.684298306031528,0.460002759721218,
-0.625827960324314));
#58541=CARTESIAN_POINT('Ctrl Pts',(0.381510489244155,0.730969532323631,
-0.609978590029333));
#58542=CARTESIAN_POINT('Ctrl Pts',(-0.0139259283247104,0.824422694440805,
-0.594129219734354));
#58543=CARTESIAN_POINT('Ctrl Pts',(-0.405980478788452,0.717667444873665,
-0.578279849439372));
#58544=CARTESIAN_POINT('Ctrl Pts',(-0.699443969858383,0.43662895416746,
-0.562430479144393));
#58545=CARTESIAN_POINT('Ctrl Pts',(-0.823049732348623,0.0495565199530879,
-0.546581108849411));
#58546=CARTESIAN_POINT('Ctrl Pts',(-0.746780502601991,-0.349550556460541,
-0.530731738554432));
#58547=CARTESIAN_POINT('Ctrl Pts',(-0.489158018863314,-0.663770399438569,
-0.514882368259451));
#58548=CARTESIAN_POINT('Ctrl Pts',(-0.112745076441616,-0.816795726192998,
-0.499032997964471));
#58549=CARTESIAN_POINT('Ctrl Pts',(0.291047646798618,-0.771464826080581,
-0.48318362766949));
#58550=CARTESIAN_POINT('Ctrl Pts',(0.624160380908134,-0.5387861630555,-0.46733425737451));
#58551=CARTESIAN_POINT('Ctrl Pts',(0.805697764950427,-0.175265005428866,
-0.45148488707953));
#58552=CARTESIAN_POINT('Ctrl Pts',(0.791574026517504,0.230818697588217,
-0.435635516784549));
#58553=CARTESIAN_POINT('Ctrl Pts',(0.58521907015831,0.580848818956341,-0.419786146489568));
#58554=CARTESIAN_POINT('Ctrl Pts',(0.236745536522281,0.789821664383754,
-0.403936776194589));
#58555=CARTESIAN_POINT('Ctrl Pts',(-0.169220892912897,0.806988847559813,
-0.388087405899608));
#58556=CARTESIAN_POINT('Ctrl Pts',(-0.534092569784946,0.628181372808885,
-0.372238035604628));
#58557=CARTESIAN_POINT('Ctrl Pts',(-0.769261577206937,0.29682206327007,
-0.356388665309647));
#58558=CARTESIAN_POINT('Ctrl Pts',(-0.817617871593714,-0.106619534487822,
-0.340539295014668));
#58559=CARTESIAN_POINT('Ctrl Pts',(-0.667418287760902,-0.484168918639777,
-0.324689924719686));
#58560=CARTESIAN_POINT('Ctrl Pts',(-0.355138301822955,-0.744139433149644,
-0.308840554424707));
#58561=CARTESIAN_POINT('Ctrl Pts',(0.04338586818354,-0.823398064963412,
-0.292991184129725));
#58562=CARTESIAN_POINT('Ctrl Pts',(0.431373949250341,-0.702697120842669,
-0.277141813834746));
#58563=CARTESIAN_POINT('Ctrl Pts',(0.714604188710661,-0.411348415639086,
-0.261292443539765));
#58564=CARTESIAN_POINT('Ctrl Pts',(0.824295204963726,-0.0201050945398566,
-0.245443073244786));
#58565=CARTESIAN_POINT('Ctrl Pts',(0.733808542786668,0.376020742711894,
-0.229593702949804));
#58566=CARTESIAN_POINT('Ctrl Pts',(0.465119270428469,0.68083103233261,-0.213744332654824));
#58567=CARTESIAN_POINT('Ctrl Pts',(0.0834764010975726,0.820303909360284,
-0.197894962359843));
#58568=CARTESIAN_POINT('Ctrl Pts',(-0.318436738291248,0.760568170329218,
-0.182045592064863));
#58569=CARTESIAN_POINT('Ctrl Pts',(-0.643021878040478,0.516131744494383,
-0.166196221769882));
#58570=CARTESIAN_POINT('Ctrl Pts',(-0.811444666397369,0.146352696178963,
-0.150346851474902));
#58571=CARTESIAN_POINT('Ctrl Pts',(-0.782823541642527,-0.258964342128821,
-0.134497481179922));
#58572=CARTESIAN_POINT('Ctrl Pts',(-0.564071074017912,-0.601399186478657,
-0.118648110884941));
#58573=CARTESIAN_POINT('Ctrl Pts',(-0.20838535721098,-0.797773318333574,
-0.102798740589961));
#58574=CARTESIAN_POINT('Ctrl Pts',(0.198006948556336,-0.800437851012032,
-0.0869493702949813));
#58575=CARTESIAN_POINT('Ctrl Pts',(0.436718461990072,-0.672574504136354,
-0.0763831234316606));
#58576=CARTESIAN_POINT('Ctrl Pts',(0.533647856309012,-0.584002718706682,
-0.0711000000000004));
#58577=CARTESIAN_POINT('Ctrl Pts',(0.437168237015815,-0.613060138694073,
-3.8529325805302));
#58578=CARTESIAN_POINT('Ctrl Pts',(0.538920413882899,-0.540501482591816,
-3.84764945709854));
#58579=CARTESIAN_POINT('Ctrl Pts',(0.705499406799793,-0.343817992754132,
-3.83708321023521));
#58580=CARTESIAN_POINT('Ctrl Pts',(0.784016863165969,0.0349405160846657,
-3.82123383994024));
#58581=CARTESIAN_POINT('Ctrl Pts',(0.672143448857669,0.405114550572477,
-3.80538446964525));
#58582=CARTESIAN_POINT('Ctrl Pts',(0.397040081409184,0.676956541024866,
-3.78953509935027));
#58583=CARTESIAN_POINT('Ctrl Pts',(0.0255178075451435,0.784377104906589,
-3.7736857290553));
#58584=CARTESIAN_POINT('Ctrl Pts',(-0.352201893258571,0.701326793874043,
-3.75783635876031));
#58585=CARTESIAN_POINT('Ctrl Pts',(-0.644390232474814,0.447955088053146,
-3.74198698846533));
#58586=CARTESIAN_POINT('Ctrl Pts',(-0.780090599417017,0.0858022054224701,
-3.72613761817035));
#58587=CARTESIAN_POINT('Ctrl Pts',(-0.726348394383058,-0.297189143787908,
-3.71028824787537));
#58588=CARTESIAN_POINT('Ctrl Pts',(-0.49621484194368,-0.608008205401332,
-3.69443887758039));
#58589=CARTESIAN_POINT('Ctrl Pts',(-0.145577086304834,-0.771174857906999,
-3.67858950728541));
#58590=CARTESIAN_POINT('Ctrl Pts',(0.240413589629476,-0.747063942303056,
-3.66274013699043));
#58591=CARTESIAN_POINT('Ctrl Pts',(0.568020599681037,-0.541531054158926,
-3.64689076669545));
#58592=CARTESIAN_POINT('Ctrl Pts',(0.757685623458616,-0.204489025259539,
-3.63104139640047));
#58593=CARTESIAN_POINT('Ctrl Pts',(0.76334912075718,0.182212478999042,-3.61519202610549));
#58594=CARTESIAN_POINT('Ctrl Pts',(0.58363572758167,0.524664281302926,-3.59934265581051));
#58595=CARTESIAN_POINT('Ctrl Pts',(0.26218826697714,0.739703035039015,-3.58349328551553));
#58596=CARTESIAN_POINT('Ctrl Pts',(-0.122930774940204,0.775107279069842,
-3.56764391522055));
#58597=CARTESIAN_POINT('Ctrl Pts',(-0.478196471685247,0.622279200122251,
-3.55179454492557));
#58598=CARTESIAN_POINT('Ctrl Pts',(-0.717333686426498,0.318332610886684,
-3.53594517463059));
#58599=CARTESIAN_POINT('Ctrl Pts',(-0.782268712177764,-0.0629200341819831,
-3.52009580433561));
#58600=CARTESIAN_POINT('Ctrl Pts',(-0.657232285878265,-0.428892750140244,
-3.50424643404063));
#58601=CARTESIAN_POINT('Ctrl Pts',(-0.37258910329319,-0.690710235105353,
-3.48839706374565));
#58602=CARTESIAN_POINT('Ctrl Pts',(0.00253615005715591,-0.784790950941299,
-3.47254769345067));
#58603=CARTESIAN_POINT('Ctrl Pts',(0.377045507487883,-0.688287697143436,
-3.45669832315569));
#58604=CARTESIAN_POINT('Ctrl Pts',(0.659990570659741,-0.424635979855658,
-3.44084895286071));
#58605=CARTESIAN_POINT('Ctrl Pts',(0.782659036924308,-0.0578627744811105,
-3.42499958256572));
#58606=CARTESIAN_POINT('Ctrl Pts',(0.715261262012136,0.322962220414213,
-3.40915021227075));
#58607=CARTESIAN_POINT('Ctrl Pts',(0.474164579764779,0.625356874149369,
-3.39330084197576));
#58608=CARTESIAN_POINT('Ctrl Pts',(0.11791854751547,0.775885613284464,-3.37745147168079));
#58609=CARTESIAN_POINT('Ctrl Pts',(-0.266963626442902,0.73799301548597,
-3.3616021013858));
#58610=CARTESIAN_POINT('Ctrl Pts',(-0.58701453849155,0.520881176804586,
-3.34575273109083));
#58611=CARTESIAN_POINT('Ctrl Pts',(-0.764510849387783,0.17727501210858,
-3.32990336079584));
#58612=CARTESIAN_POINT('Ctrl Pts',(-0.756348148343323,-0.209381821673607,
-3.31405399050086));
#58613=CARTESIAN_POINT('Ctrl Pts',(-0.564508721171237,-0.545190950467224,
-3.29820462020588));
#58614=CARTESIAN_POINT('Ctrl Pts',(-0.235580158523199,-0.748602202548133,
-3.2823552499109));
#58615=CARTESIAN_POINT('Ctrl Pts',(0.150558291334779,-0.770217806636597,
-3.26650587961592));
#58616=CARTESIAN_POINT('Ctrl Pts',(0.500134142204031,-0.604788482489186,
-3.25065650932094));
#58617=CARTESIAN_POINT('Ctrl Pts',(0.728254017983114,-0.292488211798675,
-3.23480713902596));
#58618=CARTESIAN_POINT('Ctrl Pts',(0.779519737239942,0.0908418846298628,
-3.21895776873098));
#58619=CARTESIAN_POINT('Ctrl Pts',(0.641481584197075,0.452111320236231,
-3.203108398436));
#58620=CARTESIAN_POINT('Ctrl Pts',(0.347661682346383,0.703586969306436,
-3.18725902814102));
#58621=CARTESIAN_POINT('Ctrl Pts',(-0.030586745908813,0.784198775645847,
-3.17140965784604));
#58622=CARTESIAN_POINT('Ctrl Pts',(-0.401407280853592,0.674370420190166,
-3.15556028755106));
#58623=CARTESIAN_POINT('Ctrl Pts',(-0.674747342880608,0.400773367410177,
-3.13971091725608));
#58624=CARTESIAN_POINT('Ctrl Pts',(-0.784227173114788,0.0298497855624786,
-3.1238615469611));
#58625=CARTESIAN_POINT('Ctrl Pts',(-0.703259945319463,-0.348322721135155,
-3.10801217666612));
#58626=CARTESIAN_POINT('Ctrl Pts',(-0.451508291521506,-0.641906170274961,
-3.09216280637114));
#58627=CARTESIAN_POINT('Ctrl Pts',(-0.0901092947799612,-0.77960476123738,
-3.07631343607616));
#58628=CARTESIAN_POINT('Ctrl Pts',(0.293172455684328,-0.727978832094557,
-3.06046406578118));
#58629=CARTESIAN_POINT('Ctrl Pts',(0.605258213973796,-0.49956557444142,
-3.0446146954862));
#58630=CARTESIAN_POINT('Ctrl Pts',(0.770358952933123,-0.149834416558805,
-3.02876532519122));
#58631=CARTESIAN_POINT('Ctrl Pts',(0.748380486730397,0.236283549640911,
-3.01291595489624));
#58632=CARTESIAN_POINT('Ctrl Pts',(0.544660215511656,0.565020812349893,
-2.99706658460126));
#58633=CARTESIAN_POINT('Ctrl Pts',(0.208670954864866,0.756544579879811,
-2.98121721430628));
#58634=CARTESIAN_POINT('Ctrl Pts',(-0.177993379042111,0.764343918512411,
-2.96536784401129));
#58635=CARTESIAN_POINT('Ctrl Pts',(-0.521432590753099,0.586524783832913,
-2.94951847371632));
#58636=CARTESIAN_POINT('Ctrl Pts',(-0.738243567337769,0.266269983351747,
-2.93366910342133));
#58637=CARTESIAN_POINT('Ctrl Pts',(-0.775774457324241,-0.118647630035396,
-2.91781973312635));
#58638=CARTESIAN_POINT('Ctrl Pts',(-0.624911004246794,-0.474752046357884,
-2.90197036283137));
#58639=CARTESIAN_POINT('Ctrl Pts',(-0.322289914646288,-0.715564448297303,
-2.88612099253639));
#58640=CARTESIAN_POINT('Ctrl Pts',(0.0585982488088245,-0.782604315082835,
-2.87027162224141));
#58641=CARTESIAN_POINT('Ctrl Pts',(0.425256015162297,-0.659591229715815,
-2.85442225194643));
#58642=CARTESIAN_POINT('Ctrl Pts',(0.688641719830713,-0.376398526110735,
-2.83857288165145));
#58643=CARTESIAN_POINT('Ctrl Pts',(0.784792987751374,-0.00179864560344054,
-2.82272351135647));
#58644=CARTESIAN_POINT('Ctrl Pts',(0.690359791369684,0.373238030229693,
-2.80687414106149));
#58645=CARTESIAN_POINT('Ctrl Pts',(0.428274930067974,0.657635045465955,
-2.79102477076651));
#58646=CARTESIAN_POINT('Ctrl Pts',(0.0621848732624137,0.782327495545869,
-2.77517540047153));
#58647=CARTESIAN_POINT('Ctrl Pts',(-0.319006580909582,0.717034218211455,
-2.75932603017655));
#58648=CARTESIAN_POINT('Ctrl Pts',(-0.62272830831226,0.477611476805454,
-2.74347665988157));
#58649=CARTESIAN_POINT('Ctrl Pts',(-0.775222459910957,0.122202317487599,
-2.72762728958659));
#58650=CARTESIAN_POINT('Ctrl Pts',(-0.739456319250153,-0.262883283361178,
-2.71177791929161));
#58651=CARTESIAN_POINT('Ctrl Pts',(-0.524115579072248,-0.584128520553051,
-2.69592854899663));
#58652=CARTESIAN_POINT('Ctrl Pts',(-0.181495048645192,-0.763520016808344,
-2.68007917870165));
#58653=CARTESIAN_POINT('Ctrl Pts',(0.205200973229211,-0.757493121642381,
-2.66422980840667));
#58654=CARTESIAN_POINT('Ctrl Pts',(0.542064595773359,-0.567511447249129,
-2.64838043811169));
#58655=CARTESIAN_POINT('Ctrl Pts',(0.747289566832173,-0.239711434966122,
-2.63253106781671));
#58656=CARTESIAN_POINT('Ctrl Pts',(0.771037659279318,0.146301731783345,
-2.61668169752172));
#58657=CARTESIAN_POINT('Ctrl Pts',(0.607541724901335,0.49678599140238,-2.60083232722675));
#58658=CARTESIAN_POINT('Ctrl Pts',(0.296506227875872,0.726627363633215,
-2.58498295693176));
#58659=CARTESIAN_POINT('Ctrl Pts',(-0.0865348572269629,0.780009607142402,
-2.56913358663679));
#58660=CARTESIAN_POINT('Ctrl Pts',(-0.448561229322056,0.643969015014557,
-2.5532842163418));
#58661=CARTESIAN_POINT('Ctrl Pts',(-0.701655943092713,0.351542609469197,
-2.53743484604683));
#58662=CARTESIAN_POINT('Ctrl Pts',(-0.784355757665757,-0.0262547932063836,
-2.52158547575184));
#58663=CARTESIAN_POINT('Ctrl Pts',(-0.676577287862808,-0.397676303415155,
-2.50573610545686));
#58664=CARTESIAN_POINT('Ctrl Pts',(-0.404494189987261,-0.67252339663114,
-2.48988673516188));
#58665=CARTESIAN_POINT('Ctrl Pts',(-0.0341809731945969,-0.78405033628027,
-2.4740373648669));
#58666=CARTESIAN_POINT('Ctrl Pts',(0.344432983496739,-0.705173162158963,
-2.45818799457192));
#58667=CARTESIAN_POINT('Ctrl Pts',(0.639402492961459,-0.455046943451341,
-2.44233862427694));
#58668=CARTESIAN_POINT('Ctrl Pts',(0.779095154268031,-0.0944140315091314,
-2.42648925398196));
#58669=CARTESIAN_POINT('Ctrl Pts',(0.729587051890194,0.289147025687472,
-2.41063988368698));
#58670=CARTESIAN_POINT('Ctrl Pts',(0.502901069973915,0.602489653495249,
-2.394790513392));
#58671=CARTESIAN_POINT('Ctrl Pts',(0.154087173417781,0.769519598020644,
-2.37894114309702));
#58672=CARTESIAN_POINT('Ctrl Pts',(-0.232146299842057,0.74967417203701,
-2.36309177280204));
#58673=CARTESIAN_POINT('Ctrl Pts',(-0.562003787478044,0.547772773702808,
-2.34724240250706));
#58674=CARTESIAN_POINT('Ctrl Pts',(-0.7553804547651,0.212846511149716,-2.33139303221208));
#58675=CARTESIAN_POINT('Ctrl Pts',(-0.765315397211613,-0.17376884513792,
-2.3155436619171));
#58676=CARTESIAN_POINT('Ctrl Pts',(-0.589395945854437,-0.518184993761964,
-2.29969429162212));
#58677=CARTESIAN_POINT('Ctrl Pts',(-0.270343576191636,-0.736761575790739,
-2.28384492132714));
#58678=CARTESIAN_POINT('Ctrl Pts',(0.11436086535536,-0.776417968123425,
-2.26799555103216));
#58679=CARTESIAN_POINT('Ctrl Pts',(0.47129313691476,-0.627523742855025,
-2.25214618073718));
#58680=CARTESIAN_POINT('Ctrl Pts',(0.713773379174517,-0.326237385858098,
-2.23629681044219));
#58681=CARTESIAN_POINT('Ctrl Pts',(0.78291604168216,0.0542746757380962,
-2.22044744014722));
#58682=CARTESIAN_POINT('Ctrl Pts',(0.661930050230694,0.421606306109533,
-2.20459806985223));
#58683=CARTESIAN_POINT('Ctrl Pts',(0.380196465467641,0.686552194953631,
-2.18874869955726));
#58684=CARTESIAN_POINT('Ctrl Pts',(0.00613338638989894,0.784771081476074,
-2.17289932926227));
#58685=CARTESIAN_POINT('Ctrl Pts',(-0.369419165934574,0.692410823564984,
-2.1570499589673));
#58686=CARTESIAN_POINT('Ctrl Pts',(-0.655259456628897,0.431900814132295,
-2.14120058867231));
#58687=CARTESIAN_POINT('Ctrl Pts',(-0.781972086309719,0.0665050748601965,
-2.12535121837733));
#58688=CARTESIAN_POINT('Ctrl Pts',(-0.71878529857125,-0.31504120890381,
-2.10950184808236));
#58689=CARTESIAN_POINT('Ctrl Pts',(-0.481043802502479,-0.620080743793654,
-2.09365247778737));
#58690=CARTESIAN_POINT('Ctrl Pts',(-0.126482359216051,-0.774535655445814,
-2.07780310749239));
#58691=CARTESIAN_POINT('Ctrl Pts',(0.258794920031087,-0.740897063103801,
-2.06195373719741));
#58692=CARTESIAN_POINT('Ctrl Pts',(0.581224681565798,-0.527333991212848,
-2.04610436690243));
#58693=CARTESIAN_POINT('Ctrl Pts',(0.762505890164385,-0.185709547989203,
-2.03025499660745));
#58694=CARTESIAN_POINT('Ctrl Pts',(0.758614984750142,0.201013864353375,
-2.01440562631247));
#58695=CARTESIAN_POINT('Ctrl Pts',(0.570496859244902,0.538921703349788,
-1.99855625601749));
#58696=CARTESIAN_POINT('Ctrl Pts',(0.243835398105513,0.745954132222929,
-1.98270688572251));
#58697=CARTESIAN_POINT('Ctrl Pts',(-0.142040708744516,0.771833988503416,
-1.96685751542753));
#58698=CARTESIAN_POINT('Ctrl Pts',(-0.493422684266016,0.610276431956415,
-1.95100814513255));
#58699=CARTESIAN_POINT('Ctrl Pts',(-0.724978540768651,0.300515197909675,
-1.93515877483757));
#58700=CARTESIAN_POINT('Ctrl Pts',(-0.78047567990305,-0.0822251897511038,
-1.91930940454259));
#58701=CARTESIAN_POINT('Ctrl Pts',(-0.646436799122784,-0.444997453351843,
-1.90346003424761));
#58702=CARTESIAN_POINT('Ctrl Pts',(-0.355412811455735,-0.699703510211908,
-1.88761066395263));
#58703=CARTESIAN_POINT('Ctrl Pts',(0.0219220395022374,-0.784488809948108,
-1.87176129365765));
#58704=CARTESIAN_POINT('Ctrl Pts',(0.393933193357716,-0.67876351398755,
-1.85591192336267));
#58705=CARTESIAN_POINT('Ctrl Pts',(0.670278932513053,-0.408202671939927,
-1.84006255306768));
#58706=CARTESIAN_POINT('Ctrl Pts',(0.783849579026228,-0.038511118006908,
-1.82421318277271));
#58707=CARTESIAN_POINT('Ctrl Pts',(0.707064865025314,0.340532737628068,
-1.80836381247773));
#58708=CARTESIAN_POINT('Ctrl Pts',(0.458571712453908,0.636879308257715,
-1.79251444218274));
#58709=CARTESIAN_POINT('Ctrl Pts',(0.098715887781345,0.778561778055715,
-1.77666507188777));
#58710=CARTESIAN_POINT('Ctrl Pts',(-0.285112774167507,0.731173012874683,
-1.76081570159278));
#58711=CARTESIAN_POINT('Ctrl Pts',(-0.599702711792176,0.506221222608107,
-1.74496633129781));
#58712=CARTESIAN_POINT('Ctrl Pts',(-0.768656766003741,0.158335229265017,
-1.72911696100282));
#58713=CARTESIAN_POINT('Ctrl Pts',(-0.750944985698939,-0.22800196754273,
-1.71326759070784));
#58714=CARTESIAN_POINT('Ctrl Pts',(-0.550868620014696,-0.558969616556067,
-1.69741822041286));
#58715=CARTESIAN_POINT('Ctrl Pts',(-0.217015573747099,-0.754193283913979,
-1.68156885011788));
#58716=CARTESIAN_POINT('Ctrl Pts',(0.16953900975819,-0.766263527071429,
-1.6657194798229));
#58717=CARTESIAN_POINT('Ctrl Pts',(0.514921587578651,-0.592249126124486,
-1.64987010952792));
#58718=CARTESIAN_POINT('Ctrl Pts',(0.73525710654659,-0.274408921178727,
-1.63402073923294));
#58719=CARTESIAN_POINT('Ctrl Pts',(0.777037791357327,0.110070611664803,
-1.61817136893796));
#58720=CARTESIAN_POINT('Ctrl Pts',(0.630117336479189,0.467819848892825,
-1.60232199864298));
#58721=CARTESIAN_POINT('Ctrl Pts',(0.330174903965143,0.711960533696457,
-1.586472628348));
#58722=CARTESIAN_POINT('Ctrl Pts',(-0.0499494468132064,0.783203882467899,
-1.57062325805302));
#58723=CARTESIAN_POINT('Ctrl Pts',(-0.417943734362563,0.664248676067036,
-1.55477388775804));
#58724=CARTESIAN_POINT('Ctrl Pts',(-0.684441724206405,0.383982805494072,
-1.53892451746306));
#58725=CARTESIAN_POINT('Ctrl Pts',(-0.784725232792191,0.0104679400542139,
-1.52307514716808));
#58726=CARTESIAN_POINT('Ctrl Pts',(-0.694440731150519,-0.365589031111253,
-1.5072257768731));
#58727=CARTESIAN_POINT('Ctrl Pts',(-0.435513521429528,-0.652863876624973,
-1.49137640657812));
#58728=CARTESIAN_POINT('Ctrl Pts',(-0.0708232474692601,-0.781592820058913,
-1.47552703628314));
#58729=CARTESIAN_POINT('Ctrl Pts',(0.311066225374979,-0.72051444966822,
-1.45967766598816));
#58730=CARTESIAN_POINT('Ctrl Pts',(0.617414261367809,-0.484461452139772,
-1.44382829569317));
#58731=CARTESIAN_POINT('Ctrl Pts',(0.77382522084245,-0.130758542121987,
-1.4279789253982));
#58732=CARTESIAN_POINT('Ctrl Pts',(0.742315203091658,0.254698661183609,
-1.41212955510321));
#58733=CARTESIAN_POINT('Ctrl Pts',(0.53053631503652,0.578303110122371,-1.39628018480824));
#58734=CARTESIAN_POINT('Ctrl Pts',(0.189918381561399,0.761468500395673,
-1.38043081451325));
#58735=CARTESIAN_POINT('Ctrl Pts',(-0.196820622789698,0.759713703439929,
-1.36458144421828));
#58736=CARTESIAN_POINT('Ctrl Pts',(-0.53576236908232,0.57346486607728,-1.34873207392329));
#58737=CARTESIAN_POINT('Ctrl Pts',(-0.744595939462876,0.247951922124295,
-1.33288270362831));
#58738=CARTESIAN_POINT('Ctrl Pts',(-0.772606770013859,-0.137775352216883,
-1.31703333333333));
#58739=CARTESIAN_POINT('Ctrl Pts',(-0.612992520221859,-0.49004432340533,
-1.30118396303835));
#58740=CARTESIAN_POINT('Ctrl Pts',(-0.304514999591304,-0.723307599692996,
-1.28533459274337));
#58741=CARTESIAN_POINT('Ctrl Pts',(0.0779130136849949,-0.780917941302578,
-1.26948522244839));
#58742=CARTESIAN_POINT('Ctrl Pts',(0.441420101052052,-0.648884861232661,
-1.25363585215341));
#58743=CARTESIAN_POINT('Ctrl Pts',(0.697729730230368,-0.359272170230862,
-1.23778648185843));
#58744=CARTESIAN_POINT('Ctrl Pts',(0.784597928433633,0.0175886169833986,
-1.22193711156345));
#58745=CARTESIAN_POINT('Ctrl Pts',(0.680929031865307,0.390178064878987,
-1.20608774126847));
#58746=CARTESIAN_POINT('Ctrl Pts',(0.41189870012692,0.668014019002212,-1.19023837097349));
#58747=CARTESIAN_POINT('Ctrl Pts',(0.042840087891981,0.783624907477514,
-1.17438900067851));
#58748=CARTESIAN_POINT('Ctrl Pts',(-0.336622102520883,0.708934996204979,
-1.15853963038353));
#58749=CARTESIAN_POINT('Ctrl Pts',(-0.634336693143016,0.462082490992808,
-1.14269026008855));
#58750=CARTESIAN_POINT('Ctrl Pts',(-0.778004648873088,0.103014732352219,
-1.12684088979357));
#58751=CARTESIAN_POINT('Ctrl Pts',(-0.732736666662294,-0.281069824204532,
-1.11099151949859));
#58752=CARTESIAN_POINT('Ctrl Pts',(-0.509525931050183,-0.596897473890766,
-1.09514214920361));
#58753=CARTESIAN_POINT('Ctrl Pts',(-0.162578454497519,-0.767770483206364,
-1.07929277890863));
#58754=CARTESIAN_POINT('Ctrl Pts',(0.223850679181434,-0.752192888945213,
-1.06344340861365));
#58755=CARTESIAN_POINT('Ctrl Pts',(0.555918392152804,-0.55394765999684,
-1.04759403831867));
#58756=CARTESIAN_POINT('Ctrl Pts',(0.752983103545585,-0.221178015464003,
-1.03174466802369));
#58757=CARTESIAN_POINT('Ctrl Pts',(0.767188279165573,0.165304001950049,
-1.01589529772871));
#58758=CARTESIAN_POINT('Ctrl Pts',(0.595084237596002,0.511642471765704,
-1.00004592743373));
#58759=CARTESIAN_POINT('Ctrl Pts',(0.278465894284304,0.733730205504842,
-0.984196557138746));
#58760=CARTESIAN_POINT('Ctrl Pts',(-0.105776999854121,0.777633908115894,
-0.968347186843765));
#58761=CARTESIAN_POINT('Ctrl Pts',(-0.464332288257856,0.632691705991915,
-0.952497816548785));
#58762=CARTESIAN_POINT('Ctrl Pts',(-0.710125967170823,0.334102348838551,
-0.936648446253805));
#58763=CARTESIAN_POINT('Ctrl Pts',(-0.783467828658384,-0.0456226939916094,
-0.920799075958824));
#58764=CARTESIAN_POINT('Ctrl Pts',(-0.666547036486394,-0.414268411661978,
-0.904949705663843));
#58765=CARTESIAN_POINT('Ctrl Pts',(-0.387757430673421,-0.68231037197692,
-0.889100335368864));
#58766=CARTESIAN_POINT('Ctrl Pts',(-0.0148021743544479,-0.784655443098508,
-0.873250965073883));
#58767=CARTESIAN_POINT('Ctrl Pts',(0.361747742612468,-0.696449452196295,
-0.857401594778902));
#58768=CARTESIAN_POINT('Ctrl Pts',(0.650448378540411,-0.439112941740372,
-0.841552224483922));
#58769=CARTESIAN_POINT('Ctrl Pts',(0.7811897083644,-0.0751392593474202,
-0.825702854188942));
#58770=CARTESIAN_POINT('Ctrl Pts',(0.722221618748077,0.307081751594985,
-0.809853483893961));
#58771=CARTESIAN_POINT('Ctrl Pts',(0.487864321449014,0.614728942385853,
-0.794004113598982));
#58772=CARTESIAN_POINT('Ctrl Pts',(0.135030735744269,0.77309117777536,-0.778154743304));
#58773=CARTESIAN_POINT('Ctrl Pts',(-0.250594631790622,0.743710695948,-0.762305373009021));
#58774=CARTESIAN_POINT('Ctrl Pts',(-0.575363895356359,0.533722452844257,
-0.746456002714039));
#58775=CARTESIAN_POINT('Ctrl Pts',(-0.760407879151704,0.194121420955399,
-0.730606632419061));
#58776=CARTESIAN_POINT('Ctrl Pts',(-0.760789244191175,-0.192621376468859,
-0.714757262124078));
#58777=CARTESIAN_POINT('Ctrl Pts',(-0.576415377195997,-0.532586689358392,
-0.698907891829099));
#58778=CARTESIAN_POINT('Ctrl Pts',(-0.252060881432333,-0.743215029988824,
-0.683058521534118));
#58779=CARTESIAN_POINT('Ctrl Pts',(0.133505792331293,-0.773355980234025,
-0.667209151239137));
#58780=CARTESIAN_POINT('Ctrl Pts',(0.486651011890002,-0.615689906833116,
-0.651359780944158));
#58781=CARTESIAN_POINT('Ctrl Pts',(0.721614591384625,-0.30850551089168,
-0.635510410649176));
#58782=CARTESIAN_POINT('Ctrl Pts',(0.781336377848125,0.0735984605878615,
-0.619661040354197));
#58783=CARTESIAN_POINT('Ctrl Pts',(0.651313126656813,0.437829281563337,
-0.603811670059216));
#58784=CARTESIAN_POINT('Ctrl Pts',(0.36312056805023,0.695734663365716,-0.587962299764236));
#58785=CARTESIAN_POINT('Ctrl Pts',(-0.0132546578572862,0.784683109793256,
-0.572112929469256));
#58786=CARTESIAN_POINT('Ctrl Pts',(-0.386411032543397,0.683073775428778,
-0.556263559174275));
#58787=CARTESIAN_POINT('Ctrl Pts',(-0.665728725198291,0.415582161786907,
-0.540414188879295));
#58788=CARTESIAN_POINT('Ctrl Pts',(-0.783376328488732,0.0471677507782503,
-0.524564818584314));
#58789=CARTESIAN_POINT('Ctrl Pts',(-0.710783498642241,-0.332701197483979,
-0.508715448289334));
#58790=CARTESIAN_POINT('Ctrl Pts',(-0.465579171959016,-0.63177472518931,
-0.492866077994354));
#58791=CARTESIAN_POINT('Ctrl Pts',(-0.107310434068157,-0.777423783717762,
-0.477016707699373));
#58792=CARTESIAN_POINT('Ctrl Pts',(0.277018299141874,-0.734277965547306,
-0.461167337404393));
#58793=CARTESIAN_POINT('Ctrl Pts',(0.594074025379593,-0.5128150944786,-0.445317967109412));
#58794=CARTESIAN_POINT('Ctrl Pts',(0.766860776659725,-0.166816719657547,
-0.429468596814432));
#58795=CARTESIAN_POINT('Ctrl Pts',(0.753417843719877,0.219692561404809,
-0.413619226519451));
#58796=CARTESIAN_POINT('Ctrl Pts',(0.557009799680024,0.552850207365477,
-0.397769856224471));
#58797=CARTESIAN_POINT('Ctrl Pts',(0.225333709370989,0.751749950565232,
-0.381920485929491));
#58798=CARTESIAN_POINT('Ctrl Pts',(-0.16106395103904,0.768089625311954,
-0.36607111563451));
#58799=CARTESIAN_POINT('Ctrl Pts',(-0.508347746128691,0.597901193712546,
-0.35022174533953));
#58800=CARTESIAN_POINT('Ctrl Pts',(-0.732180919712112,0.282514371853855,
-0.33437237504455));
#58801=CARTESIAN_POINT('Ctrl Pts',(-0.778206299306046,-0.101480161148845,
-0.31852300474957));
#58802=CARTESIAN_POINT('Ctrl Pts',(-0.635246774627353,-0.460830560955378,
-0.302673634454589));
#58803=CARTESIAN_POINT('Ctrl Pts',(-0.33801959718024,-0.708269736460514,
-0.286824264159609));
#58804=CARTESIAN_POINT('Ctrl Pts',(0.0412945424682123,-0.783707870452892,
-0.270974893864628));
#58805=CARTESIAN_POINT('Ctrl Pts',(0.410580463473477,-0.668825064792273,
-0.255125523569648));
#58806=CARTESIAN_POINT('Ctrl Pts',(0.680158177170402,-0.39152021914091,
-0.239276153274668));
#58807=CARTESIAN_POINT('Ctrl Pts',(0.784561765681778,-0.0191359701917467,
-0.223426782979687));
#58808=CARTESIAN_POINT('Ctrl Pts',(0.698436825222601,0.357895443353941,
-0.207577412684706));
#58809=CARTESIAN_POINT('Ctrl Pts',(0.442699161492799,0.648012985689183,
-0.191728042389726));
#58810=CARTESIAN_POINT('Ctrl Pts',(0.0794525944631093,0.780762862197761,
-0.175878672094745));
#58811=CARTESIAN_POINT('Ctrl Pts',(-0.303087156333423,0.72390656046714,
-0.160029301799766));
#58812=CARTESIAN_POINT('Ctrl Pts',(-0.612026343195399,0.491252685138143,
-0.144179931504784));
#58813=CARTESIAN_POINT('Ctrl Pts',(-0.772330660651845,0.139298068258817,
-0.128330561209805));
#58814=CARTESIAN_POINT('Ctrl Pts',(-0.745089157804027,-0.246481503575108,
-0.112481190914824));
#58815=CARTESIAN_POINT('Ctrl Pts',(-0.53688119879453,-0.572409987079866,
-0.0966318206198436));
#58816=CARTESIAN_POINT('Ctrl Pts',(-0.198340573633284,-0.759318311542457,
-0.0807824503248633));
#58817=CARTESIAN_POINT('Ctrl Pts',(0.188462434624327,-0.761854405954189,
-0.0649330800298836));
#58818=CARTESIAN_POINT('Ctrl Pts',(0.415667355070738,-0.640154446295708,
-0.0543668331665629));
#58819=CARTESIAN_POINT('Ctrl Pts',(0.507924469142727,-0.555852079925217,
-0.0490837097349027));
#58820=CARTESIAN_POINT('Ctrl Pts',(0.415028236876543,-0.58201224818692,
-3.8309162902651));
#58821=CARTESIAN_POINT('Ctrl Pts',(0.511627264408289,-0.513128261285645,
-3.82563316683344));
#58822=CARTESIAN_POINT('Ctrl Pts',(0.669770011015167,-0.326405633477014,
-3.81506691997012));
#58823=CARTESIAN_POINT('Ctrl Pts',(0.744311019991775,0.0331709844364849,
-3.79921754967514));
#58824=CARTESIAN_POINT('Ctrl Pts',(0.638103336170378,0.384597881138026,
-3.78336817938015));
#58825=CARTESIAN_POINT('Ctrl Pts',(0.37693233635043,0.642672673525976,-3.76751880908518));
#58826=CARTESIAN_POINT('Ctrl Pts',(0.0242254806678254,0.74465301760688,
-3.75166943879019));
#58827=CARTESIAN_POINT('Ctrl Pts',(-0.334364938728149,0.66580871639421,
-3.73582006849522));
#58828=CARTESIAN_POINT('Ctrl Pts',(-0.611755656975627,0.425268797348251,
-3.71997069820023));
#58829=CARTESIAN_POINT('Ctrl Pts',(-0.74058359841064,0.0814568283361267,
-3.70412132790526));
#58830=CARTESIAN_POINT('Ctrl Pts',(-0.689563119994008,-0.282138261478232,
-3.68827195761027));
#58831=CARTESIAN_POINT('Ctrl Pts',(-0.471084478528582,-0.577216165604128,
-3.6724225873153));
#58832=CARTESIAN_POINT('Ctrl Pts',(-0.138204463048699,-0.732119386773014,
-3.65657321702031));
#58833=CARTESIAN_POINT('Ctrl Pts',(0.228238055230608,-0.709229547243747,
-3.64072384672533));
#58834=CARTESIAN_POINT('Ctrl Pts',(0.539253696939214,-0.514105691107978,
-3.62487447643035));
#58835=CARTESIAN_POINT('Ctrl Pts',(0.719313302716812,-0.194132858767131,
-3.60902510613537));
#58836=CARTESIAN_POINT('Ctrl Pts',(0.724689977185254,0.172984488562333,
-3.59317573584039));
#58837=CARTESIAN_POINT('Ctrl Pts',(0.55407801044707,0.498093121100594,-3.57732636554541));
#58838=CARTESIAN_POINT('Ctrl Pts',(0.248909973231426,0.702241426641804,
-3.56147699525043));
#58839=CARTESIAN_POINT('Ctrl Pts',(-0.116705054167638,0.735852653931238,
-3.54562762495545));
#58840=CARTESIAN_POINT('Ctrl Pts',(-0.453978632754447,0.590764418372731,
-3.52977825466047));
#58841=CARTESIAN_POINT('Ctrl Pts',(-0.681004953978322,0.302210936317006,
-3.51392888436549));
#58842=CARTESIAN_POINT('Ctrl Pts',(-0.742651402569929,-0.0597335044947861,
-3.49807951407051));
#58843=CARTESIAN_POINT('Ctrl Pts',(-0.62394733590063,-0.407171854741584,
-3.48223014377553));
#58844=CARTESIAN_POINT('Ctrl Pts',(-0.353719656475381,-0.655729823889253,
-3.46638077348055));
#58845=CARTESIAN_POINT('Ctrl Pts',(0.00240770897232327,-0.745045904773835,
-3.45053140318557));
#58846=CARTESIAN_POINT('Ctrl Pts',(0.357950370006541,-0.653429973227718,
-3.43468203289059));
#58847=CARTESIAN_POINT('Ctrl Pts',(0.626565929779902,-0.403130664837067,
-3.41883266259561));
#58848=CARTESIAN_POINT('Ctrl Pts',(0.743021959663633,-0.0549323652550938,
-3.40298329230063));
#58849=CARTESIAN_POINT('Ctrl Pts',(0.67903748567224,0.306606083349546,-3.38713392200565));
#58850=CARTESIAN_POINT('Ctrl Pts',(0.450150932447457,0.593686226310738,
-3.37128455171067));
#58851=CARTESIAN_POINT('Ctrl Pts',(0.111946666584141,0.736591570095416,
-3.35543518141568));
#58852=CARTESIAN_POINT('Ctrl Pts',(-0.253443488825009,0.700618009522183,
-3.33958581112071));
#58853=CARTESIAN_POINT('Ctrl Pts',(-0.557285704455768,0.494501608595965,
-3.32373644082573));
#58854=CARTESIAN_POINT('Ctrl Pts',(-0.725792871093056,0.168297075331728,
-3.30788707053075));
#58855=CARTESIAN_POINT('Ctrl Pts',(-0.718043562850171,-0.198777863818256,
-3.29203770023576));
#58856=CARTESIAN_POINT('Ctrl Pts',(-0.535919674421936,-0.51758023519278,
-3.27618832994079));
#58857=CARTESIAN_POINT('Ctrl Pts',(-0.223649408983571,-0.7106899036542,
-3.2603389596458));
#58858=CARTESIAN_POINT('Ctrl Pts',(0.142933399339255,-0.731210804520864,
-3.24448958935082));
#58859=CARTESIAN_POINT('Ctrl Pts',(0.474805289280868,-0.574159502721701,
-3.22864021905584));
#58860=CARTESIAN_POINT('Ctrl Pts',(0.691372234966041,-0.277675404047213,
-3.21279084876086));
#58861=CARTESIAN_POINT('Ctrl Pts',(0.74004164704549,0.0862412774309402,
-3.19694147846588));
#58862=CARTESIAN_POINT('Ctrl Pts',(0.608994314626862,0.429214540814824,
-3.1810921081709));
#58863=CARTESIAN_POINT('Ctrl Pts',(0.330054662796853,0.667954427233457,
-3.16524273787592));
#58864=CARTESIAN_POINT('Ctrl Pts',(-0.029037707114729,0.744483719674407,
-3.14939336758094));
#58865=CARTESIAN_POINT('Ctrl Pts',(-0.381078362827277,0.640217524502105,
-3.13354399728596));
#58866=CARTESIAN_POINT('Ctrl Pts',(-0.640575358275033,0.380476553371603,
-3.11769462699098));
#58867=CARTESIAN_POINT('Ctrl Pts',(-0.744510678978556,0.0283380694757298,
-3.101845256696));
#58868=CARTESIAN_POINT('Ctrl Pts',(-0.667643965088134,-0.330682223858671,
-3.08599588640102));
#58869=CARTESIAN_POINT('Ctrl Pts',(-0.428642051957971,-0.609397397916976,
-3.07014651610604));
#58870=CARTESIAN_POINT('Ctrl Pts',(-0.0855457889484339,-0.740122365077501,
-3.05429714581106));
#58871=CARTESIAN_POINT('Ctrl Pts',(0.278324995004228,-0.691110985624318,
-3.03844777551607));
#58872=CARTESIAN_POINT('Ctrl Pts',(0.574605445069199,-0.474265516131577,
-3.0225984052211));
#58873=CARTESIAN_POINT('Ctrl Pts',(0.731344802587579,-0.142246184563437,
-3.00674903492611));
#58874=CARTESIAN_POINT('Ctrl Pts',(0.71047941643868,0.224317177477952,-2.99089966463114));
#58875=CARTESIAN_POINT('Ctrl Pts',(0.517076378841355,0.536405831194099,
-2.97505029433616));
#58876=CARTESIAN_POINT('Ctrl Pts',(0.198102998232633,0.71823004628459,-2.95920092404118));
#58877=CARTESIAN_POINT('Ctrl Pts',(-0.16897906120493,0.725634394284768,
-2.9433515537462));
#58878=CARTESIAN_POINT('Ctrl Pts',(-0.495025096670959,0.55682075299025,
-2.92750218345121));
#58879=CARTESIAN_POINT('Ctrl Pts',(-0.700855872396232,0.252784974676972,
-2.91165281315624));
#58880=CARTESIAN_POINT('Ctrl Pts',(-0.736486043530848,-0.112638825362308,
-2.89580344286125));
#58881=CARTESIAN_POINT('Ctrl Pts',(-0.593262937096482,-0.450708647312625,
-2.87995407256628));
#58882=CARTESIAN_POINT('Ctrl Pts',(-0.305967825914806,-0.67932531735516,
-2.8641047022713));
#58883=CARTESIAN_POINT('Ctrl Pts',(0.0556305921335755,-0.742970009161601,
-2.84825533197631));
#58884=CARTESIAN_POINT('Ctrl Pts',(0.403719299001972,-0.626186813106183,
-2.83240596168134));
#58885=CARTESIAN_POINT('Ctrl Pts',(0.65376606674796,-0.357336154431123,
-2.81655659138635));
#58886=CARTESIAN_POINT('Ctrl Pts',(0.745047838431459,-0.0017075547817826,
-2.80070722109137));
#58887=CARTESIAN_POINT('Ctrl Pts',(0.655397128067767,0.354335719079015,
-2.78485785079639));
#58888=CARTESIAN_POINT('Ctrl Pts',(0.406585323622455,0.624329698083909,
-2.76900848050141));
#58889=CARTESIAN_POINT('Ctrl Pts',(0.0590355751521699,0.742707208906157,
-2.75315911020644));
#58890=CARTESIAN_POINT('Ctrl Pts',(-0.302850773721993,0.680720652067139,
-2.73730973991145));
#58891=CARTESIAN_POINT('Ctrl Pts',(-0.591190781874206,0.453423264424848,
-2.72146036961647));
#58892=CARTESIAN_POINT('Ctrl Pts',(-0.735962001540153,0.116013488800808,
-2.70561099932149));
#58893=CARTESIAN_POINT('Ctrl Pts',(-0.702007205556663,-0.249569791123137,
-2.68976162902651));
#58894=CARTESIAN_POINT('Ctrl Pts',(-0.497572207410877,-0.554545846352661,
-2.67391225873153));
#58895=CARTESIAN_POINT('Ctrl Pts',(-0.17230339183656,-0.724852218356499,
-2.65806288843655));
#58896=CARTESIAN_POINT('Ctrl Pts',(0.194808750759242,-0.719130549985429,
-2.64221351814157));
#58897=CARTESIAN_POINT('Ctrl Pts',(0.514612211977501,-0.538770330083558,
-2.62636414784659));
#58898=CARTESIAN_POINT('Ctrl Pts',(0.709443745217406,-0.227571460571446,
-2.61051477755161));
#58899=CARTESIAN_POINT('Ctrl Pts',(0.731989136448934,0.138892409495504,
-2.59466540725663));
#58900=CARTESIAN_POINT('Ctrl Pts',(0.576773309597993,0.471626702626239,
-2.57881603696165));
#58901=CARTESIAN_POINT('Ctrl Pts',(0.28148993124078,0.689827961092316,-2.56296666666667));
#58902=CARTESIAN_POINT('Ctrl Pts',(-0.0821523756355886,0.740506707918403,
-2.54711729637169));
#58903=CARTESIAN_POINT('Ctrl Pts',(-0.425844241126725,0.611355771702471,
-2.5312679260767));
#58904=CARTESIAN_POINT('Ctrl Pts',(-0.666121196140744,0.333739043785331,
-2.51541855578173));
#58905=CARTESIAN_POINT('Ctrl Pts',(-0.744632751478249,-0.0249251423396785,
-2.49956918548675));
#58906=CARTESIAN_POINT('Ctrl Pts',(-0.642312627306116,-0.377536337453543,
-2.48371981519176));
#58907=CARTESIAN_POINT('Ctrl Pts',(-0.38400893816799,-0.638464041823668,
-2.46787044489678));
#58908=CARTESIAN_POINT('Ctrl Pts',(-0.0324499079267794,-0.744342797889699,
-2.45202107460181));
#58909=CARTESIAN_POINT('Ctrl Pts',(0.326989478555387,-0.669460288746687,
-2.43617170430682));
#58910=CARTESIAN_POINT('Ctrl Pts',(0.607020517134824,-0.432001491979012,
-2.42032233401185));
#58911=CARTESIAN_POINT('Ctrl Pts',(0.739638566704057,-0.0896325160792074,
-2.40447296371686));
#58912=CARTESIAN_POINT('Ctrl Pts',(0.692637758545539,0.274503429362429,
-2.38862359342189));
#58913=CARTESIAN_POINT('Ctrl Pts',(0.477432088432004,0.571977095896485,
-2.3727742231269));
#58914=CARTESIAN_POINT('Ctrl Pts',(0.146283564298739,0.730547956065019,
-2.35692485283192));
#58915=CARTESIAN_POINT('Ctrl Pts',(-0.220389455049494,0.71170758419291,
-2.34107548253694));
#58916=CARTESIAN_POINT('Ctrl Pts',(-0.533541600888341,0.520031304265645,
-2.32522611224196));
#58917=CARTESIAN_POINT('Ctrl Pts',(-0.717124877260507,0.202067087148858,
-2.30937674194698));
#58918=CARTESIAN_POINT('Ctrl Pts',(-0.726556673301297,-0.164968475097737,
-2.293527371652));
#58919=CARTESIAN_POINT('Ctrl Pts',(-0.559546507541209,-0.491941971367719,
-2.27767800135702));
#58920=CARTESIAN_POINT('Ctrl Pts',(-0.256652263997058,-0.699448935005199,
-2.26182863106204));
#58921=CARTESIAN_POINT('Ctrl Pts',(0.108569160102076,-0.737096964292657,
-2.24597926076706));
#58922=CARTESIAN_POINT('Ctrl Pts',(0.447424911290323,-0.595743355860196,
-2.23012989047208));
#58923=CARTESIAN_POINT('Ctrl Pts',(0.677624955349841,-0.309715380925531,
-2.2142805201771));
#58924=CARTESIAN_POINT('Ctrl Pts',(0.743265948641989,0.0515259826111631,
-2.19843114988212));
#58925=CARTESIAN_POINT('Ctrl Pts',(0.628407186117013,0.400254426248131,
-2.18258177958713));
#58926=CARTESIAN_POINT('Ctrl Pts',(0.360941750495969,0.651782364017028,
-2.16673240929216));
#58927=CARTESIAN_POINT('Ctrl Pts',(0.00582276644080296,0.745027041580168,
-2.15088303899718));
#58928=CARTESIAN_POINT('Ctrl Pts',(-0.350710257801012,0.657344287544868,
-2.1350336687022));
#58929=CARTESIAN_POINT('Ctrl Pts',(-0.622074418850181,0.410027577983399,
-2.11918429840722));
#58930=CARTESIAN_POINT('Ctrl Pts',(-0.742369799057592,0.0631369839469131,
-2.10333492811223));
#58931=CARTESIAN_POINT('Ctrl Pts',(-0.68238305050513,-0.299086224487242,
-2.08748555781726));
#58932=CARTESIAN_POINT('Ctrl Pts',(-0.456681763011447,-0.588677300927662,
-2.07163618752227));
#58933=CARTESIAN_POINT('Ctrl Pts',(-0.120076771587415,-0.735309979681948,
-2.0557868172273));
#58934=CARTESIAN_POINT('Ctrl Pts',(0.245688479351311,-0.7033749842074,-2.03993744693231));
#58935=CARTESIAN_POINT('Ctrl Pts',(0.551789069732108,-0.50062762590462,
-2.02408807663734));
#58936=CARTESIAN_POINT('Ctrl Pts',(0.723889451262795,-0.17630445157503,
-2.00823870634235));
#58937=CARTESIAN_POINT('Ctrl Pts',(0.72019559732466,0.190833694322822,-1.99238933604737));
#58938=CARTESIAN_POINT('Ctrl Pts',(0.541604548519495,0.511628488571264,
-1.97653996575239));
#58939=CARTESIAN_POINT('Ctrl Pts',(0.231486569231601,0.708175942517187,
-1.96069059545741));
#58940=CARTESIAN_POINT('Ctrl Pts',(-0.134847182213743,0.732745136281187,
-1.94484122516244));
#58941=CARTESIAN_POINT('Ctrl Pts',(-0.468433727216114,0.579369519824041,
-1.92899185486745));
#58942=CARTESIAN_POINT('Ctrl Pts',(-0.688262641408817,0.285295870519851,
-1.91314248457247));
#58943=CARTESIAN_POINT('Ctrl Pts',(-0.740949176834782,-0.0780609674714476,
-1.89729311427749));
#58944=CARTESIAN_POINT('Ctrl Pts',(-0.613698577059101,-0.42246094945019,
-1.88144374398251));
#58945=CARTESIAN_POINT('Ctrl Pts',(-0.33741324280261,-0.664267642502741,
-1.86559437368753));
#58946=CARTESIAN_POINT('Ctrl Pts',(0.0208118171289387,-0.744759065445003,
-1.84974500339255));
#58947=CARTESIAN_POINT('Ctrl Pts',(0.373982793906604,-0.644388133935232,
-1.83389563309757));
#58948=CARTESIAN_POINT('Ctrl Pts',(0.636333246613063,-0.387529607320008,
-1.81804626280259));
#58949=CARTESIAN_POINT('Ctrl Pts',(0.744152207809883,-0.0365607563707129,
-1.80219689250761));
#58950=CARTESIAN_POINT('Ctrl Pts',(0.671256187988306,0.323286757201912,
-1.78634752221263));
#58951=CARTESIAN_POINT('Ctrl Pts',(0.435347752161404,0.60462511689702,-1.77049815191765));
#58952=CARTESIAN_POINT('Ctrl Pts',(0.0937165086312298,0.739132202860013,
-1.75464878162267));
#58953=CARTESIAN_POINT('Ctrl Pts',(-0.270673488955788,0.694143399933487,
-1.73879941132769));
#58954=CARTESIAN_POINT('Ctrl Pts',(-0.569331296400163,0.480584094861693,
-1.72295004103271));
#58955=CARTESIAN_POINT('Ctrl Pts',(-0.729728821415302,0.150316481100898,
-1.70710067073772));
#58956=CARTESIAN_POINT('Ctrl Pts',(-0.712914038616748,-0.216455008807559,
-1.69125130044275));
#58957=CARTESIAN_POINT('Ctrl Pts',(-0.522970364169069,-0.530661092879054,
-1.67540193014776));
#58958=CARTESIAN_POINT('Ctrl Pts',(-0.206025011244697,-0.715997829631028,
-1.65955255985279));
#58959=CARTESIAN_POINT('Ctrl Pts',(0.160952856003563,-0.727456785959838,
-1.6437031895578));
#58960=CARTESIAN_POINT('Ctrl Pts',(0.488843837514907,-0.562255191010648,
-1.62785381926283));
#58961=CARTESIAN_POINT('Ctrl Pts',(0.69802065828021,-0.260511723169583,
-1.61200444896784));
#58962=CARTESIAN_POINT('Ctrl Pts',(0.737685397125054,0.104496182529187,
-1.59615507867287));
#58963=CARTESIAN_POINT('Ctrl Pts',(0.59820559922069,0.444127524879664,-1.58030570837788));
#58964=CARTESIAN_POINT('Ctrl Pts',(0.313453486897711,0.675903919833572,
-1.5644563380829));
#58965=CARTESIAN_POINT('Ctrl Pts',(-0.0474198010938648,0.743539211984775,
-1.54860696778792));
#58966=CARTESIAN_POINT('Ctrl Pts',(-0.396777342219896,0.630608387191001,
-1.53275759749294));
#58967=CARTESIAN_POINT('Ctrl Pts',(-0.649778776201089,0.364536334668214,
-1.51690822719796));
#58968=CARTESIAN_POINT('Ctrl Pts',(-0.744983514862478,0.00993780045431491,
-1.50105885690298));
#58969=CARTESIAN_POINT('Ctrl Pts',(-0.65927139224945,-0.347074096780775,
-1.485209486608));
#58970=CARTESIAN_POINT('Ctrl Pts',(-0.413457322903013,-0.619800160884617,
-1.46936011631302));
#58971=CARTESIAN_POINT('Ctrl Pts',(-0.0672364665092823,-0.742009740411855,
-1.45351074601804));
#58972=CARTESIAN_POINT('Ctrl Pts',(0.295312550496548,-0.684024630268491,
-1.43766137572306));
#58973=CARTESIAN_POINT('Ctrl Pts',(0.586145860154621,-0.459926328794428,
-1.42181200542808));
#58974=CARTESIAN_POINT('Ctrl Pts',(0.734635524413049,-0.124136390978171,
-1.4059626351331));
#58975=CARTESIAN_POINT('Ctrl Pts',(0.704721303745212,0.241799671923618,
-1.39011326483812));
#58976=CARTESIAN_POINT('Ctrl Pts',(0.503667770860069,0.5490154587,-1.37426389454314));
#58977=CARTESIAN_POINT('Ctrl Pts',(0.180300132479707,0.72290459918479,-1.35841452424816));
#58978=CARTESIAN_POINT('Ctrl Pts',(-0.186852815783132,0.721238672374574,
-1.34256515395318));
#58979=CARTESIAN_POINT('Ctrl Pts',(-0.508629156003826,0.544422243261198,
-1.3267157836582));
#58980=CARTESIAN_POINT('Ctrl Pts',(-0.706886534232653,0.235394615518856,
-1.31086641336322));
#58981=CARTESIAN_POINT('Ctrl Pts',(-0.733478780952995,-0.130797840908901,
-1.29501704306824));
#58982=CARTESIAN_POINT('Ctrl Pts',(-0.581948054192647,-0.465226460464269,
-1.27916767277326));
#58983=CARTESIAN_POINT('Ctrl Pts',(-0.289093105769863,-0.686676323671537,
-1.26331830247828));
#58984=CARTESIAN_POINT('Ctrl Pts',(0.0739671777623989,-0.741369040295444,
-1.2474689321833));
#58985=CARTESIAN_POINT('Ctrl Pts',(0.419064769005327,-0.61602265922061,
-1.23161956188832));
#58986=CARTESIAN_POINT('Ctrl Pts',(0.662393822869109,-0.341077147753364,
-1.21577019159333));
#58987=CARTESIAN_POINT('Ctrl Pts',(0.744862657720982,0.0166978569750356,
-1.19992082129835));
#58988=CARTESIAN_POINT('Ctrl Pts',(0.646443981068284,0.370417840600733,
-1.18407145100337));
#58989=CARTESIAN_POINT('Ctrl Pts',(0.39103845341634,0.634183037651179,-1.16822208070839));
#58990=CARTESIAN_POINT('Ctrl Pts',(0.040670489390563,0.743938914553779,
-1.15237271041341));
#58991=CARTESIAN_POINT('Ctrl Pts',(-0.319574172763753,0.6730316080223,-1.13652334011843));
#58992=CARTESIAN_POINT('Ctrl Pts',(-0.6022112702843,0.438680730414834,-1.12067396982345));
#58993=CARTESIAN_POINT('Ctrl Pts',(-0.738603288993907,0.097797642006873,
-1.10482459952847));
#58994=CARTESIAN_POINT('Ctrl Pts',(-0.695627863852887,-0.266835290631117,
-1.08897522923349));
#58995=CARTESIAN_POINT('Ctrl Pts',(-0.483721439256766,-0.566668127300346,
-1.07312585893851));
#58996=CARTESIAN_POINT('Ctrl Pts',(-0.15434481193055,-0.728887423629223,
-1.05727648864353));
#58997=CARTESIAN_POINT('Ctrl Pts',(0.212513958787283,-0.714098742902743,
-1.04142711834855));
#58998=CARTESIAN_POINT('Ctrl Pts',(0.527764395047013,-0.525893468884509,
-1.02557774805357));
#58999=CARTESIAN_POINT('Ctrl Pts',(0.714848937781003,-0.209976649768712,
-1.00972837775859));
#59000=CARTESIAN_POINT('Ctrl Pts',(0.728334704799049,0.156932326434056,
-0.993879007463609));
#59001=CARTESIAN_POINT('Ctrl Pts',(0.564946720759936,0.485730789632812,
-0.978029637168628));
#59002=CARTESIAN_POINT('Ctrl Pts',(0.264363234447157,0.696571085796245,
-0.962180266873649));
#59003=CARTESIAN_POINT('Ctrl Pts',(-0.100420016905207,0.738251324075671,
-0.946330896578666));
#59004=CARTESIAN_POINT('Ctrl Pts',(-0.44081658867988,0.600649592057928,
-0.930481526283688));
#59005=CARTESIAN_POINT('Ctrl Pts',(-0.674162263313043,0.317182029786296,
-0.914632155988704));
#59006=CARTESIAN_POINT('Ctrl Pts',(-0.743789790853027,-0.0433121728562648,
-0.898782785693728));
#59007=CARTESIAN_POINT('Ctrl Pts',(-0.632790349172193,-0.393288152998858,
-0.882933415398745));
#59008=CARTESIAN_POINT('Ctrl Pts',(-0.368119797281484,-0.64775536442716,
-0.867084045103766));
#59009=CARTESIAN_POINT('Ctrl Pts',(-0.0140525312776586,-0.744917259606335,
-0.851234674808785));
#59010=CARTESIAN_POINT('Ctrl Pts',(0.343427346953139,-0.661178383387911,
-0.835385304513805));
#59011=CARTESIAN_POINT('Ctrl Pts',(0.617506993572057,-0.416874453743954,
-0.819535934218824));
#59012=CARTESIAN_POINT('Ctrl Pts',(0.741627043953897,-0.0713338977690619,
-0.803686563923845));
#59013=CARTESIAN_POINT('Ctrl Pts',(0.685645341274624,0.291529866880099,
-0.787837193628863));
#59014=CARTESIAN_POINT('Ctrl Pts',(0.463156862786047,0.583596536786253,
-0.771987823333884));
#59015=CARTESIAN_POINT('Ctrl Pts',(0.128192223119029,0.733938656310268,
-0.756138453038902));
#59016=CARTESIAN_POINT('Ctrl Pts',(-0.237903487482845,0.706046123095525,
-0.740289082743923));
#59017=CARTESIAN_POINT('Ctrl Pts',(-0.546225097875833,0.506692549526098,
-0.724439712448941));
#59018=CARTESIAN_POINT('Ctrl Pts',(-0.721897692169123,0.184290312647237,
-0.708590342153963));
#59019=CARTESIAN_POINT('Ctrl Pts',(-0.722259743312219,-0.182866236591916,
-0.692740971858981));
#59020=CARTESIAN_POINT('Ctrl Pts',(-0.547223328344242,-0.505614305781167,
-0.676891601564001));
#59021=CARTESIAN_POINT('Ctrl Pts',(-0.239295480203475,-0.705575559702084,
-0.66104223126902));
#59022=CARTESIAN_POINT('Ctrl Pts',(0.126744509121461,-0.734190048081749,
-0.64519286097404));
#59023=CARTESIAN_POINT('Ctrl Pts',(0.462005000220514,-0.584508834035863,
-0.62934349067906));
#59024=CARTESIAN_POINT('Ctrl Pts',(0.685069056277096,-0.292881521141793,
-0.613494120384079));
#59025=CARTESIAN_POINT('Ctrl Pts',(0.74176628549086,0.0698711314049664,
-0.597644750089099));
#59026=CARTESIAN_POINT('Ctrl Pts',(0.618327947282097,0.415655803405456,
-0.58179537979412));
#59027=CARTESIAN_POINT('Ctrl Pts',(0.344730646856306,0.660499794407802,
-0.565946009499137));
#59028=CARTESIAN_POINT('Ctrl Pts',(-0.0125833873898627,0.744943525145706,
-0.550096639204159));
#59029=CARTESIAN_POINT('Ctrl Pts',(-0.366841586298341,0.64848010598389,
-0.534247268909176));
#59030=CARTESIAN_POINT('Ctrl Pts',(-0.632013480538201,0.394535369406354,
-0.518397898614198));
#59031=CARTESIAN_POINT('Ctrl Pts',(-0.743702924628839,0.044778981603412,
-0.502548528319216));
#59032=CARTESIAN_POINT('Ctrl Pts',(-0.674786494682493,-0.315851838507415,
-0.486699158024237));
#59033=CARTESIAN_POINT('Ctrl Pts',(-0.442000325054718,-0.599779050940051,
-0.470849787729256));
#59034=CARTESIAN_POINT('Ctrl Pts',(-0.101875791694698,-0.738051841242525,
-0.455000417434276));
#59035=CARTESIAN_POINT('Ctrl Pts',(0.262988951485128,-0.697091105014031,
-0.439151047139295));
#59036=CARTESIAN_POINT('Ctrl Pts',(0.563987669851054,-0.4868440259017,-0.423301676844314));
#59037=CARTESIAN_POINT('Ctrl Pts',(0.72802378836902,-0.158368433886228,
-0.407452306549335));
#59038=CARTESIAN_POINT('Ctrl Pts',(0.715261660922253,0.208566425221401,
-0.391602936254353));
#59039=CARTESIAN_POINT('Ctrl Pts',(0.528800529201736,0.524851595774613,
-0.375753565959374));
#59040=CARTESIAN_POINT('Ctrl Pts',(0.213921882219699,0.713678236746709,
-0.359904195664393));
#59041=CARTESIAN_POINT('Ctrl Pts',(-0.152907009165183,0.729190403064095,
-0.344054825369413));
#59042=CARTESIAN_POINT('Ctrl Pts',(-0.482602922472436,0.567621014616206,
-0.328205455074432));
#59043=CARTESIAN_POINT('Ctrl Pts',(-0.695100262217286,0.268206680437639,
-0.312356084779452));
#59044=CARTESIAN_POINT('Ctrl Pts',(-0.738794727018378,-0.096340787809866,
-0.296506714484472));
#59045=CARTESIAN_POINT('Ctrl Pts',(-0.603075261493803,-0.437492203270981,
-0.280657344189491));
#59046=CARTESIAN_POINT('Ctrl Pts',(-0.320900892537525,-0.672400039771382,
-0.264807973894511));
#59047=CARTESIAN_POINT('Ctrl Pts',(0.0392032167528849,-0.744017675942373,
-0.24895860359953));
#59048=CARTESIAN_POINT('Ctrl Pts',(0.389786977696613,-0.634953008741876,
-0.23310923330455));
#59049=CARTESIAN_POINT('Ctrl Pts',(0.645712165630145,-0.371692022642734,
-0.21725986300957));
#59050=CARTESIAN_POINT('Ctrl Pts',(0.744828326399828,-0.0181668458436364,
-0.20141049271459));
#59051=CARTESIAN_POINT('Ctrl Pts',(0.663065107658535,0.339770143995986,
-0.185561122419609));
#59052=CARTESIAN_POINT('Ctrl Pts',(0.420279052557129,0.615194939045757,
-0.169711752124629));
#59053=CARTESIAN_POINT('Ctrl Pts',(0.0754287878286457,0.741221815035238,
-0.153862381829648));
#59054=CARTESIAN_POINT('Ctrl Pts',(-0.287737574375596,0.687244950605065,
-0.138013011534668));
#59055=CARTESIAN_POINT('Ctrl Pts',(-0.581030808350321,0.466373625781902,
-0.122163641239687));
#59056=CARTESIAN_POINT('Ctrl Pts',(-0.733216654906317,0.132243440338671,
-0.106314270944707));
#59057=CARTESIAN_POINT('Ctrl Pts',(-0.70735477396553,-0.233998665021394,
-0.0904649006497263));
#59058=CARTESIAN_POINT('Ctrl Pts',(-0.509691323571145,-0.543420787681075,
-0.0746155303547458));
#59059=CARTESIAN_POINT('Ctrl Pts',(-0.188295790055588,-0.720863304751339,
-0.0587661600597657));
#59060=CARTESIAN_POINT('Ctrl Pts',(0.17891792069232,-0.723270960896346,
-0.0429167897647859));
#59061=CARTESIAN_POINT('Ctrl Pts',(0.394616248151404,-0.607734388455063,
-0.0323505429014652));
#59062=CARTESIAN_POINT('Ctrl Pts',(0.482201081976442,-0.527701441143752,
-0.027067419469805));
#59063=CARTESIAN_POINT('Ctrl Pts',(0.392888236737271,-0.550964357679767,
-3.8089));
#59064=CARTESIAN_POINT('Ctrl Pts',(0.484334114933679,-0.485755039979474,
-3.80361687656834));
#59065=CARTESIAN_POINT('Ctrl Pts',(0.634040615230541,-0.308993274199896,
-3.79305062970502));
#59066=CARTESIAN_POINT('Ctrl Pts',(0.704605176817581,0.0314014527883039,
-3.77720125941004));
#59067=CARTESIAN_POINT('Ctrl Pts',(0.604063223483086,0.364081211703574,
-3.76135188911506));
#59068=CARTESIAN_POINT('Ctrl Pts',(0.356824591291676,0.608388806027088,
-3.74550251882008));
#59069=CARTESIAN_POINT('Ctrl Pts',(0.0229331537905069,0.704928930307171,
-3.7296531485251));
#59070=CARTESIAN_POINT('Ctrl Pts',(-0.316527984197726,0.630290638914377,
-3.71380377823012));
#59071=CARTESIAN_POINT('Ctrl Pts',(-0.57912108147644,0.402582506643355,
-3.69795440793514));
#59072=CARTESIAN_POINT('Ctrl Pts',(-0.701076597404263,0.077111451249784,
-3.68210503764016));
#59073=CARTESIAN_POINT('Ctrl Pts',(-0.652777845604957,-0.267087379168557,
-3.66625566734518));
#59074=CARTESIAN_POINT('Ctrl Pts',(-0.445954115113484,-0.546424125806921,
-3.6504062970502));
#59075=CARTESIAN_POINT('Ctrl Pts',(-0.130831839792564,-0.693063915639031,
-3.63455692675522));
#59076=CARTESIAN_POINT('Ctrl Pts',(0.21606252083174,-0.671395152184437,
-3.61870755646024));
#59077=CARTESIAN_POINT('Ctrl Pts',(0.510486794197391,-0.48668032805703,
-3.60285818616526));
#59078=CARTESIAN_POINT('Ctrl Pts',(0.680940981975007,-0.183776692274722,
-3.58700881587028));
#59079=CARTESIAN_POINT('Ctrl Pts',(0.686030833613329,0.163756498125624,
-3.5711594455753));
#59080=CARTESIAN_POINT('Ctrl Pts',(0.524520293312469,0.471521960898263,
-3.55531007528032));
#59081=CARTESIAN_POINT('Ctrl Pts',(0.235631679485712,0.664779818244593,
-3.53946070498533));
#59082=CARTESIAN_POINT('Ctrl Pts',(-0.110479333395072,0.696598028792635,
-3.52361133469035));
#59083=CARTESIAN_POINT('Ctrl Pts',(-0.429760793823647,0.55924963662321,
-3.50776196439537));
#59084=CARTESIAN_POINT('Ctrl Pts',(-0.644676221530144,0.286089261747328,
-3.49191259410039));
#59085=CARTESIAN_POINT('Ctrl Pts',(-0.703034092962096,-0.0565469748075895,
-3.47606322380541));
#59086=CARTESIAN_POINT('Ctrl Pts',(-0.590662385922995,-0.385450959342922,
-3.46021385351043));
#59087=CARTESIAN_POINT('Ctrl Pts',(-0.334850209657572,-0.620749412673154,
-3.44436448321545));
#59088=CARTESIAN_POINT('Ctrl Pts',(0.00227926788749094,-0.70530085860637,
-3.42851511292047));
#59089=CARTESIAN_POINT('Ctrl Pts',(0.338855232525197,-0.618572249312001,
-3.41266574262549));
#59090=CARTESIAN_POINT('Ctrl Pts',(0.593141288900064,-0.381625349818476,
-3.39681637233051));
#59091=CARTESIAN_POINT('Ctrl Pts',(0.703384882402956,-0.0520019560290773,
-3.38096700203553));
#59092=CARTESIAN_POINT('Ctrl Pts',(0.642813709332344,0.290249946284879,
-3.36511763174055));
#59093=CARTESIAN_POINT('Ctrl Pts',(0.426137285130135,0.562015578472108,
-3.34926826144557));
#59094=CARTESIAN_POINT('Ctrl Pts',(0.105974785652812,0.697297526906368,
-3.33341889115059));
#59095=CARTESIAN_POINT('Ctrl Pts',(-0.239923351207117,0.663243003558396,
-3.31756952085561));
#59096=CARTESIAN_POINT('Ctrl Pts',(-0.527556870419987,0.468122040387345,
-3.30172015056063));
#59097=CARTESIAN_POINT('Ctrl Pts',(-0.687074892798328,0.159319138554876,
-3.28587078026565));
#59098=CARTESIAN_POINT('Ctrl Pts',(-0.679738977357021,-0.188173905962906,
-3.27002140997067));
#59099=CARTESIAN_POINT('Ctrl Pts',(-0.507330627672634,-0.489969519918335,
-3.25417203967569));
#59100=CARTESIAN_POINT('Ctrl Pts',(-0.211718659443945,-0.672777604760268,
-3.23832266938071));
#59101=CARTESIAN_POINT('Ctrl Pts',(0.135308507343731,-0.692203802405131,
-3.22247329908573));
#59102=CARTESIAN_POINT('Ctrl Pts',(0.449476436357704,-0.543530522954218,
-3.20662392879074));
#59103=CARTESIAN_POINT('Ctrl Pts',(0.65449045194897,-0.262862596295751,
-3.19077455849577));
#59104=CARTESIAN_POINT('Ctrl Pts',(0.700563556851036,0.0816406702320175,
-3.17492518820078));
#59105=CARTESIAN_POINT('Ctrl Pts',(0.576507045056651,0.406317761393417,
-3.1590758179058));
#59106=CARTESIAN_POINT('Ctrl Pts',(0.312447643247322,0.632321885160478,
-3.14322644761082));
#59107=CARTESIAN_POINT('Ctrl Pts',(-0.0274886683206437,0.704768663702968,
-3.12737707731584));
#59108=CARTESIAN_POINT('Ctrl Pts',(-0.360749444800962,0.606064628814044,
-3.11152770702087));
#59109=CARTESIAN_POINT('Ctrl Pts',(-0.606403373669456,0.360179739333031,
-3.09567833672588));
#59110=CARTESIAN_POINT('Ctrl Pts',(-0.704794184842326,0.0268263533889801,
-3.0798289664309));
#59111=CARTESIAN_POINT('Ctrl Pts',(-0.632027984856805,-0.313041726582184,
-3.06397959613592));
#59112=CARTESIAN_POINT('Ctrl Pts',(-0.405775812394436,-0.576888625558993,
-3.04813022584094));
#59113=CARTESIAN_POINT('Ctrl Pts',(-0.0809822831169064,-0.700639968917618,
-3.03228085554596));
#59114=CARTESIAN_POINT('Ctrl Pts',(0.263477534324128,-0.654243139154081,
-3.01643148525098));
#59115=CARTESIAN_POINT('Ctrl Pts',(0.543952676164601,-0.448965457821732,
-3.000582114956));
#59116=CARTESIAN_POINT('Ctrl Pts',(0.692330652242036,-0.134657952568069,
-2.98473274466102));
#59117=CARTESIAN_POINT('Ctrl Pts',(0.672578346146962,0.212350805314992,
-2.96888337436604));
#59118=CARTESIAN_POINT('Ctrl Pts',(0.489492542171056,0.507790850038306,
-2.95303400407106));
#59119=CARTESIAN_POINT('Ctrl Pts',(0.1875350416004,0.679915512689367,-2.93718463377608));
#59120=CARTESIAN_POINT('Ctrl Pts',(-0.159964743367749,0.686924870057126,
-2.9213352634811));
#59121=CARTESIAN_POINT('Ctrl Pts',(-0.468617602588818,0.527116722147587,
-2.90548589318612));
#59122=CARTESIAN_POINT('Ctrl Pts',(-0.663468177454696,0.239299966002197,
-2.88963652289114));
#59123=CARTESIAN_POINT('Ctrl Pts',(-0.697197629737455,-0.106630020689219,
-2.87378715259615));
#59124=CARTESIAN_POINT('Ctrl Pts',(-0.56161486994617,-0.426665248267367,
-2.85793778230118));
#59125=CARTESIAN_POINT('Ctrl Pts',(-0.289645737183324,-0.643086186413016,
-2.84208841200619));
#59126=CARTESIAN_POINT('Ctrl Pts',(0.0526629354583269,-0.703335703240367,
-2.82623904171122));
#59127=CARTESIAN_POINT('Ctrl Pts',(0.382182582841647,-0.592782396496553,
-2.81038967141623));
#59128=CARTESIAN_POINT('Ctrl Pts',(0.618890413665208,-0.33827378275151,
-2.79454030112126));
#59129=CARTESIAN_POINT('Ctrl Pts',(0.705302689111543,-0.0016164639601243,
-2.77869093082627));
#59130=CARTESIAN_POINT('Ctrl Pts',(0.620434464765853,0.335433407928336,
-2.7628415605313));
#59131=CARTESIAN_POINT('Ctrl Pts',(0.384895717176935,0.591024350701866,
-2.74699219023631));
#59132=CARTESIAN_POINT('Ctrl Pts',(0.0558862770419258,0.703086922266445,
-2.73114281994134));
#59133=CARTESIAN_POINT('Ctrl Pts',(-0.286694966534403,0.644407085922823,
-2.71529344964635));
#59134=CARTESIAN_POINT('Ctrl Pts',(-0.559653255436154,0.429235052044242,
-2.69944407935137));
#59135=CARTESIAN_POINT('Ctrl Pts',(-0.696701543169347,0.109824660114017,
-2.68359470905639));
#59136=CARTESIAN_POINT('Ctrl Pts',(-0.664558091863175,-0.236256298885097,
-2.66774533876141));
#59137=CARTESIAN_POINT('Ctrl Pts',(-0.471028835749505,-0.52496317215227,
-2.65189596846643));
#59138=CARTESIAN_POINT('Ctrl Pts',(-0.163111735027927,-0.686184419904654,
-2.63604659817145));
#59139=CARTESIAN_POINT('Ctrl Pts',(0.184416528289274,-0.680767978328477,
-2.62019722787647));
#59140=CARTESIAN_POINT('Ctrl Pts',(0.487159828181642,-0.510029212917986,
-2.60434785758149));
#59141=CARTESIAN_POINT('Ctrl Pts',(0.671597923602639,-0.21543148617677,
-2.58849848728651));
#59142=CARTESIAN_POINT('Ctrl Pts',(0.692940613618548,0.131483087207663,
-2.57264911699153));
#59143=CARTESIAN_POINT('Ctrl Pts',(0.546004894294652,0.446467413850098,
-2.55679974669655));
#59144=CARTESIAN_POINT('Ctrl Pts',(0.266473634605688,0.653028558551418,
-2.54095037640157));
#59145=CARTESIAN_POINT('Ctrl Pts',(-0.0777698940442144,0.701003808694404,
-2.52510100610659));
#59146=CARTESIAN_POINT('Ctrl Pts',(-0.403127252931393,0.578742528390386,
-2.50925163581161));
#59147=CARTESIAN_POINT('Ctrl Pts',(-0.630586449188775,0.315935478101465,
-2.49340226551663));
#59148=CARTESIAN_POINT('Ctrl Pts',(-0.704909745290741,-0.0235954914729733,
-2.47755289522165));
#59149=CARTESIAN_POINT('Ctrl Pts',(-0.608047966749425,-0.357396371491931,
-2.46170352492667));
#59150=CARTESIAN_POINT('Ctrl Pts',(-0.363523686348719,-0.604404687016196,
-2.44585415463169));
#59151=CARTESIAN_POINT('Ctrl Pts',(-0.0307188426589624,-0.704635259499128,
-2.43000478433671));
#59152=CARTESIAN_POINT('Ctrl Pts',(0.309545973614037,-0.633747415334411,
-2.41415541404173));
#59153=CARTESIAN_POINT('Ctrl Pts',(0.574638541308189,-0.408956040506685,
-2.39830604374675));
#59154=CARTESIAN_POINT('Ctrl Pts',(0.700181979140083,-0.0848510006492837,
-2.38245667345177));
#59155=CARTESIAN_POINT('Ctrl Pts',(0.655688465200883,0.259859833037388,
-2.36660730315679));
#59156=CARTESIAN_POINT('Ctrl Pts',(0.451963106890093,0.54146453829772,-2.35075793286181));
#59157=CARTESIAN_POINT('Ctrl Pts',(0.138479955179697,0.691576314109395,
-2.33490856256682));
#59158=CARTESIAN_POINT('Ctrl Pts',(-0.20863261025693,0.673740996348811,
-2.31905919227184));
#59159=CARTESIAN_POINT('Ctrl Pts',(-0.505079414298638,0.492289834828481,
-2.30320982197686));
#59160=CARTESIAN_POINT('Ctrl Pts',(-0.678869299755915,0.191287663148,-2.28736045168189));
#59161=CARTESIAN_POINT('Ctrl Pts',(-0.687797949390983,-0.156168105057554,
-2.2715110813869));
#59162=CARTESIAN_POINT('Ctrl Pts',(-0.529697069227978,-0.465698948973474,
-2.25566171109192));
#59163=CARTESIAN_POINT('Ctrl Pts',(-0.24296095180248,-0.662136294219658,
-2.23981234079694));
#59164=CARTESIAN_POINT('Ctrl Pts',(0.102777454848793,-0.69777596046189,
-2.22396297050196));
#59165=CARTESIAN_POINT('Ctrl Pts',(0.423556685665886,-0.563962968865366,
-2.20811360020698));
#59166=CARTESIAN_POINT('Ctrl Pts',(0.641476531525165,-0.293193375992965,
-2.192264229912));
#59167=CARTESIAN_POINT('Ctrl Pts',(0.70361585560182,0.048777289484231,-2.17641485961702));
#59168=CARTESIAN_POINT('Ctrl Pts',(0.59488432200333,0.378902546386728,-2.16056548932204));
#59169=CARTESIAN_POINT('Ctrl Pts',(0.341687035524299,0.617012533080427,
-2.14471611902706));
#59170=CARTESIAN_POINT('Ctrl Pts',(0.00551214649170594,0.70528300168426,
-2.12886674873208));
#59171=CARTESIAN_POINT('Ctrl Pts',(-0.332001349667448,0.622277751524753,
-2.1130173784371));
#59172=CARTESIAN_POINT('Ctrl Pts',(-0.588889381071465,0.388154341834502,
-2.09716800814212));
#59173=CARTESIAN_POINT('Ctrl Pts',(-0.702767511805465,0.0597688930336289,
-2.08131863784714));
#59174=CARTESIAN_POINT('Ctrl Pts',(-0.645980802439012,-0.283131240070673,
-2.06546926755216));
#59175=CARTESIAN_POINT('Ctrl Pts',(-0.432319723520416,-0.557273858061672,
-2.04961989725718));
#59176=CARTESIAN_POINT('Ctrl Pts',(-0.113671183958779,-0.69608430391808,
-2.0337705269622));
#59177=CARTESIAN_POINT('Ctrl Pts',(0.232582038671535,-0.665852905311,-2.01792115666722));
#59178=CARTESIAN_POINT('Ctrl Pts',(0.522353457898419,-0.473921260596391,
-2.00207178637224));
#59179=CARTESIAN_POINT('Ctrl Pts',(0.685273012361204,-0.166899355160858,
-1.98622241607726));
#59180=CARTESIAN_POINT('Ctrl Pts',(0.681776209899179,0.180653524292269,
-1.97037304578227));
#59181=CARTESIAN_POINT('Ctrl Pts',(0.512712237794087,0.484335273792739,
-1.9545236754873));
#59182=CARTESIAN_POINT('Ctrl Pts',(0.219137740357689,0.670397752811446,
-1.93867430519231));
#59183=CARTESIAN_POINT('Ctrl Pts',(-0.12765365568297,0.693656284058958,
-1.92282493489733));
#59184=CARTESIAN_POINT('Ctrl Pts',(-0.443444770166212,0.548462607691666,
-1.90697556460235));
#59185=CARTESIAN_POINT('Ctrl Pts',(-0.651546742048982,0.270076543130026,
-1.89112619430737));
#59186=CARTESIAN_POINT('Ctrl Pts',(-0.701422673766515,-0.0738967451917915,
-1.87527682401239));
#59187=CARTESIAN_POINT('Ctrl Pts',(-0.580960354995419,-0.399924445548537,
-1.85942745371742));
#59188=CARTESIAN_POINT('Ctrl Pts',(-0.319413674149484,-0.628831774793575,
-1.84357808342243));
#59189=CARTESIAN_POINT('Ctrl Pts',(0.0197015947556392,-0.705029320941897,
-1.82772871312745));
#59190=CARTESIAN_POINT('Ctrl Pts',(0.354032394455494,-0.610012753882915,
-1.81187934283247));
#59191=CARTESIAN_POINT('Ctrl Pts',(0.602387560713073,-0.366856542700088,
-1.79602997253749));
#59192=CARTESIAN_POINT('Ctrl Pts',(0.704454836593539,-0.0346103947345185,
-1.78018060224251));
#59193=CARTESIAN_POINT('Ctrl Pts',(0.635447510951297,0.306040776775757,
-1.76433123194753));
#59194=CARTESIAN_POINT('Ctrl Pts',(0.412123791868901,0.572370925536324,
-1.74848186165255));
#59195=CARTESIAN_POINT('Ctrl Pts',(0.0887171294811145,0.699702627664309,
-1.73263249135757));
#59196=CARTESIAN_POINT('Ctrl Pts',(-0.256234203744069,0.657113786992292,
-1.71678312106259));
#59197=CARTESIAN_POINT('Ctrl Pts',(-0.53895988100815,0.454946967115278,
-1.70093375076761));
#59198=CARTESIAN_POINT('Ctrl Pts',(-0.690800876826863,0.142297732936779,
-1.68508438047263));
#59199=CARTESIAN_POINT('Ctrl Pts',(-0.674883091534556,-0.204908050072388,
-1.66923501017765));
#59200=CARTESIAN_POINT('Ctrl Pts',(-0.495072108323442,-0.502352569202039,
-1.65338563988267));
#59201=CARTESIAN_POINT('Ctrl Pts',(-0.195034448742293,-0.677802375348079,
-1.63753626958769));
#59202=CARTESIAN_POINT('Ctrl Pts',(0.152366702248935,-0.688650044848245,
-1.62168689929271));
#59203=CARTESIAN_POINT('Ctrl Pts',(0.462766087451164,-0.532261255896812,
-1.60583752899773));
#59204=CARTESIAN_POINT('Ctrl Pts',(0.660784210013829,-0.246614525160438,
-1.58998815870274));
#59205=CARTESIAN_POINT('Ctrl Pts',(0.698333002892782,0.0989217533935704,
-1.57413878840777));
#59206=CARTESIAN_POINT('Ctrl Pts',(0.566293861962189,0.420435200866502,
-1.55828941811278));
#59207=CARTESIAN_POINT('Ctrl Pts',(0.296732069830279,0.639847305970687,
-1.54244004781781));
#59208=CARTESIAN_POINT('Ctrl Pts',(-0.0448901553745235,0.703874541501651,
-1.52659067752282));
#59209=CARTESIAN_POINT('Ctrl Pts',(-0.37561095007723,0.596968098314967,
-1.51074130722784));
#59210=CARTESIAN_POINT('Ctrl Pts',(-0.615115828195774,0.345089863842356,
-1.49489193693286));
#59211=CARTESIAN_POINT('Ctrl Pts',(-0.705241796932766,0.00940766085441594,
-1.47904256663788));
#59212=CARTESIAN_POINT('Ctrl Pts',(-0.624102053348382,-0.328559162450296,
-1.4631931963429));
#59213=CARTESIAN_POINT('Ctrl Pts',(-0.391401124376496,-0.58673644514426,
-1.44734382604792));
#59214=CARTESIAN_POINT('Ctrl Pts',(-0.0636496855493053,-0.702426660764798,
-1.43149445575294));
#59215=CARTESIAN_POINT('Ctrl Pts',(0.279558875618117,-0.647534810868762,
-1.41564508545796));
#59216=CARTESIAN_POINT('Ctrl Pts',(0.554877458941432,-0.435391205449084,
-1.39979571516298));
#59217=CARTESIAN_POINT('Ctrl Pts',(0.695445827983648,-0.117514239834355,
-1.383946344868));
#59218=CARTESIAN_POINT('Ctrl Pts',(0.667127404398765,0.228900682663626,
-1.36809697457302));
#59219=CARTESIAN_POINT('Ctrl Pts',(0.476799226683618,0.51972780727763,-1.35224760427804));
#59220=CARTESIAN_POINT('Ctrl Pts',(0.170681883398015,0.684340697973908,
-1.33639823398306));
#59221=CARTESIAN_POINT('Ctrl Pts',(-0.176885008776566,0.682763641309219,
-1.32054886368808));
#59222=CARTESIAN_POINT('Ctrl Pts',(-0.481495942925332,0.515379620445116,
-1.3046994933931));
#59223=CARTESIAN_POINT('Ctrl Pts',(-0.669177129002431,0.222837308913415,
-1.28885012309812));
#59224=CARTESIAN_POINT('Ctrl Pts',(-0.69435079189213,-0.123820329600919,
-1.27300075280314));
#59225=CARTESIAN_POINT('Ctrl Pts',(-0.550903588163435,-0.440408597523208,
-1.25715138250816));
#59226=CARTESIAN_POINT('Ctrl Pts',(-0.273671211948421,-0.650045047650077,
-1.24130201221318));
#59227=CARTESIAN_POINT('Ctrl Pts',(0.0700213418398019,-0.70182013928831,
-1.2254526419182));
#59228=CARTESIAN_POINT('Ctrl Pts',(0.396709436958603,-0.583160457208559,
-1.20960327162322));
#59229=CARTESIAN_POINT('Ctrl Pts',(0.627057915507849,-0.322882125275867,
-1.19375390132824));
#59230=CARTESIAN_POINT('Ctrl Pts',(0.705127387008331,0.0158070969666729,
-1.17790453103325));
#59231=CARTESIAN_POINT('Ctrl Pts',(0.611958930271261,0.35065761632248,-1.16205516073828));
#59232=CARTESIAN_POINT('Ctrl Pts',(0.37017820670576,0.600352056300146,-1.14620579044329));
#59233=CARTESIAN_POINT('Ctrl Pts',(0.0385008908891459,0.704252921630042,
-1.13035642014832));
#59234=CARTESIAN_POINT('Ctrl Pts',(-0.302526243006624,0.637128219839621,
-1.11450704985333));
#59235=CARTESIAN_POINT('Ctrl Pts',(-0.570085847425583,0.41527896983686,
-1.09865767955835));
#59236=CARTESIAN_POINT('Ctrl Pts',(-0.699201929114728,0.0925805516615262,
-1.08280830926337));
#59237=CARTESIAN_POINT('Ctrl Pts',(-0.658519061043479,-0.2526007570577,
-1.06695893896839));
#59238=CARTESIAN_POINT('Ctrl Pts',(-0.45791694746335,-0.536438780709928,
-1.05110956867341));
#59239=CARTESIAN_POINT('Ctrl Pts',(-0.146111169363581,-0.69000436405208,
-1.03526019837843));
#59240=CARTESIAN_POINT('Ctrl Pts',(0.201177238393133,-0.676004596860274,
-1.01941082808345));
#59241=CARTESIAN_POINT('Ctrl Pts',(0.49961039794122,-0.497839277772177,
-1.00356145778847));
#59242=CARTESIAN_POINT('Ctrl Pts',(0.676714772016422,-0.198775284073422,
-0.987712087493491));
#59243=CARTESIAN_POINT('Ctrl Pts',(0.689481130432523,0.148560650918064,
-0.971862717198511));
#59244=CARTESIAN_POINT('Ctrl Pts',(0.53480920392387,0.459819107499921,-0.956013346903531));
#59245=CARTESIAN_POINT('Ctrl Pts',(0.250260574610009,0.659411966087648,
-0.94016397660855));
#59246=CARTESIAN_POINT('Ctrl Pts',(-0.0950630339562937,0.698868740035448,
-0.92431460631357));
#59247=CARTESIAN_POINT('Ctrl Pts',(-0.417300889101903,0.568607478123943,
-0.908465236018589));
#59248=CARTESIAN_POINT('Ctrl Pts',(-0.638198559455265,0.30026171073404,
-0.892615865723609));
#59249=CARTESIAN_POINT('Ctrl Pts',(-0.70411175304767,-0.0410016517209196,
-0.876766495428628));
#59250=CARTESIAN_POINT('Ctrl Pts',(-0.599033661857993,-0.372307894335739,
-0.860917125133648));
#59251=CARTESIAN_POINT('Ctrl Pts',(-0.348482163889545,-0.613200356877398,
-0.845067754838668));
#59252=CARTESIAN_POINT('Ctrl Pts',(-0.0133028882008698,-0.705179076114163,
-0.829218384543688));
#59253=CARTESIAN_POINT('Ctrl Pts',(0.325106951293811,-0.625907314579525,
-0.813369014248707));
#59254=CARTESIAN_POINT('Ctrl Pts',(0.584565608603702,-0.394635965747537,
-0.797519643953726));
#59255=CARTESIAN_POINT('Ctrl Pts',(0.702064379543393,-0.067528536190703,
-0.781670273658747));
#59256=CARTESIAN_POINT('Ctrl Pts',(0.64906906380117,0.275977982165213,-0.765820903363766));
#59257=CARTESIAN_POINT('Ctrl Pts',(0.438449404123081,0.552464131186653,
-0.749971533068786));
#59258=CARTESIAN_POINT('Ctrl Pts',(0.121353710493789,0.694786134845175,
-0.734122162773805));
#59259=CARTESIAN_POINT('Ctrl Pts',(-0.225212343175068,0.66838155024305,
-0.718272792478825));
#59260=CARTESIAN_POINT('Ctrl Pts',(-0.517086300395306,0.479662646207939,
-0.702423422183845));
#59261=CARTESIAN_POINT('Ctrl Pts',(-0.683387505186542,0.174459204339074,
-0.686574051888864));
#59262=CARTESIAN_POINT('Ctrl Pts',(-0.683730242433263,-0.173111096714972,
-0.670724681593884));
#59263=CARTESIAN_POINT('Ctrl Pts',(-0.518031279492488,-0.478641922203943,
-0.654875311298903));
#59264=CARTESIAN_POINT('Ctrl Pts',(-0.226530078974616,-0.667936089415343,
-0.639025941003923));
#59265=CARTESIAN_POINT('Ctrl Pts',(0.119983225911628,-0.695024115929475,
-0.623176570708943));
#59266=CARTESIAN_POINT('Ctrl Pts',(0.437358988551026,-0.553327761238609,
-0.607327200413961));
#59267=CARTESIAN_POINT('Ctrl Pts',(0.648523521169567,-0.277257531391908,
-0.591477830118983));
#59268=CARTESIAN_POINT('Ctrl Pts',(0.702196193133595,0.0661438022220719,
-0.575628459824));
#59269=CARTESIAN_POINT('Ctrl Pts',(0.585342767907381,0.393482325247575,
-0.559779089529022));
#59270=CARTESIAN_POINT('Ctrl Pts',(0.326340725662382,0.625264925449887,
-0.54392971923404));
#59271=CARTESIAN_POINT('Ctrl Pts',(-0.011912116922439,0.705203940498158,
-0.528080348939061));
#59272=CARTESIAN_POINT('Ctrl Pts',(-0.347272140053286,0.613886436539002,
-0.51223097864408));
#59273=CARTESIAN_POINT('Ctrl Pts',(-0.59829823587811,0.373488577025802,
-0.496381608349099));
#59274=CARTESIAN_POINT('Ctrl Pts',(-0.704029520768948,0.0423902124285739,
-0.480532238054118));
#59275=CARTESIAN_POINT('Ctrl Pts',(-0.638789490722744,-0.299002479530853,
-0.464682867759139));
#59276=CARTESIAN_POINT('Ctrl Pts',(-0.41842147815042,-0.567783376690792,
-0.448833497464158));
#59277=CARTESIAN_POINT('Ctrl Pts',(-0.0964411493212378,-0.698679898767291,
-0.432984127169178));
#59278=CARTESIAN_POINT('Ctrl Pts',(0.248959603828383,-0.659904244480755,
-0.417134756874197));
#59279=CARTESIAN_POINT('Ctrl Pts',(0.533901314322515,-0.4608729573248,-0.401285386579217));
#59280=CARTESIAN_POINT('Ctrl Pts',(0.689186800078316,-0.149920148114908,
-0.385436016284236));
#59281=CARTESIAN_POINT('Ctrl Pts',(0.677105478124627,0.197440289037993,
-0.369586645989256));
#59282=CARTESIAN_POINT('Ctrl Pts',(0.50059125872345,0.496852984183748,-0.353737275694276));
#59283=CARTESIAN_POINT('Ctrl Pts',(0.202510055068408,0.675606522928187,
-0.337887905399296));
#59284=CARTESIAN_POINT('Ctrl Pts',(-0.144750067291325,0.690291180816235,
-0.322038535104314));
#59285=CARTESIAN_POINT('Ctrl Pts',(-0.456858098816181,0.537340835519866,
-0.306189164809335));
#59286=CARTESIAN_POINT('Ctrl Pts',(-0.65801960472246,0.253898989021423,
-0.290339794514354));
#59287=CARTESIAN_POINT('Ctrl Pts',(-0.699383154730711,-0.091201414470888,
-0.274490424219375));
#59288=CARTESIAN_POINT('Ctrl Pts',(-0.570903748360253,-0.414153845586582,
-0.258641053924393));
#59289=CARTESIAN_POINT('Ctrl Pts',(-0.303782187894811,-0.636530343082252,
-0.242791683629414));
#59290=CARTESIAN_POINT('Ctrl Pts',(0.0371118910375575,-0.704327481431854,
-0.226942313334432));
#59291=CARTESIAN_POINT('Ctrl Pts',(0.36899349191975,-0.601080952691479,
-0.211092943039453));
#59292=CARTESIAN_POINT('Ctrl Pts',(0.611266154089886,-0.351863826144559,
-0.195243572744473));
#59293=CARTESIAN_POINT('Ctrl Pts',(0.705094887117879,-0.0171977214955263,
-0.179394202449492));
#59294=CARTESIAN_POINT('Ctrl Pts',(0.627693390094468,0.321644844638033,
-0.163544832154511));
#59295=CARTESIAN_POINT('Ctrl Pts',(0.39785894362146,0.58237689240233,-0.147695461859531));
#59296=CARTESIAN_POINT('Ctrl Pts',(0.071404981194182,0.701680767872716,
-0.13184609156455));
#59297=CARTESIAN_POINT('Ctrl Pts',(-0.272387992417769,0.650583340742987,
-0.11599672126957));
#59298=CARTESIAN_POINT('Ctrl Pts',(-0.550035273505243,0.441494566425662,
-0.100147350974589));
#59299=CARTESIAN_POINT('Ctrl Pts',(-0.694102649160791,0.125188812418524,
-0.084297980679609));
#59300=CARTESIAN_POINT('Ctrl Pts',(-0.669620390127032,-0.221515826467681,
-0.0684486103846286));
#59301=CARTESIAN_POINT('Ctrl Pts',(-0.482501448347761,-0.514431588282284,
-0.0525992400896481));
#59302=CARTESIAN_POINT('Ctrl Pts',(-0.178251006477893,-0.682408297960222,
-0.036749869794668));
#59303=CARTESIAN_POINT('Ctrl Pts',(0.169373406760312,-0.684687515838503,
-0.0209004994996882));
#59304=CARTESIAN_POINT('Ctrl Pts',(0.37356514123207,-0.575314330614417,
-0.0103342526363675));
#59305=CARTESIAN_POINT('Ctrl Pts',(0.456477694810158,-0.499550802362287,
-0.00505112920470729));
#59306=CARTESIAN_POINT('Ctrl Pts',(0.533647856309012,-0.584002718706682,
-0.0711000000000004));
#59307=CARTESIAN_POINT('Ctrl Pts',(0.436718461990072,-0.672574504136354,
-0.0763831234316606));
#59308=CARTESIAN_POINT('Ctrl Pts',(0.317362705273201,-0.736506177574195,
-0.0816662468633211));
#59309=CARTESIAN_POINT('Ctrl Pts',(0.189952775953544,-0.768027925513371,
-0.0869493702949814));
#59310=CARTESIAN_POINT('Ctrl Pts',(0.0625428466338946,-0.799549673452546,
-0.0922324937266413));
#59311=CARTESIAN_POINT('Ctrl Pts',(-0.0729212552885391,-0.79866149589306,
-0.0975156171583011));
#59312=CARTESIAN_POINT('Ctrl Pts',(-0.199934259050909,-0.7654883851375,
-0.102798740589961));
#59313=CARTESIAN_POINT('Ctrl Pts',(-0.326947262813287,-0.732315274381938,
-0.108081864021621));
#59314=CARTESIAN_POINT('Ctrl Pts',(-0.4455091684156,-0.666857230430297,
-0.113364987453281));
#59315=CARTESIAN_POINT('Ctrl Pts',(-0.541248865820859,-0.57705573439617,
-0.118648110884941));
#59316=CARTESIAN_POINT('Ctrl Pts',(-0.636988563226119,-0.487254238362043,
-0.123931234316602));
#59317=CARTESIAN_POINT('Ctrl Pts',(-0.709906052434325,-0.373109290245429,
-0.129214357748262));
#59318=CARTESIAN_POINT('Ctrl Pts',(-0.751134984497568,-0.248483976469156,
-0.134497481179922));
#59319=CARTESIAN_POINT('Ctrl Pts',(-0.777588539083348,-0.168521135430888,
-0.137887270512046));
#59320=CARTESIAN_POINT('Ctrl Pts',(-0.79099642429751,-0.0842436963923346,
-0.14127705984417));
#59321=CARTESIAN_POINT('Ctrl Pts',(-0.791054317571617,1.54395522024842E-5,
-0.144666849176294));
#59322=CARTESIAN_POINT('Origin',(0.,0.,-0.599));
#59323=CARTESIAN_POINT('',(0.23094010767585,-0.4,-0.599));
#59324=CARTESIAN_POINT('',(-0.230940107675851,-0.4,-0.599));
#59325=CARTESIAN_POINT('',(0.115470053837925,-0.4,-0.599));
#59326=CARTESIAN_POINT('Origin',(0.,0.,-0.599));
#59327=CARTESIAN_POINT('Origin',(0.,0.,-0.599));
#59328=CARTESIAN_POINT('',(-0.461880215351701,1.11022302462516E-16,-0.599));
#59329=CARTESIAN_POINT('',(-0.288675134594813,-0.3,-0.599));
#59330=CARTESIAN_POINT('Origin',(0.,0.,-0.599));
#59331=CARTESIAN_POINT('Origin',(0.,0.,-0.599));
#59332=CARTESIAN_POINT('',(-0.23094010767585,0.4,-0.599));
#59333=CARTESIAN_POINT('',(-0.404145188432738,0.1,-0.599));
#59334=CARTESIAN_POINT('Origin',(0.,0.,-0.599));
#59335=CARTESIAN_POINT('Origin',(0.,0.,-0.599));
#59336=CARTESIAN_POINT('',(0.23094010767585,0.4,-0.599));
#59337=CARTESIAN_POINT('',(-0.115470053837925,0.4,-0.599));
#59338=CARTESIAN_POINT('Origin',(0.,0.,-0.599));
#59339=CARTESIAN_POINT('Origin',(0.,0.,-0.599));
#59340=CARTESIAN_POINT('',(0.461880215351701,0.,-0.599));
#59341=CARTESIAN_POINT('',(0.288675134594813,0.3,-0.599));
#59342=CARTESIAN_POINT('Origin',(0.,0.,-0.599));
#59343=CARTESIAN_POINT('Origin',(0.,0.,-0.599));
#59344=CARTESIAN_POINT('',(0.404145188432738,-0.1,-0.599));
#59345=CARTESIAN_POINT('Origin',(0.,0.,-0.599));
#59346=CARTESIAN_POINT('Origin',(0.,0.,-0.73806406460551));
#59347=CARTESIAN_POINT('',(0.,0.,-0.87712812921102));
#59348=CARTESIAN_POINT('',(-0.460219541126976,-5.63606387946214E-17,-0.6));
#59349=CARTESIAN_POINT('',(-0.23094010767585,-2.82820063659975E-17,-0.73806406460551));
#59350=CARTESIAN_POINT('',(-0.460210453731243,-0.00289211196316049,-0.6));
#59351=CARTESIAN_POINT('Origin',(0.,0.,-0.6));
#59352=CARTESIAN_POINT('Ctrl Pts',(-0.4618802153517,-6.93889390390722E-16,
-0.599));
#59353=CARTESIAN_POINT('Ctrl Pts',(-0.461043830945924,-0.00144866028546382,
-0.599503641468823));
#59354=CARTESIAN_POINT('Ctrl Pts',(-0.460210453731243,-0.00289211196316079,
-0.6));
#59355=CARTESIAN_POINT('',(-0.232609869296308,-0.397107888036839,-0.6));
#59356=CARTESIAN_POINT('Ctrl Pts',(-0.232609869296308,-0.397107888036839,
-0.6));
#59357=CARTESIAN_POINT('Ctrl Pts',(-0.231776492081632,-0.398551339714529,
-0.599503641468825));
#59358=CARTESIAN_POINT('Ctrl Pts',(-0.230940107675851,-0.399999999999999,
-0.599));
#59359=CARTESIAN_POINT('',(-0.227600584434936,-0.4,-0.6));
#59360=CARTESIAN_POINT('Origin',(0.,0.,-0.6));
#59361=CARTESIAN_POINT('Ctrl Pts',(-0.23094010767585,-0.4,-0.599));
#59362=CARTESIAN_POINT('Ctrl Pts',(-0.229267338864258,-0.4,-0.599503641468835));
#59363=CARTESIAN_POINT('Ctrl Pts',(-0.227600584434936,-0.4,-0.6));
#59364=CARTESIAN_POINT('',(0.227600584434936,-0.4,-0.6));
#59365=CARTESIAN_POINT('Ctrl Pts',(0.227600584434936,-0.4,-0.6));
#59366=CARTESIAN_POINT('Ctrl Pts',(0.229267338864223,-0.4,-0.599503641468845));
#59367=CARTESIAN_POINT('Ctrl Pts',(0.23094010767585,-0.4,-0.599));
#59368=CARTESIAN_POINT('',(0.232609869296308,-0.397107888036839,-0.6));
#59369=CARTESIAN_POINT('Origin',(0.,0.,-0.6));
#59370=CARTESIAN_POINT('Ctrl Pts',(0.230940107675851,-0.399999999999999,
-0.599));
#59371=CARTESIAN_POINT('Ctrl Pts',(0.231776492081654,-0.39855133971449,
-0.599503641468839));
#59372=CARTESIAN_POINT('Ctrl Pts',(0.232609869296308,-0.397107888036839,
-0.6));
#59373=CARTESIAN_POINT('',(0.460210453731243,-0.0028921119631606,-0.6));
#59374=CARTESIAN_POINT('Ctrl Pts',(0.460210453731243,-0.00289211196316057,
-0.6));
#59375=CARTESIAN_POINT('Ctrl Pts',(0.461043830945901,-0.00144866028550258,
-0.599503641468836));
#59376=CARTESIAN_POINT('Ctrl Pts',(0.4618802153517,-7.21644966006351E-16,
-0.599));
#59377=CARTESIAN_POINT('',(0.460210453731243,0.0028921119631606,-0.6));
#59378=CARTESIAN_POINT('Origin',(0.,0.,-0.6));
#59379=CARTESIAN_POINT('Ctrl Pts',(0.4618802153517,9.15933995315753E-16,
-0.599));
#59380=CARTESIAN_POINT('Ctrl Pts',(0.461043830945894,0.00144866028551485,
-0.59950364146884));
#59381=CARTESIAN_POINT('Ctrl Pts',(0.460210453731243,0.0028921119631606,
-0.6));
#59382=CARTESIAN_POINT('',(0.232609869296308,0.397107888036839,-0.6));
#59383=CARTESIAN_POINT('Ctrl Pts',(0.232609869296308,0.397107888036839,
-0.6));
#59384=CARTESIAN_POINT('Ctrl Pts',(0.231776492081656,0.398551339714487,
-0.59950364146884));
#59385=CARTESIAN_POINT('Ctrl Pts',(0.230940107675851,0.399999999999999,
-0.599));
#59386=CARTESIAN_POINT('',(0.227600584434936,0.4,-0.6));
#59387=CARTESIAN_POINT('Origin',(0.,0.,-0.6));
#59388=CARTESIAN_POINT('Ctrl Pts',(0.23094010767585,0.4,-0.599));
#59389=CARTESIAN_POINT('Ctrl Pts',(0.229267338864267,0.4,-0.599503641468832));
#59390=CARTESIAN_POINT('Ctrl Pts',(0.227600584434936,0.4,-0.6));
#59391=CARTESIAN_POINT('',(-0.227600584434936,0.4,-0.6));
#59392=CARTESIAN_POINT('Ctrl Pts',(-0.227600584434935,0.4,-0.6));
#59393=CARTESIAN_POINT('Ctrl Pts',(-0.22926733886426,0.4,-0.599503641468834));
#59394=CARTESIAN_POINT('Ctrl Pts',(-0.230940107675849,0.4,-0.599));
#59395=CARTESIAN_POINT('',(-0.232609869296308,0.397107888036839,-0.6));
#59396=CARTESIAN_POINT('Origin',(0.,0.,-0.6));
#59397=CARTESIAN_POINT('Ctrl Pts',(-0.230940107675851,0.399999999999999,
-0.599));
#59398=CARTESIAN_POINT('Ctrl Pts',(-0.231776492081655,0.398551339714488,
-0.599503641468839));
#59399=CARTESIAN_POINT('Ctrl Pts',(-0.232609869296308,0.397107888036839,
-0.6));
#59400=CARTESIAN_POINT('',(-0.460210453731243,0.00289211196316071,-0.6));
#59401=CARTESIAN_POINT('Ctrl Pts',(-0.460210453731243,0.00289211196316076,
-0.6));
#59402=CARTESIAN_POINT('Ctrl Pts',(-0.461043830945898,0.00144866028550932,
-0.599503641468838));
#59403=CARTESIAN_POINT('Ctrl Pts',(-0.4618802153517,9.15933995315753E-16,
-0.599));
#59404=CARTESIAN_POINT('Origin',(0.,0.,-0.6));
#59405=CARTESIAN_POINT('Origin',(-0.461880215351701,5.55111512312578E-17,
0.));
#59406=CARTESIAN_POINT('',(-0.23094010767585,0.4,0.));
#59407=CARTESIAN_POINT('',(-0.23094010767585,0.4,0.));
#59408=CARTESIAN_POINT('',(-0.461880215351701,5.6564012731995E-17,0.));
#59409=CARTESIAN_POINT('',(-0.404145188432738,0.1,0.));
#59410=CARTESIAN_POINT('',(-0.461880215351701,5.6564012731995E-17,0.));
#59411=CARTESIAN_POINT('Origin',(-0.461880215351701,5.55111512312578E-17,
0.));
#59412=CARTESIAN_POINT('',(-0.461880215351701,5.55111512312578E-17,-0.6));
#59413=CARTESIAN_POINT('',(-0.461880215351701,5.6564012731995E-17,0.));
#59414=CARTESIAN_POINT('',(-0.23094010767585,0.4,-0.6));
#59415=CARTESIAN_POINT('Origin',(-0.23094010767585,0.4,0.));
#59416=CARTESIAN_POINT('',(0.23094010767585,0.4,0.));
#59417=CARTESIAN_POINT('',(0.23094010767585,0.4,0.));
#59418=CARTESIAN_POINT('',(-0.115470053837925,0.4,0.));
#59419=CARTESIAN_POINT('Origin',(-0.23094010767585,0.4,0.));
#59420=CARTESIAN_POINT('',(0.23094010767585,0.4,-0.6));
#59421=CARTESIAN_POINT('',(0.23094010767585,0.4,-0.6));
#59422=CARTESIAN_POINT('',(0.23094010767585,0.4,0.));
#59423=CARTESIAN_POINT('Origin',(-0.23094010767585,0.4,0.));
#59424=CARTESIAN_POINT('',(-0.23094010767585,0.4,-0.6));
#59425=CARTESIAN_POINT('',(-0.23094010767585,0.4,0.));
#59426=CARTESIAN_POINT('',(0.23094010767585,0.4,-0.6));
#59427=CARTESIAN_POINT('Origin',(-0.230940107675851,-0.4,0.));
#59428=CARTESIAN_POINT('',(-0.230940107675851,-0.4,0.));
#59429=CARTESIAN_POINT('',(-0.288675134594813,-0.3,0.));
#59430=CARTESIAN_POINT('',(-0.230940107675851,-0.4,0.));
#59431=CARTESIAN_POINT('Origin',(-0.230940107675851,-0.4,0.));
#59432=CARTESIAN_POINT('',(-0.230940107675851,-0.4,-0.6));
#59433=CARTESIAN_POINT('',(-0.230940107675851,-0.4,0.));
#59434=CARTESIAN_POINT('',(-0.461880215351701,5.6564012731995E-17,-0.6));
#59435=CARTESIAN_POINT('Origin',(0.23094010767585,0.4,0.));
#59436=CARTESIAN_POINT('',(0.461880215351701,0.,0.));
#59437=CARTESIAN_POINT('',(0.461880215351701,0.,0.));
#59438=CARTESIAN_POINT('',(0.288675134594813,0.3,0.));
#59439=CARTESIAN_POINT('Origin',(0.23094010767585,0.4,0.));
#59440=CARTESIAN_POINT('',(0.461880215351701,0.,-0.6));
#59441=CARTESIAN_POINT('',(0.461880215351701,0.,-0.6));
#59442=CARTESIAN_POINT('',(0.461880215351701,0.,0.));
#59443=CARTESIAN_POINT('Origin',(0.23094010767585,0.4,0.));
#59444=CARTESIAN_POINT('',(0.461880215351701,0.,-0.6));
#59445=CARTESIAN_POINT('Origin',(0.,0.,-0.6));
#59446=CARTESIAN_POINT('',(-0.23094010767585,0.4,-0.6));
#59447=CARTESIAN_POINT('Origin',(0.,0.,-0.6));
#59448=CARTESIAN_POINT('Origin',(0.,0.,-0.6));
#59449=CARTESIAN_POINT('',(0.23094010767585,-0.4,-0.6));
#59450=CARTESIAN_POINT('Origin',(0.,0.,-0.6));
#59451=CARTESIAN_POINT('',(0.23094010767585,-0.4,-0.6));
#59452=CARTESIAN_POINT('',(-0.230940107675851,-0.4,-0.6));
#59453=CARTESIAN_POINT('',(0.23094010767585,-0.4,-0.6));
#59454=CARTESIAN_POINT('Origin',(0.,0.,-0.6));
#59455=CARTESIAN_POINT('',(-0.230940107675851,-0.4,-0.6));
#59456=CARTESIAN_POINT('Origin',(0.,0.,-0.6));
#59457=CARTESIAN_POINT('',(-0.461880215351701,5.6564012731995E-17,-0.6));
#59458=CARTESIAN_POINT('Origin',(0.461880215351701,0.,0.));
#59459=CARTESIAN_POINT('',(0.23094010767585,-0.4,0.));
#59460=CARTESIAN_POINT('',(0.23094010767585,-0.4,0.));
#59461=CARTESIAN_POINT('',(0.404145188432738,-0.1,0.));
#59462=CARTESIAN_POINT('Origin',(0.461880215351701,0.,0.));
#59463=CARTESIAN_POINT('',(0.23094010767585,-0.4,0.));
#59464=CARTESIAN_POINT('Origin',(0.461880215351701,0.,0.));
#59465=CARTESIAN_POINT('Origin',(0.23094010767585,-0.4,0.));
#59466=CARTESIAN_POINT('Origin',(0.23094010767585,-0.4,0.));
#59467=CARTESIAN_POINT('',(0.115470053837925,-0.4,0.));
#59468=CARTESIAN_POINT('Origin',(-0.461880215351701,5.55111512312578E-17,
0.));
#59469=CARTESIAN_POINT('Origin',(-0.230940107675851,-0.4,0.));
#59470=CARTESIAN_POINT('Origin',(0.23094010767585,-0.4,0.));
#59471=CARTESIAN_POINT('Origin',(0.6,0.,-4.));
#59472=CARTESIAN_POINT('',(-0.6,-7.34788079488412E-17,-4.));
#59473=CARTESIAN_POINT('Origin',(0.,0.,-4.));
#59474=CARTESIAN_POINT('Origin',(0.,0.,-3.9));
#59475=CARTESIAN_POINT('',(-0.7,-8.57252759403147E-17,-3.9));
#59476=CARTESIAN_POINT('Origin',(0.,0.,-1.94));
#59477=CARTESIAN_POINT('Origin',(0.,0.,-0.0711000000000002));
#59478=CARTESIAN_POINT('Origin',(0.,0.,-0.04));
#59479=CARTESIAN_POINT('',(-0.72,-8.81745695386094E-17,-6.93889390390723E-18));
#59480=CARTESIAN_POINT('Origin',(0.,0.,0.));
#59481=CARTESIAN_POINT('',(-0.76,-9.30731567351988E-17,-0.04));
#59482=CARTESIAN_POINT('Origin',(0.,0.,0.));
#70734=UNCERTAINTY_MEASURE_WITH_UNIT(LENGTH_MEASURE(0.001),#70758,
'DISTANCE_ACCURACY_VALUE',
'Maximum model space distance between geometric entities at asserted c
onnectivities');
#70740=UNCERTAINTY_MEASURE_WITH_UNIT(LENGTH_MEASURE(0.001),#70758,
'DISTANCE_ACCURACY_VALUE',
'Maximum model space distance between geometric entities at asserted c
onnectivities');
#70751=(
GEOMETRIC_REPRESENTATION_CONTEXT(3)
GLOBAL_UNCERTAINTY_ASSIGNED_CONTEXT((#70734))
GLOBAL_UNIT_ASSIGNED_CONTEXT((#70758,#70760,#70761))
REPRESENTATION_CONTEXT('','3D')
);
#70757=(
GEOMETRIC_REPRESENTATION_CONTEXT(3)
GLOBAL_UNCERTAINTY_ASSIGNED_CONTEXT((#70740))
GLOBAL_UNIT_ASSIGNED_CONTEXT((#70758,#70760,#70761))
REPRESENTATION_CONTEXT('','3D')
);
#70758=(
LENGTH_UNIT()
NAMED_UNIT(*)
SI_UNIT(.CENTI.,.METRE.)
);
#70760=(
NAMED_UNIT(*)
PLANE_ANGLE_UNIT()
SI_UNIT($,.RADIAN.)
);
#70761=(
NAMED_UNIT(*)
SI_UNIT($,.STERADIAN.)
SOLID_ANGLE_UNIT()
);
#70772=SHAPE_DEFINITION_REPRESENTATION(#70788,#70827);
#70788=PRODUCT_DEFINITION_SHAPE('',$,#70844);
#70827=SHAPE_REPRESENTATION('',(#27689),#70751);
#70833=PRODUCT_DEFINITION_CONTEXT('part definition',#70883,'design');
#70844=PRODUCT_DEFINITION('2026-10-19-02-56-03-690',
'14_ISO_4026_M16x40_Hub_Set_Screw',#70860,#70833);
#70860=PRODUCT_DEFINITION_FORMATION('',$,#70895);
#70883=APPLICATION_CONTEXT(
'Core Data for Automotive Mechanical Design Process');
#70884=PRODUCT_CONTEXT('part definition',#70883,'mechanical');
#70895=PRODUCT('2026-10-19-02-56-03-690',
'14_ISO_4026_M16x40_Hub_Set_Screw',$,(#70884));
#71048=COLOUR_RGB('Black',0.12,0.14,0.17);
#71049=FILL_AREA_STYLE_COLOUR('',#71048);
#71050=FILL_AREA_STYLE('',(#71049));
#71051=SURFACE_STYLE_FILL_AREA(#71050);
#71052=SURFACE_SIDE_STYLE('',(#71051));
#71053=SURFACE_STYLE_USAGE(.BOTH.,#71052);
#71054=PRESENTATION_STYLE_ASSIGNMENT((#71053));
ENDSEC;
END-ISO-10303-21;
